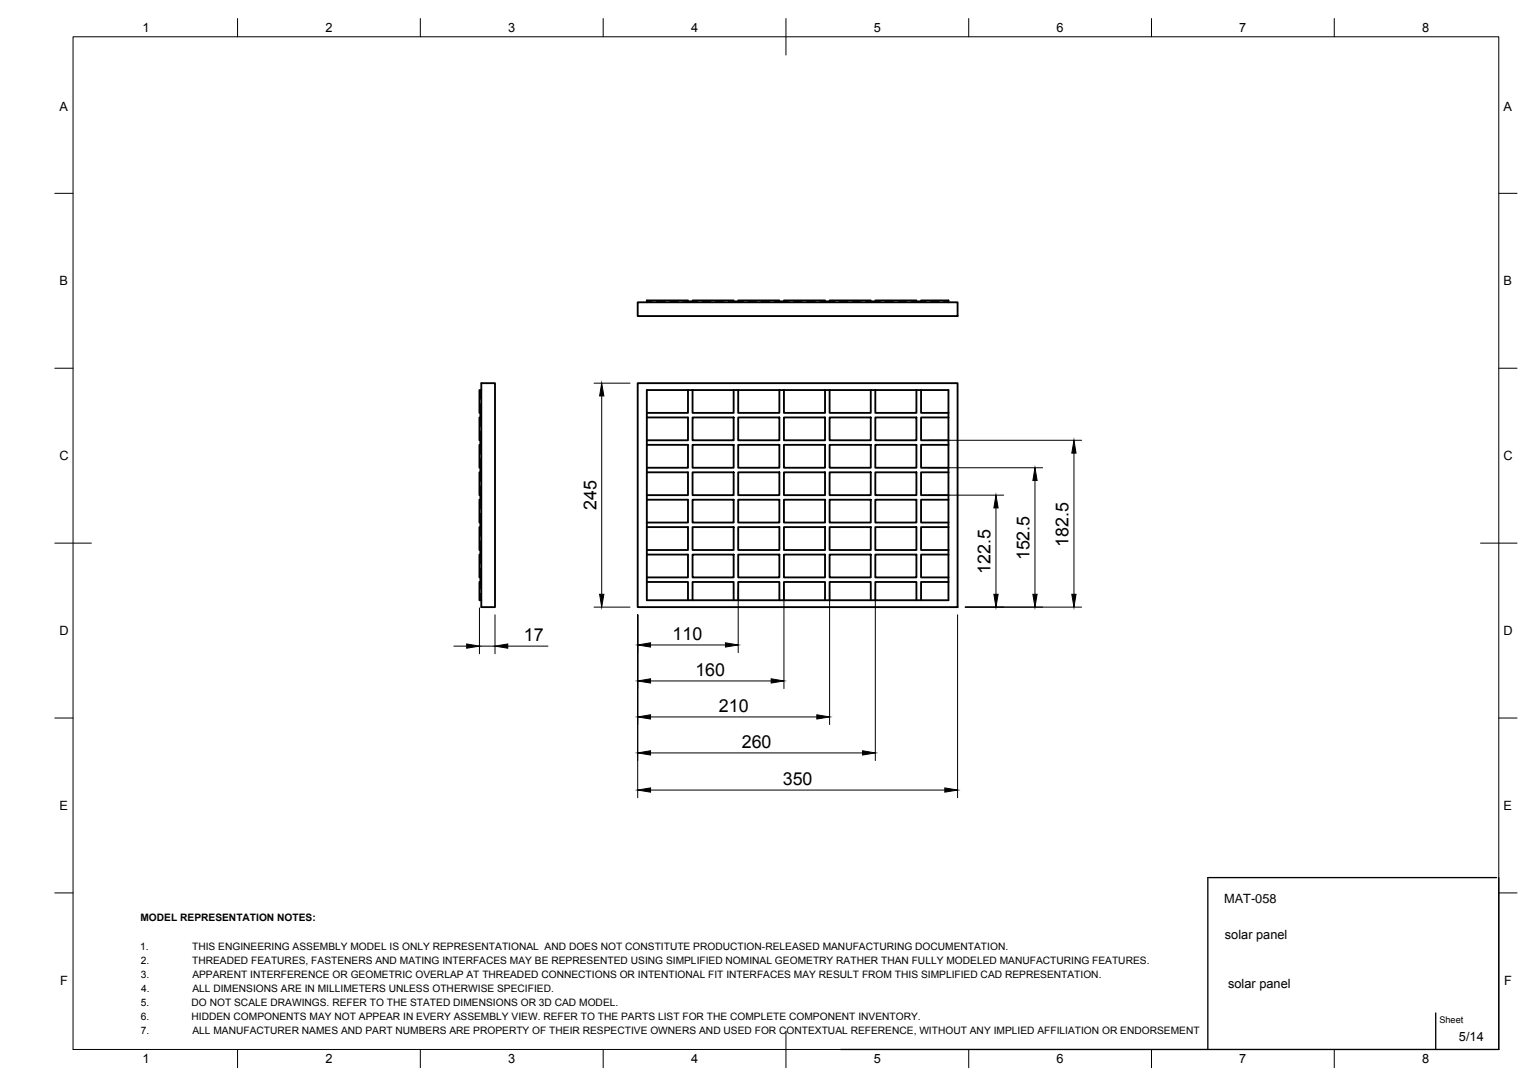
ISO-10303-21;
HEADER;
FILE_DESCRIPTION (('STEP AP214'),
    '1' );
FILE_NAME ('solar panel.step',
    '2026-10-21T17:54:40',
    ( '' ),
    ( '' ),
    'SwSTEP 2.0',
    'SolidWorks 2026',
    '' );
FILE_SCHEMA (( 'AUTOMOTIVE_DESIGN' ));
ENDSEC;

DATA;
#20=EDGE_CURVE ( 'NONE', #23493, #39659, #10554, .T. ) ;
#22=ORIENTED_EDGE ( 'NONE', *, *, #35505, .T. ) ;
#25=FACE_OUTER_BOUND ( 'NONE', #19071, .T. ) ;
#30=DIRECTION ( 'NONE',  ( 0.000000000000000000, 0.000000000000000000, 1.000000000000000000 ) ) ;
#34=AXIS2_PLACEMENT_3D ( 'NONE', #550, #47684, #4384 ) ;
#36=VERTEX_POINT ( 'NONE', #37038 ) ;
#46=ORIENTED_EDGE ( 'NONE', *, *, #39361, .F. ) ;
#51=CARTESIAN_POINT ( 'NONE',  ( -114.9999999999984652, 17.00000000000000000, 60.00000000000000000 ) ) ;
#57=LINE ( 'NONE', #42375, #32687 ) ;
#58=CARTESIAN_POINT ( 'NONE',  ( 130.0000000000021032, 17.00000000000000000, 95.00000000000000000 ) ) ;
#72=LINE ( 'NONE', #42385, #35392 ) ;
#73=EDGE_LOOP ( 'NONE', ( #24470, #20215, #48107, #6586 ) ) ;
#92=EDGE_CURVE ( 'NONE', #33627, #36736, #41611, .T. ) ;
#94=EDGE_CURVE ( 'NONE', #19596, #23363, #2597, .T. ) ;
#110=ORIENTED_EDGE ( 'NONE', *, *, #46921, .F. ) ;
#119=ORIENTED_EDGE ( 'NONE', *, *, #13290, .T. ) ;
#121=CARTESIAN_POINT ( 'NONE',  ( -114.9999999999978542, 17.00000000000000000, 95.00000000000000000 ) ) ;
#123=DIRECTION ( 'NONE',  ( -0.000000000000000000, -1.000000000000000000, -0.000000000000000000 ) ) ;
#125=CARTESIAN_POINT ( 'NONE',  ( -115.0000000000000284, 17.00000000000000000, -114.9999999999999858 ) ) ;
#133=ORIENTED_EDGE ( 'NONE', *, *, #48424, .F. ) ;
#137=FACE_OUTER_BOUND ( 'NONE', #38012, .T. ) ;
#140=VECTOR ( 'NONE', #20878, 1000.000000000000000 ) ;
#150=CARTESIAN_POINT ( 'NONE',  ( -14.99999999999876366, 17.00000000000000000, 30.00000000000000000 ) ) ;
#156=VERTEX_POINT ( 'NONE', #11065 ) ;
#162=LINE ( 'NONE', #15801, #49153 ) ;
#164=AXIS2_PLACEMENT_3D ( 'NONE', #11516, #32040, #11769 ) ;
#166=ORIENTED_EDGE ( 'NONE', *, *, #34974, .F. ) ;
#174=LINE ( 'NONE', #20666, #643 ) ;
#175=CARTESIAN_POINT ( 'NONE',  ( 30.00000000000062172, 17.00000000000000000, -54.99999999999999289 ) ) ;
#180=ADVANCED_FACE ( 'NONE', ( #12327 ), #40546, .F. ) ;
#186=ORIENTED_EDGE ( 'NONE', *, *, #38813, .T. ) ;
#193=EDGE_CURVE ( 'NONE', #28907, #37670, #20287, .T. ) ;
#196=VECTOR ( 'NONE', #29683, 1000.000000000000000 ) ;
#198=PLANE ( 'NONE',  #9790 ) ;
#221=ORIENTED_EDGE ( 'NONE', *, *, #30959, .F. ) ;
#224=ORIENTED_EDGE ( 'NONE', *, *, #7871, .F. ) ;
#230=PLANE ( 'NONE',  #20488 ) ;
#235=ADVANCED_FACE ( 'NONE', ( #32351 ), #40053, .F. ) ;
#243=DIRECTION ( 'NONE',  ( 1.000000000000000000, 0.000000000000000000, 0.000000000000000000 ) ) ;
#245=VECTOR ( 'NONE', #20305, 1000.000000000000000 ) ;
#246=EDGE_CURVE ( 'NONE', #20951, #20388, #31853, .T. ) ;
#251=DIRECTION ( 'NONE',  ( -1.000000000000000000, -0.000000000000000000, 9.251858538543084240E-16 ) ) ;
#264=EDGE_LOOP ( 'NONE', ( #43850, #6676, #18926, #28305 ) ) ;
#272=DIRECTION ( 'NONE',  ( 0.000000000000000000, 0.000000000000000000, 1.000000000000000000 ) ) ;
#277=VECTOR ( 'NONE', #22809, 1000.000000000000000 ) ;
#287=DIRECTION ( 'NONE',  ( -0.000000000000000000, -1.000000000000000000, -0.000000000000000000 ) ) ;
#302=VERTEX_POINT ( 'NONE', #41553 ) ;
#311=VECTOR ( 'NONE', #35432, 1000.000000000000000 ) ;
#313=EDGE_LOOP ( 'NONE', ( #26683, #2356, #8405, #20446 ) ) ;
#319=VECTOR ( 'NONE', #21069, 1000.000000000000000 ) ;
#321=ORIENTED_EDGE ( 'NONE', *, *, #26994, .T. ) ;
#325=VERTEX_POINT ( 'NONE', #9998 ) ;
#331=VECTOR ( 'NONE', #47511, 1000.000000000000000 ) ;
#338=EDGE_CURVE ( 'NONE', #17026, #45615, #13594, .T. ) ;
#343=VERTEX_POINT ( 'NONE', #22300 ) ;
#346=VECTOR ( 'NONE', #39780, 1000.000000000000000 ) ;
#364=FACE_OUTER_BOUND ( 'NONE', #38900, .T. ) ;
#375=VERTEX_POINT ( 'NONE', #32866 ) ;
#384=VECTOR ( 'NONE', #28524, 1000.000000000000000 ) ;
#389=DIRECTION ( 'NONE',  ( 0.000000000000000000, 0.000000000000000000, 1.000000000000000000 ) ) ;
#393=ORIENTED_EDGE ( 'NONE', *, *, #8336, .F. ) ;
#404=AXIS2_PLACEMENT_3D ( 'NONE', #20557, #28515, #1323 ) ;
#405=VERTEX_POINT ( 'NONE', #29501 ) ;
#409=DIRECTION ( 'NONE',  ( 1.000000000000000000, 0.000000000000000000, 0.000000000000000000 ) ) ;
#418=VERTEX_POINT ( 'NONE', #45117 ) ;
#437=ADVANCED_FACE ( 'NONE', ( #14088 ), #48694, .T. ) ;
#442=LINE ( 'NONE', #685, #41199 ) ;
#455=EDGE_LOOP ( 'NONE', ( #22398, #42737, #33219, #30241 ) ) ;
#465=ADVANCED_FACE ( 'NONE', ( #19658 ), #39933, .F. ) ;
#469=CARTESIAN_POINT ( 'NONE',  ( 135.0000000000015632, 17.00000000000000000, 35.00000000000000000 ) ) ;
#475=AXIS2_PLACEMENT_3D ( 'NONE', #19383, #34284, #35070 ) ;
#477=ORIENTED_EDGE ( 'NONE', *, *, #9884, .T. ) ;
#503=CARTESIAN_POINT ( 'NONE',  ( 35.00000000000186162, 17.00000000000000000, 90.00000000000000000 ) ) ;
#512=ORIENTED_EDGE ( 'NONE', *, *, #25092, .T. ) ;
#515=AXIS2_PLACEMENT_3D ( 'NONE', #26720, #30070, #30315 ) ;
#517=ORIENTED_EDGE ( 'NONE', *, *, #29930, .T. ) ;
#529=CARTESIAN_POINT ( 'NONE',  ( 130.0000000000008811, 17.00000000000000000, 0.000000000000000000 ) ) ;
#530=VECTOR ( 'NONE', #42052, 1000.000000000000000 ) ;
#540=CARTESIAN_POINT ( 'NONE',  ( 0.000000000000000000, 17.00000000000000000, 0.000000000000000000 ) ) ;
#550=CARTESIAN_POINT ( 'NONE',  ( -14.99999999999906919, 17.00000000000000000, 0.000000000000000000 ) ) ;
#553=ADVANCED_FACE ( 'NONE', ( #32726 ), #1435, .F. ) ;
#554=EDGE_LOOP ( 'NONE', ( #44360, #32925, #21521, #39510 ) ) ;
#562=FACE_OUTER_BOUND ( 'NONE', #36379, .T. ) ;
#570=FACE_OUTER_BOUND ( 'NONE', #16621, .T. ) ;
#572=VERTEX_POINT ( 'NONE', #13469 ) ;
#574=VERTEX_POINT ( 'NONE', #21414 ) ;
#593=VERTEX_POINT ( 'NONE', #47822 ) ;
#598=LINE ( 'NONE', #43663, #20030 ) ;
#608=ORIENTED_EDGE ( 'NONE', *, *, #26583, .T. ) ;
#614=VERTEX_POINT ( 'NONE', #44251 ) ;
#623=CARTESIAN_POINT ( 'NONE',  ( -19.99999999999971223, 16.00000000000000000, -84.99999999999998579 ) ) ;
#628=FACE_OUTER_BOUND ( 'NONE', #50651, .T. ) ;
#632=EDGE_LOOP ( 'NONE', ( #41784, #42230, #9108, #39526 ) ) ;
#643=VECTOR ( 'NONE', #47580, 1000.000000000000000 ) ;
#650=DIRECTION ( 'NONE',  ( -1.000000000000000000, 0.000000000000000000, -0.000000000000000000 ) ) ;
#651=ORIENTED_EDGE ( 'NONE', *, *, #30859, .F. ) ;
#654=ORIENTED_EDGE ( 'NONE', *, *, #31562, .T. ) ;
#659=ORIENTED_EDGE ( 'NONE', *, *, #38242, .F. ) ;
#674=CARTESIAN_POINT ( 'NONE',  ( -119.9999999999994174, 17.00000000000000000, -54.99999999999999289 ) ) ;
#680=CARTESIAN_POINT ( 'NONE',  ( 80.00000000000153477, 16.00000000000000000, 60.00000000000000000 ) ) ;
#681=CARTESIAN_POINT ( 'NONE',  ( 164.9999999999999716, 17.00000000000000000, -60.00000000000001421 ) ) ;
#685=CARTESIAN_POINT ( 'NONE',  ( 35.00000000000091660, 17.00000000000000000, -24.99999999999999289 ) ) ;
#690=LINE ( 'NONE', #30995, #5198 ) ;
#699=ORIENTED_EDGE ( 'NONE', *, *, #40875, .F. ) ;
#706=ORIENTED_EDGE ( 'NONE', *, *, #193, .T. ) ;
#709=CARTESIAN_POINT ( 'NONE',  ( -119.9999999999978400, 17.00000000000000000, 95.00000000000000000 ) ) ;
#717=FACE_OUTER_BOUND ( 'NONE', #38405, .T. ) ;
#726=EDGE_CURVE ( 'NONE', #3329, #34466, #14990, .T. ) ;
#732=CARTESIAN_POINT ( 'NONE',  ( -14.99999999999970868, 17.00000000000000000, -60.00000000000000000 ) ) ;
#740=EDGE_CURVE ( 'NONE', #30097, #19392, #10883, .T. ) ;
#752=VECTOR ( 'NONE', #24361, 1000.000000000000000 ) ;
#755=VECTOR ( 'NONE', #25642, 1000.000000000000000 ) ;
#766=EDGE_CURVE ( 'NONE', #31254, #1663, #37599, .T. ) ;
#768=ORIENTED_EDGE ( 'NONE', *, *, #15009, .T. ) ;
#774=ADVANCED_FACE ( 'NONE', ( #50080 ), #18072, .T. ) ;
#781=CARTESIAN_POINT ( 'NONE',  ( 135.0000000000021600, 16.00000000000000000, 95.00000000000000000 ) ) ;
#785=ORIENTED_EDGE ( 'NONE', *, *, #12346, .F. ) ;
#789=CARTESIAN_POINT ( 'NONE',  ( -19.99999999999940670, 17.00000000000000000, -30.00000000000000000 ) ) ;
#791=VECTOR ( 'NONE', #23137, 1000.000000000000000 ) ;
#794=EDGE_CURVE ( 'NONE', #35777, #38611, #10388, .T. ) ;
#798=VECTOR ( 'NONE', #15889, 1000.000000000000000 ) ;
#799=DIRECTION ( 'NONE',  ( 0.000000000000000000, -1.000000000000000000, 0.000000000000000000 ) ) ;
#802=EDGE_LOOP ( 'NONE', ( #19892, #43000, #16154, #21779 ) ) ;
#811=CARTESIAN_POINT ( 'NONE',  ( 35.00000000000186162, 16.00000000000000000, 65.00000000000000000 ) ) ;
#817=LINE ( 'NONE', #58, #1250 ) ;
#821=ORIENTED_EDGE ( 'NONE', *, *, #15184, .F. ) ;
#826=LINE ( 'NONE', #16475, #23214 ) ;
#839=CARTESIAN_POINT ( 'NONE',  ( 35.00000000000152767, 16.00000000000000000, 35.00000000000000000 ) ) ;
#844=CARTESIAN_POINT ( 'NONE',  ( -14.99999999999970868, 16.00000000000000000, -84.99999999999998579 ) ) ;
#845=VECTOR ( 'NONE', #3851, 1000.000000000000000 ) ;
#848=CARTESIAN_POINT ( 'NONE',  ( -164.9999999999990905, 17.00000000000000000, -24.99999999999999289 ) ) ;
#865=VERTEX_POINT ( 'NONE', #23456 ) ;
#867=AXIS2_PLACEMENT_3D ( 'NONE', #20688, #16848, #48346 ) ;
#871=LINE ( 'NONE', #16519, #9645 ) ;
#880=CARTESIAN_POINT ( 'NONE',  ( -19.99999999999815969, 16.00000000000000000, 65.00000000000000000 ) ) ;
#889=CARTESIAN_POINT ( 'NONE',  ( -64.99999999999940314, 17.00000000000000000, -54.99999999999999289 ) ) ;
#892=CARTESIAN_POINT ( 'NONE',  ( 85.00000000000184741, 17.00000000000000000, 65.00000000000000000 ) ) ;
#902=ORIENTED_EDGE ( 'NONE', *, *, #48896, .F. ) ;
#907=VERTEX_POINT ( 'NONE', #23706 ) ;
#908=ORIENTED_EDGE ( 'NONE', *, *, #17972, .T. ) ;
#919=LINE ( 'NONE', #40420, #42638 ) ;
#929=ORIENTED_EDGE ( 'NONE', *, *, #34476, .T. ) ;
#934=EDGE_CURVE ( 'NONE', #2472, #2811, #29066, .T. ) ;
#940=VECTOR ( 'NONE', #40898, 1000.000000000000000 ) ;
#941=ADVANCED_FACE ( 'NONE', ( #36028 ), #13159, .F. ) ;
#950=VERTEX_POINT ( 'NONE', #33187 ) ;
#970=VERTEX_POINT ( 'NONE', #24218 ) ;
#971=EDGE_CURVE ( 'NONE', #865, #3838, #17011, .T. ) ;
#978=ORIENTED_EDGE ( 'NONE', *, *, #12489, .T. ) ;
#981=LINE ( 'NONE', #28431, #46677 ) ;
#984=ORIENTED_EDGE ( 'NONE', *, *, #12101, .F. ) ;
#988=DIRECTION ( 'NONE',  ( 0.000000000000000000, 0.000000000000000000, -1.000000000000000000 ) ) ;
#997=CARTESIAN_POINT ( 'NONE',  ( -64.99999999999815259, 17.00000000000000000, 90.00000000000000000 ) ) ;
#1003=DIRECTION ( 'NONE',  ( -0.000000000000000000, -1.000000000000000000, -0.000000000000000000 ) ) ;
#1014=DIRECTION ( 'NONE',  ( 0.000000000000000000, 0.000000000000000000, -1.000000000000000000 ) ) ;
#1020=DIRECTION ( 'NONE',  ( -1.000000000000000000, -0.000000000000000000, -0.000000000000000000 ) ) ;
#1027=CARTESIAN_POINT ( 'NONE',  ( 85.00000000000056843, 17.00000000000000000, -30.00000000000000000 ) ) ;
#1034=EDGE_LOOP ( 'NONE', ( #26621, #37966, #49162, #17827 ) ) ;
#1035=CARTESIAN_POINT ( 'NONE',  ( -14.99999999999876366, 17.00000000000000000, 5.000000000000004441 ) ) ;
#1038=ORIENTED_EDGE ( 'NONE', *, *, #33245, .F. ) ;
#1046=DIRECTION ( 'NONE',  ( 0.000000000000000000, 0.000000000000000000, 1.000000000000000000 ) ) ;
#1057=DIRECTION ( 'NONE',  ( 0.000000000000000000, -0.000000000000000000, -1.000000000000000000 ) ) ;
#1067=ORIENTED_EDGE ( 'NONE', *, *, #11385, .F. ) ;
#1082=FACE_OUTER_BOUND ( 'NONE', #44486, .T. ) ;
#1090=EDGE_CURVE ( 'NONE', #32291, #24319, #41871, .T. ) ;
#1118=MECHANICAL_DESIGN_GEOMETRIC_PRESENTATION_REPRESENTATION('',(#6856),#35553);
#1147=VECTOR ( 'NONE', #17968, 1000.000000000000000 ) ;
#1148=EDGE_CURVE ( 'NONE', #30975, #45021, #10068, .T. ) ;
#1152=ORIENTED_EDGE ( 'NONE', *, *, #2044, .F. ) ;
#1162=PLANE ( 'NONE',  #7566 ) ;
#1174=VECTOR ( 'NONE', #42245, 1000.000000000000000 ) ;
#1181=ORIENTED_EDGE ( 'NONE', *, *, #33713, .F. ) ;
#1195=CARTESIAN_POINT ( 'NONE',  ( 35.00000000000122213, 17.00000000000000000, 5.000000000000004441 ) ) ;
#1202=DIRECTION ( 'NONE',  ( 0.000000000000000000, 0.000000000000000000, -1.000000000000000000 ) ) ;
#1204=AXIS2_PLACEMENT_3D ( 'NONE', #26739, #7748, #19015 ) ;
#1220=CARTESIAN_POINT ( 'NONE',  ( 35.00000000000091660, 16.00000000000000000, -24.99999999999999289 ) ) ;
#1236=EDGE_LOOP ( 'NONE', ( #22817, #30759, #48688, #4298 ) ) ;
#1245=LINE ( 'NONE', #9175, #17393 ) ;
#1247=FACE_OUTER_BOUND ( 'NONE', #4168, .T. ) ;
#1250=VECTOR ( 'NONE', #8517, 1000.000000000000000 ) ;
#1252=DIRECTION ( 'NONE',  ( -0.000000000000000000, -1.000000000000000000, -0.000000000000000000 ) ) ;
#1268=DIRECTION ( 'NONE',  ( 0.000000000000000000, 0.000000000000000000, 1.000000000000000000 ) ) ;
#1282=DIRECTION ( 'NONE',  ( -0.000000000000000000, -1.000000000000000000, -0.000000000000000000 ) ) ;
#1289=CARTESIAN_POINT ( 'NONE',  ( 80.00000000000061107, 17.00000000000000000, -54.99999999999999289 ) ) ;
#1292=EDGE_LOOP ( 'NONE', ( #10870, #27472, #30423, #39009 ) ) ;
#1293=ORIENTED_EDGE ( 'NONE', *, *, #18051, .F. ) ;
#1305=CARTESIAN_POINT ( 'NONE',  ( 30.00000000000123279, 17.00000000000000000, 5.000000000000004441 ) ) ;
#1319=DIRECTION ( 'NONE',  ( -1.000000000000000000, -0.000000000000000000, -0.000000000000000000 ) ) ;
#1323=DIRECTION ( 'NONE',  ( -1.000000000000000000, 0.000000000000000000, 2.312964634635843537E-16 ) ) ;
#1336=DIRECTION ( 'NONE',  ( -0.000000000000000000, -1.000000000000000000, -0.000000000000000000 ) ) ;
#1341=LINE ( 'NONE', #1837, #13601 ) ;
#1344=ORIENTED_EDGE ( 'NONE', *, *, #33713, .T. ) ;
#1348=CARTESIAN_POINT ( 'NONE',  ( -165.0000000000000284, 17.00000000000000000, -90.00000000000000000 ) ) ;
#1349=PLANE ( 'NONE',  #45547 ) ;
#1359=DIRECTION ( 'NONE',  ( 1.000000000000000000, 0.000000000000000000, 0.000000000000000000 ) ) ;
#1370=PLANE ( 'NONE',  #15035 ) ;
#1375=ORIENTED_EDGE ( 'NONE', *, *, #9884, .F. ) ;
#1384=DIRECTION ( 'NONE',  ( -0.000000000000000000, -0.000000000000000000, -1.000000000000000000 ) ) ;
#1386=ADVANCED_FACE ( 'NONE', ( #562 ), #28506, .F. ) ;
#1400=DIRECTION ( 'NONE',  ( 0.000000000000000000, 0.000000000000000000, 1.000000000000000000 ) ) ;
#1405=VERTEX_POINT ( 'NONE', #16688 ) ;
#1408=VECTOR ( 'NONE', #18293, 1000.000000000000000 ) ;
#1409=DIRECTION ( 'NONE',  ( 0.000000000000000000, 0.000000000000000000, 1.000000000000000000 ) ) ;
#1421=ORIENTED_EDGE ( 'NONE', *, *, #38820, .F. ) ;
#1424=AXIS2_PLACEMENT_3D ( 'NONE', #27930, #20227, #24090 ) ;
#1435=PLANE ( 'NONE',  #19680 ) ;
#1457=AXIS2_PLACEMENT_3D ( 'NONE', #19407, #34828, #31472 ) ;
#1471=DIRECTION ( 'NONE',  ( -2.312964634635864737E-16, 0.000000000000000000, -1.000000000000000000 ) ) ;
#1474=VERTEX_POINT ( 'NONE', #49462 ) ;
#1481=VERTEX_POINT ( 'NONE', #33623 ) ;
#1494=DIRECTION ( 'NONE',  ( 0.000000000000000000, 0.000000000000000000, 1.000000000000000000 ) ) ;
#1503=EDGE_CURVE ( 'NONE', #46696, #38550, #18450, .T. ) ;
#1526=LINE ( 'NONE', #32071, #45024 ) ;
#1528=VERTEX_POINT ( 'NONE', #48945 ) ;
#1535=ORIENTED_EDGE ( 'NONE', *, *, #37841, .F. ) ;
#1539=LINE ( 'NONE', #14076, #755 ) ;
#1549=CARTESIAN_POINT ( 'NONE',  ( 135.0000000000006253, 17.00000000000000000, -54.99999999999999289 ) ) ;
#1556=ORIENTED_EDGE ( 'NONE', *, *, #33956, .F. ) ;
#1578=ORIENTED_EDGE ( 'NONE', *, *, #38465, .F. ) ;
#1593=CARTESIAN_POINT ( 'NONE',  ( 135.0000000000015632, 17.00000000000000000, 35.00000000000000000 ) ) ;
#1597=CARTESIAN_POINT ( 'NONE',  ( -164.9999999999997442, 17.00000000000000000, -84.99999999999998579 ) ) ;
#1601=VECTOR ( 'NONE', #37906, 1000.000000000000000 ) ;
#1616=DIRECTION ( 'NONE',  ( 0.000000000000000000, 0.000000000000000000, 1.000000000000000000 ) ) ;
#1617=CARTESIAN_POINT ( 'NONE',  ( 129.9999999999999432, 17.00000000000000000, -114.9999999999999858 ) ) ;
#1626=DIRECTION ( 'NONE',  ( 1.000000000000000000, 0.000000000000000000, 0.000000000000000000 ) ) ;
#1628=LINE ( 'NONE', #17272, #16605 ) ;
#1653=CARTESIAN_POINT ( 'NONE',  ( 135.0000000000009663, 17.00000000000000000, -24.99999999999999289 ) ) ;
#1658=CARTESIAN_POINT ( 'NONE',  ( -64.99999999999815259, 16.00000000000000000, 90.00000000000000000 ) ) ;
#1663=VERTEX_POINT ( 'NONE', #31551 ) ;
#1669=VECTOR ( 'NONE', #37747, 1000.000000000000000 ) ;
#1683=CARTESIAN_POINT ( 'NONE',  ( -20.00000000000003197, 17.00000000000000000, -90.00000000000000000 ) ) ;
#1691=ADVANCED_FACE ( 'NONE', ( #22813 ), #15118, .F. ) ;
#1694=EDGE_CURVE ( 'NONE', #25157, #35762, #23369, .T. ) ;
#1697=ADVANCED_FACE ( 'NONE', ( #38733 ), #46388, .F. ) ;
#1701=DIRECTION ( 'NONE',  ( -0.000000000000000000, -1.000000000000000000, -0.000000000000000000 ) ) ;
#1707=AXIS2_PLACEMENT_3D ( 'NONE', #46684, #11062, #3101 ) ;
#1710=VECTOR ( 'NONE', #40010, 1000.000000000000000 ) ;
#1711=ORIENTED_EDGE ( 'NONE', *, *, #30976, .F. ) ;
#1718=ORIENTED_EDGE ( 'NONE', *, *, #38682, .T. ) ;
#1728=DIRECTION ( 'NONE',  ( 0.000000000000000000, 0.000000000000000000, 1.000000000000000000 ) ) ;
#1734=EDGE_CURVE ( 'NONE', #3452, #11387, #40498, .T. ) ;
#1743=VECTOR ( 'NONE', #7024, 1000.000000000000000 ) ;
#1751=CARTESIAN_POINT ( 'NONE',  ( 85.00000000000123634, 17.00000000000000000, 30.00000000000000000 ) ) ;
#1756=LINE ( 'NONE', #16389, #30760 ) ;
#1759=CARTESIAN_POINT ( 'NONE',  ( 135.0000000000009663, 16.00000000000000000, -24.99999999999999289 ) ) ;
#1770=EDGE_LOOP ( 'NONE', ( #6940, #12949, #39459, #6702 ) ) ;
#1775=EDGE_CURVE ( 'NONE', #28153, #21400, #32556, .T. ) ;
#1776=ORIENTED_EDGE ( 'NONE', *, *, #3846, .F. ) ;
#1778=CARTESIAN_POINT ( 'NONE',  ( 29.99999999999998579, 17.00000000000000000, -114.9999999999999858 ) ) ;
#1785=ORIENTED_EDGE ( 'NONE', *, *, #33974, .F. ) ;
#1788=ORIENTED_EDGE ( 'NONE', *, *, #23940, .F. ) ;
#1828=VECTOR ( 'NONE', #15724, 1000.000000000000000 ) ;
#1829=CARTESIAN_POINT ( 'NONE',  ( -114.9999999999991047, 16.00000000000000000, 0.000000000000000000 ) ) ;
#1834=DIRECTION ( 'NONE',  ( 0.000000000000000000, 0.000000000000000000, 1.000000000000000000 ) ) ;
#1837=CARTESIAN_POINT ( 'NONE',  ( -64.99999999999971578, 17.00000000000000000, -84.99999999999998579 ) ) ;
#1844=EDGE_CURVE ( 'NONE', #27666, #42474, #27940, .T. ) ;
#1866=DIRECTION ( 'NONE',  ( 1.000000000000000000, 0.000000000000000000, -0.000000000000000000 ) ) ;
#1867=FACE_OUTER_BOUND ( 'NONE', #40919, .T. ) ;
#1871=DIRECTION ( 'NONE',  ( 1.000000000000000000, 0.000000000000000000, 0.000000000000000000 ) ) ;
#1876=PLANE ( 'NONE',  #43014 ) ;
#1878=VERTEX_POINT ( 'NONE', #33812 ) ;
#1880=VECTOR ( 'NONE', #42551, 1000.000000000000000 ) ;
#1895=CARTESIAN_POINT ( 'NONE',  ( -114.9999999999994031, 17.00000000000000000, -30.00000000000000000 ) ) ;
#1900=ORIENTED_EDGE ( 'NONE', *, *, #7055, .T. ) ;
#1920=ORIENTED_EDGE ( 'NONE', *, *, #36078, .T. ) ;
#1929=ORIENTED_EDGE ( 'NONE', *, *, #31783, .F. ) ;
#1932=LINE ( 'NONE', #10389, #25219 ) ;
#1935=CARTESIAN_POINT ( 'NONE',  ( -64.99999999999877787, 16.00000000000000000, 5.000000000000004441 ) ) ;
#1936=EDGE_LOOP ( 'NONE', ( #15982, #1788, #659, #23682 ) ) ;
#1945=VECTOR ( 'NONE', #17455, 1000.000000000000000 ) ;
#1956=ORIENTED_EDGE ( 'NONE', *, *, #49060, .F. ) ;
#1964=DIRECTION ( 'NONE',  ( 1.000000000000000000, 0.000000000000000000, -2.312964634635864737E-16 ) ) ;
#1966=ORIENTED_EDGE ( 'NONE', *, *, #5485, .F. ) ;
#1968=CARTESIAN_POINT ( 'NONE',  ( 80.00000000000186162, 17.00000000000000000, 90.00000000000000000 ) ) ;
#1970=ORIENTED_EDGE ( 'NONE', *, *, #23753, .T. ) ;
#1972=AXIS2_PLACEMENT_3D ( 'NONE', #21850, #37515, #2333 ) ;
#1974=CARTESIAN_POINT ( 'NONE',  ( -114.9999999999997158, 17.00000000000000000, -60.00000000000000000 ) ) ;
#1976=EDGE_LOOP ( 'NONE', ( #15294, #42100, #49619, #25944 ) ) ;
#1983=EDGE_CURVE ( 'NONE', #7644, #20370, #41239, .T. ) ;
#1986=ADVANCED_FACE ( 'NONE', ( #25345 ), #40750, .F. ) ;
#2004=FACE_OUTER_BOUND ( 'NONE', #22418, .T. ) ;
#2005=EDGE_CURVE ( 'NONE', #47191, #2839, #26858, .T. ) ;
#2009=DIRECTION ( 'NONE',  ( 0.000000000000000000, 0.000000000000000000, 1.000000000000000000 ) ) ;
#2011=ORIENTED_EDGE ( 'NONE', *, *, #2047, .T. ) ;
#2014=CARTESIAN_POINT ( 'NONE',  ( -14.99999999999970868, 16.00000000000000000, -84.99999999999998579 ) ) ;
#2015=AXIS2_PLACEMENT_3D ( 'NONE', #44272, #17345, #9648 ) ;
#2023=CARTESIAN_POINT ( 'NONE',  ( -14.99999999999782041, 17.00000000000000000, 95.00000000000000000 ) ) ;
#2026=ORIENTED_EDGE ( 'NONE', *, *, #48076, .T. ) ;
#2041=ORIENTED_EDGE ( 'NONE', *, *, #38374, .F. ) ;
#2043=DIRECTION ( 'NONE',  ( -0.000000000000000000, -1.000000000000000000, -0.000000000000000000 ) ) ;
#2044=EDGE_CURVE ( 'NONE', #38025, #4851, #20418, .T. ) ;
#2047=EDGE_CURVE ( 'NONE', #35257, #35256, #8875, .T. ) ;
#2070=DIRECTION ( 'NONE',  ( 0.000000000000000000, 0.000000000000000000, -1.000000000000000000 ) ) ;
#2073=VECTOR ( 'NONE', #34325, 1000.000000000000000 ) ;
#2074=LINE ( 'NONE', #40570, #4337 ) ;
#2086=VERTEX_POINT ( 'NONE', #15819 ) ;
#2088=LINE ( 'NONE', #17475, #45768 ) ;
#2094=CARTESIAN_POINT ( 'NONE',  ( -19.99999999999878142, 16.00000000000000000, 5.000000000000004441 ) ) ;
#2096=ORIENTED_EDGE ( 'NONE', *, *, #29840, .F. ) ;
#2105=CARTESIAN_POINT ( 'NONE',  ( -19.99999999999783995, 17.00000000000000000, 95.00000000000000000 ) ) ;
#2108=CARTESIAN_POINT ( 'NONE',  ( 80.00000000000186162, 16.00000000000000000, 65.00000000000000000 ) ) ;
#2112=VECTOR ( 'NONE', #2639, 1000.000000000000000 ) ;
#2114=ORIENTED_EDGE ( 'NONE', *, *, #45262, .T. ) ;
#2118=EDGE_CURVE ( 'NONE', #35523, #46762, #44012, .T. ) ;
#2120=VECTOR ( 'NONE', #33876, 1000.000000000000000 ) ;
#2123=LINE ( 'NONE', #49009, #11921 ) ;
#2138=EDGE_CURVE ( 'NONE', #27259, #5809, #11372, .T. ) ;
#2139=VERTEX_POINT ( 'NONE', #50063 ) ;
#2156=ADVANCED_FACE ( 'NONE', ( #11635 ), #23175, .F. ) ;
#2172=FACE_OUTER_BOUND ( 'NONE', #36485, .T. ) ;
#2173=DIRECTION ( 'NONE',  ( -0.000000000000000000, -1.000000000000000000, -0.000000000000000000 ) ) ;
#2181=CARTESIAN_POINT ( 'NONE',  ( 135.0000000000021600, 16.00000000000000000, 115.0000000000000142 ) ) ;
#2183=ORIENTED_EDGE ( 'NONE', *, *, #7997, .F. ) ;
#2186=PLANE ( 'NONE',  #50543 ) ;
#2203=EDGE_CURVE ( 'NONE', #37192, #42338, #42157, .T. ) ;
#2210=DIRECTION ( 'NONE',  ( 0.000000000000000000, 0.000000000000000000, 1.000000000000000000 ) ) ;
#2212=VERTEX_POINT ( 'NONE', #27023 ) ;
#2256=EDGE_CURVE ( 'NONE', #44339, #18412, #42918, .T. ) ;
#2269=LINE ( 'NONE', #21775, #35286 ) ;
#2276=EDGE_CURVE ( 'NONE', #40766, #23064, #38342, .T. ) ;
#2277=PLANE ( 'NONE',  #41450 ) ;
#2278=ORIENTED_EDGE ( 'NONE', *, *, #5208, .F. ) ;
#2285=DIRECTION ( 'NONE',  ( -1.000000000000000000, -0.000000000000000000, -0.000000000000000000 ) ) ;
#2288=VERTEX_POINT ( 'NONE', #44899 ) ;
#2315=VECTOR ( 'NONE', #33438, 1000.000000000000000 ) ;
#2319=ORIENTED_EDGE ( 'NONE', *, *, #36924, .T. ) ;
#2324=VERTEX_POINT ( 'NONE', #13376 ) ;
#2329=DIRECTION ( 'NONE',  ( -0.000000000000000000, -0.000000000000000000, 1.000000000000000000 ) ) ;
#2330=LINE ( 'NONE', #17480, #1147 ) ;
#2333=DIRECTION ( 'NONE',  ( 0.000000000000000000, 0.000000000000000000, 1.000000000000000000 ) ) ;
#2335=ORIENTED_EDGE ( 'NONE', *, *, #44178, .F. ) ;
#2340=ADVANCED_FACE ( 'NONE', ( #45151 ), #6193, .F. ) ;
#2345=ORIENTED_EDGE ( 'NONE', *, *, #1694, .F. ) ;
#2348=PLANE ( 'NONE',  #18537 ) ;
#2356=ORIENTED_EDGE ( 'NONE', *, *, #31937, .F. ) ;
#2373=CARTESIAN_POINT ( 'NONE',  ( -114.9999999999981526, 17.00000000000000000, 65.00000000000000000 ) ) ;
#2374=ORIENTED_EDGE ( 'NONE', *, *, #30806, .F. ) ;
#2385=DIRECTION ( 'NONE',  ( 0.000000000000000000, 0.000000000000000000, 1.000000000000000000 ) ) ;
#2390=ORIENTED_EDGE ( 'NONE', *, *, #31295, .T. ) ;
#2404=LINE ( 'NONE', #6504, #16910 ) ;
#2405=CARTESIAN_POINT ( 'NONE',  ( 85.00000000000029843, 17.00000000000000000, -84.99999999999998579 ) ) ;
#2412=EDGE_CURVE ( 'NONE', #43496, #12984, #18225, .T. ) ;
#2415=ORIENTED_EDGE ( 'NONE', *, *, #42173, .F. ) ;
#2416=CARTESIAN_POINT ( 'NONE',  ( 85.00000000000029843, 16.00000000000000000, -84.99999999999998579 ) ) ;
#2417=LINE ( 'NONE', #37094, #7683 ) ;
#2422=VECTOR ( 'NONE', #2823, 1000.000000000000000 ) ;
#2425=PLANE ( 'NONE',  #10262 ) ;
#2428=EDGE_CURVE ( 'NONE', #26536, #46696, #22335, .T. ) ;
#2429=CARTESIAN_POINT ( 'NONE',  ( 35.00000000000216716, 16.00000000000000000, 115.0000000000000142 ) ) ;
#2443=VECTOR ( 'NONE', #28402, 1000.000000000000000 ) ;
#2444=LINE ( 'NONE', #29144, #11728 ) ;
#2450=LINE ( 'NONE', #29155, #45062 ) ;
#2452=CARTESIAN_POINT ( 'NONE',  ( -69.99999999999909051, 17.00000000000000000, 0.000000000000000000 ) ) ;
#2462=FACE_OUTER_BOUND ( 'NONE', #40549, .T. ) ;
#2472=VERTEX_POINT ( 'NONE', #37761 ) ;
#2483=EDGE_CURVE ( 'NONE', #43501, #26701, #32077, .T. ) ;
#2484=FACE_OUTER_BOUND ( 'NONE', #34875, .T. ) ;
#2500=ORIENTED_EDGE ( 'NONE', *, *, #41569, .F. ) ;
#2503=VECTOR ( 'NONE', #23758, 1000.000000000000000 ) ;
#2504=DIRECTION ( 'NONE',  ( -0.000000000000000000, -1.000000000000000000, -0.000000000000000000 ) ) ;
#2506=CARTESIAN_POINT ( 'NONE',  ( 164.9999999999999716, 17.00000000000000000, 59.99999999999999289 ) ) ;
#2507=VERTEX_POINT ( 'NONE', #24383 ) ;
#2513=CARTESIAN_POINT ( 'NONE',  ( -14.99999999999812594, 17.00000000000000000, 65.00000000000000000 ) ) ;
#2514=CARTESIAN_POINT ( 'NONE',  ( 34.99999999999997868, 17.00000000000000000, -90.00000000000000000 ) ) ;
#2516=LINE ( 'NONE', #17163, #37250 ) ;
#2517=ORIENTED_EDGE ( 'NONE', *, *, #44457, .F. ) ;
#2527=VERTEX_POINT ( 'NONE', #15916 ) ;
#2531=DIRECTION ( 'NONE',  ( -1.000000000000000000, -0.000000000000000000, -0.000000000000000000 ) ) ;
#2536=ORIENTED_EDGE ( 'NONE', *, *, #50341, .F. ) ;
#2544=FACE_BOUND ( 'NONE', #50410, .T. ) ;
#2547=CARTESIAN_POINT ( 'NONE',  ( -14.99999999999782041, 16.00000000000000000, 95.00000000000000000 ) ) ;
#2568=VECTOR ( 'NONE', #24294, 1000.000000000000000 ) ;
#2573=ORIENTED_EDGE ( 'NONE', *, *, #11718, .F. ) ;
#2575=CARTESIAN_POINT ( 'NONE',  ( 135.0000000000012790, 17.00000000000000000, 30.00000000000000000 ) ) ;
#2579=ORIENTED_EDGE ( 'NONE', *, *, #19259, .T. ) ;
#2580=EDGE_LOOP ( 'NONE', ( #21869, #13993, #23994, #18416 ) ) ;
#2582=ORIENTED_EDGE ( 'NONE', *, *, #14692, .T. ) ;
#2586=LINE ( 'NONE', #41347, #40139 ) ;
#2597=LINE ( 'NONE', #7737, #5617 ) ;
#2603=LINE ( 'NONE', #50203, #34893 ) ;
#2607=PLANE ( 'NONE',  #17875 ) ;
#2608=LINE ( 'NONE', #33933, #3718 ) ;
#2612=ORIENTED_EDGE ( 'NONE', *, *, #49052, .T. ) ;
#2636=CARTESIAN_POINT ( 'NONE',  ( -164.9999999999984936, 17.00000000000000000, 35.00000000000000000 ) ) ;
#2639=DIRECTION ( 'NONE',  ( 1.000000000000000000, 0.000000000000000000, 0.000000000000000000 ) ) ;
#2645=LINE ( 'NONE', #45212, #940 ) ;
#2663=FACE_OUTER_BOUND ( 'NONE', #13509, .T. ) ;
#2669=VECTOR ( 'NONE', #32314, 1000.000000000000000 ) ;
#2670=EDGE_CURVE ( 'NONE', #17128, #13622, #41268, .T. ) ;
#2675=LINE ( 'NONE', #33995, #41584 ) ;
#2677=VECTOR ( 'NONE', #42373, 1000.000000000000000 ) ;
#2689=DIRECTION ( 'NONE',  ( 0.000000000000000000, -1.000000000000000000, 0.000000000000000000 ) ) ;
#2691=ORIENTED_EDGE ( 'NONE', *, *, #7899, .F. ) ;
#2698=VECTOR ( 'NONE', #10503, 1000.000000000000000 ) ;
#2707=EDGE_LOOP ( 'NONE', ( #7508, #36482, #24854, #40175 ) ) ;
#2735=EDGE_LOOP ( 'NONE', ( #31824, #12828, #119, #35228 ) ) ;
#2747=VERTEX_POINT ( 'NONE', #25379 ) ;
#2753=CARTESIAN_POINT ( 'NONE',  ( -14.99999999999782041, 17.00000000000000000, 95.00000000000000000 ) ) ;
#2756=ADVANCED_FACE ( 'NONE', ( #39154 ), #45603, .F. ) ;
#2762=CARTESIAN_POINT ( 'NONE',  ( -19.99999999999846523, 17.00000000000000000, 60.00000000000000000 ) ) ;
#2768=VECTOR ( 'NONE', #30748, 1000.000000000000000 ) ;
#2791=CARTESIAN_POINT ( 'NONE',  ( -164.9999999999984936, 16.00000000000000000, 35.00000000000000000 ) ) ;
#2792=VECTOR ( 'NONE', #31544, 1000.000000000000000 ) ;
#2807=DIRECTION ( 'NONE',  ( 0.000000000000000000, -0.000000000000000000, -1.000000000000000000 ) ) ;
#2810=PLANE ( 'NONE',  #22180 ) ;
#2811=VERTEX_POINT ( 'NONE', #41527 ) ;
#2823=DIRECTION ( 'NONE',  ( -0.000000000000000000, -1.000000000000000000, -0.000000000000000000 ) ) ;
#2827=EDGE_CURVE ( 'NONE', #34035, #9083, #18668, .T. ) ;
#2833=LINE ( 'NONE', #11570, #18533 ) ;
#2839=VERTEX_POINT ( 'NONE', #10230 ) ;
#2848=EDGE_LOOP ( 'NONE', ( #12548, #50011, #24278, #41729 ) ) ;
#2849=EDGE_CURVE ( 'NONE', #36058, #16866, #34344, .T. ) ;
#2852=CARTESIAN_POINT ( 'NONE',  ( -114.9999999999994031, 17.00000000000000000, -54.99999999999999289 ) ) ;
#2853=DIRECTION ( 'NONE',  ( -1.000000000000000000, -0.000000000000000000, -0.000000000000000000 ) ) ;
#2868=ORIENTED_EDGE ( 'NONE', *, *, #35603, .F. ) ;
#2872=VECTOR ( 'NONE', #1252, 1000.000000000000000 ) ;
#2874=ORIENTED_EDGE ( 'NONE', *, *, #44978, .T. ) ;
#2877=LINE ( 'NONE', #14450, #7010 ) ;
#2884=ORIENTED_EDGE ( 'NONE', *, *, #5325, .T. ) ;
#2886=CARTESIAN_POINT ( 'NONE',  ( -64.99999999999877787, 17.00000000000000000, 30.00000000000000000 ) ) ;
#2908=EDGE_CURVE ( 'NONE', #22082, #37470, #14575, .T. ) ;
#2919=CARTESIAN_POINT ( 'NONE',  ( -14.99999999999845812, 17.00000000000000000, 35.00000000000000000 ) ) ;
#2934=ADVANCED_FACE ( 'NONE', ( #44477 ), #8850, .F. ) ;
#2941=DIRECTION ( 'NONE',  ( -1.000000000000000000, -0.000000000000000000, -0.000000000000000000 ) ) ;
#2951=AXIS2_PLACEMENT_3D ( 'NONE', #20075, #19309, #11624 ) ;
#2956=CARTESIAN_POINT ( 'NONE',  ( 85.00000000000090949, 17.00000000000000000, -24.99999999999999289 ) ) ;
#2959=ORIENTED_EDGE ( 'NONE', *, *, #42129, .T. ) ;
#2961=DIRECTION ( 'NONE',  ( -0.000000000000000000, -1.000000000000000000, -0.000000000000000000 ) ) ;
#2967=DIRECTION ( 'NONE',  ( -6.938893903907222461E-16, -0.000000000000000000, -1.000000000000000000 ) ) ;
#2976=ORIENTED_EDGE ( 'NONE', *, *, #28015, .T. ) ;
#2977=CARTESIAN_POINT ( 'NONE',  ( 0.000000000000000000, 17.00000000000000000, 0.000000000000000000 ) ) ;
#2978=CARTESIAN_POINT ( 'NONE',  ( -19.99999999999815969, 16.00000000000000000, 90.00000000000000000 ) ) ;
#2986=EDGE_LOOP ( 'NONE', ( #17759, #28658, #20389, #1956 ) ) ;
#2993=AXIS2_PLACEMENT_3D ( 'NONE', #43795, #24563, #24067 ) ;
#3004=EDGE_CURVE ( 'NONE', #20642, #23633, #49307, .T. ) ;
#3007=LINE ( 'NONE', #14304, #29645 ) ;
#3008=DIRECTION ( 'NONE',  ( 1.000000000000000000, 0.000000000000000000, -9.251858538543084240E-16 ) ) ;
#3009=LINE ( 'NONE', #18655, #2073 ) ;
#3010=ORIENTED_EDGE ( 'NONE', *, *, #11718, .T. ) ;
#3014=LINE ( 'NONE', #2762, #17264 ) ;
#3017=DIRECTION ( 'NONE',  ( -0.000000000000000000, -1.000000000000000000, -0.000000000000000000 ) ) ;
#3021=CARTESIAN_POINT ( 'NONE',  ( 135.0000000000003411, 17.00000000000000000, -84.99999999999998579 ) ) ;
#3040=CARTESIAN_POINT ( 'NONE',  ( -14.99999999999812594, 17.00000000000000000, 90.00000000000000000 ) ) ;
#3041=DIRECTION ( 'NONE',  ( 0.000000000000000000, -0.000000000000000000, -1.000000000000000000 ) ) ;
#3043=CARTESIAN_POINT ( 'NONE',  ( 35.00000000000122213, 17.00000000000000000, 30.00000000000000000 ) ) ;
#3044=CARTESIAN_POINT ( 'NONE',  ( -14.99999999999937472, 17.00000000000000000, -30.00000000000000000 ) ) ;
#3049=EDGE_CURVE ( 'NONE', #32394, #22969, #49558, .T. ) ;
#3052=EDGE_CURVE ( 'NONE', #43342, #34175, #49058, .T. ) ;
#3056=LINE ( 'NONE', #18700, #32288 ) ;
#3065=LINE ( 'NONE', #37994, #26446 ) ;
#3078=LINE ( 'NONE', #33899, #2422 ) ;
#3079=CARTESIAN_POINT ( 'NONE',  ( 80.00000000000028422, 17.00000000000000000, -60.00000000000000000 ) ) ;
#3086=VERTEX_POINT ( 'NONE', #29606 ) ;
#3093=EDGE_LOOP ( 'NONE', ( #8101, #18855, #13246, #36911 ) ) ;
#3096=DIRECTION ( 'NONE',  ( -1.000000000000000000, -0.000000000000000000, 4.625929269271635797E-16 ) ) ;
#3099=FACE_OUTER_BOUND ( 'NONE', #17848, .T. ) ;
#3101=DIRECTION ( 'NONE',  ( 0.000000000000000000, 0.000000000000000000, 1.000000000000000000 ) ) ;
#3102=CARTESIAN_POINT ( 'NONE',  ( -114.9999999999991047, 17.00000000000000000, -24.99999999999999289 ) ) ;
#3106=CARTESIAN_POINT ( 'NONE',  ( 30.00000000000187228, 17.00000000000000000, 65.00000000000000000 ) ) ;
#3115=AXIS2_PLACEMENT_3D ( 'NONE', #37666, #37173, #45809 ) ;
#3116=CARTESIAN_POINT ( 'NONE',  ( 35.00000000000028422, 17.00000000000000000, -84.99999999999998579 ) ) ;
#3118=CARTESIAN_POINT ( 'NONE',  ( -19.99999999999878142, 17.00000000000000000, 5.000000000000004441 ) ) ;
#3129=LINE ( 'NONE', #31107, #42142 ) ;
#3130=LINE ( 'NONE', #43162, #23045 ) ;
#3131=ORIENTED_EDGE ( 'NONE', *, *, #37323, .T. ) ;
#3138=ORIENTED_EDGE ( 'NONE', *, *, #22162, .F. ) ;
#3141=ADVANCED_FACE ( 'NONE', ( #21916 ), #37583, .F. ) ;
#3142=VECTOR ( 'NONE', #25991, 1000.000000000000000 ) ;
#3149=ORIENTED_EDGE ( 'NONE', *, *, #42550, .T. ) ;
#3154=LINE ( 'NONE', #18300, #28798 ) ;
#3159=CARTESIAN_POINT ( 'NONE',  ( 85.00000000000123634, 17.00000000000000000, 5.000000000000004441 ) ) ;
#3166=ORIENTED_EDGE ( 'NONE', *, *, #19090, .F. ) ;
#3175=DIRECTION ( 'NONE',  ( 1.000000000000000000, 0.000000000000000000, 0.000000000000000000 ) ) ;
#3176=CARTESIAN_POINT ( 'NONE',  ( -20.00000000000003197, 16.00000000000000000, -114.9999999999999858 ) ) ;
#3181=CARTESIAN_POINT ( 'NONE',  ( 135.0000000000006253, 16.00000000000000000, -54.99999999999999289 ) ) ;
#3182=VECTOR ( 'NONE', #6227, 1000.000000000000000 ) ;
#3183=PLANE ( 'NONE',  #12279 ) ;
#3194=EDGE_CURVE ( 'NONE', #17776, #34175, #42153, .T. ) ;
#3198=ORIENTED_EDGE ( 'NONE', *, *, #37933, .T. ) ;
#3202=CARTESIAN_POINT ( 'NONE',  ( -69.99999999999816680, 17.00000000000000000, 65.00000000000000000 ) ) ;
#3216=VERTEX_POINT ( 'NONE', #38337 ) ;
#3221=CARTESIAN_POINT ( 'NONE',  ( 35.00000000000061107, 16.00000000000000000, -30.00000000000000000 ) ) ;
#3229=CARTESIAN_POINT ( 'NONE',  ( -14.99999999999812594, 17.00000000000000000, 90.00000000000000000 ) ) ;
#3233=DIRECTION ( 'NONE',  ( 0.000000000000000000, -0.000000000000000000, -1.000000000000000000 ) ) ;
#3236=CARTESIAN_POINT ( 'NONE',  ( -64.99999999999971578, 16.00000000000000000, -60.00000000000000000 ) ) ;
#3250=VECTOR ( 'NONE', #31432, 1000.000000000000000 ) ;
#3256=VECTOR ( 'NONE', #17185, 1000.000000000000000 ) ;
#3258=VERTEX_POINT ( 'NONE', #26772 ) ;
#3275=ORIENTED_EDGE ( 'NONE', *, *, #12788, .F. ) ;
#3279=EDGE_LOOP ( 'NONE', ( #36139, #43467, #26596, #6835 ) ) ;
#3284=VERTEX_POINT ( 'NONE', #26515 ) ;
#3287=ORIENTED_EDGE ( 'NONE', *, *, #49621, .T. ) ;
#3297=EDGE_CURVE ( 'NONE', #20901, #15399, #36008, .T. ) ;
#3306=DIRECTION ( 'NONE',  ( -0.000000000000000000, -1.000000000000000000, -0.000000000000000000 ) ) ;
#3317=LINE ( 'NONE', #31048, #25609 ) ;
#3323=LINE ( 'NONE', #30801, #43763 ) ;
#3327=VECTOR ( 'NONE', #48289, 1000.000000000000000 ) ;
#3329=VERTEX_POINT ( 'NONE', #4930 ) ;
#3331=CARTESIAN_POINT ( 'NONE',  ( 30.00000000000092726, 17.00000000000000000, -24.99999999999999289 ) ) ;
#3339=AXIS2_PLACEMENT_3D ( 'NONE', #47286, #19860, #30933 ) ;
#3348=ORIENTED_EDGE ( 'NONE', *, *, #27379, .T. ) ;
#3349=DIRECTION ( 'NONE',  ( 0.000000000000000000, 0.000000000000000000, -1.000000000000000000 ) ) ;
#3355=LINE ( 'NONE', #41858, #30385 ) ;
#3361=ORIENTED_EDGE ( 'NONE', *, *, #20811, .T. ) ;
#3381=DIRECTION ( 'NONE',  ( -0.000000000000000000, -0.000000000000000000, -1.000000000000000000 ) ) ;
#3388=EDGE_CURVE ( 'NONE', #36127, #23493, #27543, .T. ) ;
#3389=DIRECTION ( 'NONE',  ( -1.000000000000000000, -0.000000000000000000, -0.000000000000000000 ) ) ;
#3395=VERTEX_POINT ( 'NONE', #23681 ) ;
#3404=VECTOR ( 'NONE', #1319, 1000.000000000000000 ) ;
#3409=DIRECTION ( 'NONE',  ( 0.000000000000000000, 0.000000000000000000, 1.000000000000000000 ) ) ;
#3412=DIRECTION ( 'NONE',  ( -0.000000000000000000, -0.000000000000000000, -1.000000000000000000 ) ) ;
#3413=AXIS2_PLACEMENT_3D ( 'NONE', #19158, #15338, #35105 ) ;
#3426=ORIENTED_EDGE ( 'NONE', *, *, #40442, .T. ) ;
#3438=VECTOR ( 'NONE', #42191, 1000.000000000000000 ) ;
#3442=LINE ( 'NONE', #3181, #34377 ) ;
#3452=VERTEX_POINT ( 'NONE', #25702 ) ;
#3453=CARTESIAN_POINT ( 'NONE',  ( -175.0000000000000000, 15.00000000000000000, 122.5000000000000142 ) ) ;
#3463=EDGE_CURVE ( 'NONE', #11684, #2139, #29297, .T. ) ;
#3465=ORIENTED_EDGE ( 'NONE', *, *, #7771, .T. ) ;
#3468=CARTESIAN_POINT ( 'NONE',  ( 85.00000000000152056, 17.00000000000000000, 35.00000000000000000 ) ) ;
#3474=ORIENTED_EDGE ( 'NONE', *, *, #22858, .F. ) ;
#3478=PLANE ( 'NONE',  #25794 ) ;
#3481=CARTESIAN_POINT ( 'NONE',  ( 129.9999999999999432, 16.00000000000000000, -90.00000000000000000 ) ) ;
#3487=VECTOR ( 'NONE', #47496, 1000.000000000000000 ) ;
#3499=ORIENTED_EDGE ( 'NONE', *, *, #25092, .F. ) ;
#3502=DIRECTION ( 'NONE',  ( 0.000000000000000000, 0.000000000000000000, 1.000000000000000000 ) ) ;
#3505=DIRECTION ( 'NONE',  ( -1.000000000000000000, 0.000000000000000000, -0.000000000000000000 ) ) ;
#3506=DIRECTION ( 'NONE',  ( -0.000000000000000000, -1.000000000000000000, -0.000000000000000000 ) ) ;
#3517=CARTESIAN_POINT ( 'NONE',  ( -65.00000000000002842, 17.00000000000000000, -114.9999999999999858 ) ) ;
#3529=CARTESIAN_POINT ( 'NONE',  ( 0.000000000000000000, 17.00000000000000000, 0.000000000000000000 ) ) ;
#3534=CARTESIAN_POINT ( 'NONE',  ( 85.00000000000213163, 17.00000000000000000, 115.0000000000000142 ) ) ;
#3550=CARTESIAN_POINT ( 'NONE',  ( -15.00000000000001421, 17.00000000000000000, -114.9999999999999858 ) ) ;
#3563=ORIENTED_EDGE ( 'NONE', *, *, #11111, .F. ) ;
#3569=DIRECTION ( 'NONE',  ( -0.000000000000000000, -1.000000000000000000, -0.000000000000000000 ) ) ;
#3576=DIRECTION ( 'NONE',  ( 0.000000000000000000, 0.000000000000000000, 1.000000000000000000 ) ) ;
#3599=CARTESIAN_POINT ( 'NONE',  ( 30.00000000000092726, 17.00000000000000000, 0.000000000000000000 ) ) ;
#3606=CARTESIAN_POINT ( 'NONE',  ( 85.00000000000090949, 17.00000000000000000, -24.99999999999999289 ) ) ;
#3607=EDGE_LOOP ( 'NONE', ( #34537, #18552, #35865, #36207 ) ) ;
#3610=CARTESIAN_POINT ( 'NONE',  ( 0.000000000000000000, 17.00000000000000000, 0.000000000000000000 ) ) ;
#3611=DIRECTION ( 'NONE',  ( 0.000000000000000000, 0.000000000000000000, 1.000000000000000000 ) ) ;
#3613=VECTOR ( 'NONE', #42083, 1000.000000000000000 ) ;
#3614=ORIENTED_EDGE ( 'NONE', *, *, #6119, .F. ) ;
#3616=EDGE_CURVE ( 'NONE', #39284, #48491, #15415, .T. ) ;
#3619=VECTOR ( 'NONE', #26495, 1000.000000000000000 ) ;
#3630=DIRECTION ( 'NONE',  ( -0.000000000000000000, -1.000000000000000000, -0.000000000000000000 ) ) ;
#3634=DIRECTION ( 'NONE',  ( 0.000000000000000000, 0.000000000000000000, 1.000000000000000000 ) ) ;
#3673=CARTESIAN_POINT ( 'NONE',  ( 130.0000000000021032, 16.00000000000000000, 95.00000000000000000 ) ) ;
#3674=ORIENTED_EDGE ( 'NONE', *, *, #36613, .T. ) ;
#3680=CARTESIAN_POINT ( 'NONE',  ( -65.00000000000002842, 16.00000000000000000, -90.00000000000000000 ) ) ;
#3683=CARTESIAN_POINT ( 'NONE',  ( -65.00000000000002842, 16.00000000000000000, -90.00000000000000000 ) ) ;
#3693=VECTOR ( 'NONE', #4074, 1000.000000000000000 ) ;
#3703=AXIS2_PLACEMENT_3D ( 'NONE', #32046, #36923, #37171 ) ;
#3705=ADVANCED_FACE ( 'NONE', ( #44107 ), #35442, .F. ) ;
#3709=LINE ( 'NONE', #27584, #4912 ) ;
#3711=CARTESIAN_POINT ( 'NONE',  ( 164.9999999999999716, 16.00000000000000000, 65.00000000000000000 ) ) ;
#3713=VECTOR ( 'NONE', #5926, 1000.000000000000000 ) ;
#3718=VECTOR ( 'NONE', #10070, 1000.000000000000000 ) ;
#3719=VERTEX_POINT ( 'NONE', #16670 ) ;
#3720=ORIENTED_EDGE ( 'NONE', *, *, #43078, .T. ) ;
#3730=AXIS2_PLACEMENT_3D ( 'NONE', #26082, #13766, #6585 ) ;
#3739=LINE ( 'NONE', #38651, #3861 ) ;
#3742=ORIENTED_EDGE ( 'NONE', *, *, #12633, .T. ) ;
#3746=CARTESIAN_POINT ( 'NONE',  ( -69.99999999999940314, 17.00000000000000000, -54.99999999999999289 ) ) ;
#3766=AXIS2_PLACEMENT_3D ( 'NONE', #45100, #37960, #14581 ) ;
#3772=DIRECTION ( 'NONE',  ( -0.000000000000000000, -1.000000000000000000, -0.000000000000000000 ) ) ;
#3780=CARTESIAN_POINT ( 'NONE',  ( 164.9999999999999716, 15.00000000000000000, 115.0000000000000142 ) ) ;
#3789=VERTEX_POINT ( 'NONE', #47934 ) ;
#3791=LINE ( 'NONE', #4307, #46173 ) ;
#3796=DIRECTION ( 'NONE',  ( 1.000000000000000000, 0.000000000000000000, 0.000000000000000000 ) ) ;
#3798=CARTESIAN_POINT ( 'NONE',  ( -69.99999999999940314, 16.00000000000000000, -30.00000000000000000 ) ) ;
#3803=VERTEX_POINT ( 'NONE', #35187 ) ;
#3806=ORIENTED_EDGE ( 'NONE', *, *, #8825, .F. ) ;
#3807=DIRECTION ( 'NONE',  ( -0.000000000000000000, -1.000000000000000000, -0.000000000000000000 ) ) ;
#3813=PLANE ( 'NONE',  #25568 ) ;
#3819=DIRECTION ( 'NONE',  ( 0.000000000000000000, 0.000000000000000000, -1.000000000000000000 ) ) ;
#3820=CARTESIAN_POINT ( 'NONE',  ( 35.00000000000216716, 17.00000000000000000, 115.0000000000000142 ) ) ;
#3838=VERTEX_POINT ( 'NONE', #20277 ) ;
#3841=EDGE_CURVE ( 'NONE', #7468, #41411, #35946, .T. ) ;
#3846=EDGE_CURVE ( 'NONE', #9471, #7228, #32084, .T. ) ;
#3847=AXIS2_PLACEMENT_3D ( 'NONE', #42030, #21520, #29478 ) ;
#3851=DIRECTION ( 'NONE',  ( -0.000000000000000000, -0.000000000000000000, -1.000000000000000000 ) ) ;
#3852=DIRECTION ( 'NONE',  ( -0.000000000000000000, -1.000000000000000000, -0.000000000000000000 ) ) ;
#3861=VECTOR ( 'NONE', #34813, 1000.000000000000000 ) ;
#3863=CARTESIAN_POINT ( 'NONE',  ( -165.0000000000000284, 16.00000000000000000, -114.9999999999999858 ) ) ;
#3867=EDGE_LOOP ( 'NONE', ( #9418, #36728, #42468, #12485 ) ) ;
#3884=FACE_OUTER_BOUND ( 'NONE', #39698, .T. ) ;
#3888=EDGE_CURVE ( 'NONE', #34035, #31951, #9225, .T. ) ;
#3914=EDGE_LOOP ( 'NONE', ( #27318, #30038, #31505, #40737 ) ) ;
#3916=EDGE_CURVE ( 'NONE', #9256, #30177, #1539, .T. ) ;
#3921=DIRECTION ( 'NONE',  ( 1.000000000000000000, 0.000000000000000000, 0.000000000000000000 ) ) ;
#3926=EDGE_CURVE ( 'NONE', #34772, #8207, #5879, .T. ) ;
#3927=ORIENTED_EDGE ( 'NONE', *, *, #35284, .T. ) ;
#3934=ORIENTED_EDGE ( 'NONE', *, *, #21121, .F. ) ;
#3936=CARTESIAN_POINT ( 'NONE',  ( -114.9999999999987779, 17.00000000000000000, 30.00000000000000000 ) ) ;
#3940=ORIENTED_EDGE ( 'NONE', *, *, #44807, .T. ) ;
#3943=ORIENTED_EDGE ( 'NONE', *, *, #12300, .F. ) ;
#3955=FACE_OUTER_BOUND ( 'NONE', #41248, .T. ) ;
#3964=AXIS2_PLACEMENT_3D ( 'NONE', #5219, #16771, #9076 ) ;
#3965=LINE ( 'NONE', #30155, #23785 ) ;
#3969=ORIENTED_EDGE ( 'NONE', *, *, #971, .F. ) ;
#3982=CARTESIAN_POINT ( 'NONE',  ( 35.00000000000091660, 16.00000000000000000, -24.99999999999999289 ) ) ;
#3984=ORIENTED_EDGE ( 'NONE', *, *, #46187, .T. ) ;
#3988=CARTESIAN_POINT ( 'NONE',  ( -69.99999999999972999, 17.00000000000000000, -60.00000000000000000 ) ) ;
#3998=LINE ( 'NONE', #42476, #48834 ) ;
#4019=VECTOR ( 'NONE', #18189, 1000.000000000000000 ) ;
#4023=ORIENTED_EDGE ( 'NONE', *, *, #7311, .T. ) ;
#4024=PLANE ( 'NONE',  #33528 ) ;
#4037=ORIENTED_EDGE ( 'NONE', *, *, #26822, .T. ) ;
#4044=EDGE_CURVE ( 'NONE', #49920, #14126, #34109, .T. ) ;
#4047=LINE ( 'NONE', #8159, #24117 ) ;
#4053=ADVANCED_FACE ( 'NONE', ( #25900 ), #26390, .F. ) ;
#4063=ORIENTED_EDGE ( 'NONE', *, *, #33730, .T. ) ;
#4064=DIRECTION ( 'NONE',  ( 1.000000000000000000, 0.000000000000000000, 0.000000000000000000 ) ) ;
#4069=DIRECTION ( 'NONE',  ( -1.000000000000000000, -0.000000000000000000, -0.000000000000000000 ) ) ;
#4074=DIRECTION ( 'NONE',  ( 1.000000000000000000, 0.000000000000000000, 0.000000000000000000 ) ) ;
#4077=FACE_OUTER_BOUND ( 'NONE', #33283, .T. ) ;
#4080=VECTOR ( 'NONE', #6104, 1000.000000000000000 ) ;
#4088=VECTOR ( 'NONE', #48245, 1000.000000000000000 ) ;
#4091=LINE ( 'NONE', #39506, #752 ) ;
#4092=CARTESIAN_POINT ( 'NONE',  ( -114.9999999999984652, 17.00000000000000000, 35.00000000000000000 ) ) ;
#4093=CARTESIAN_POINT ( 'NONE',  ( -164.9999999999997442, 17.00000000000000000, -60.00000000000000000 ) ) ;
#4095=VECTOR ( 'NONE', #23354, 1000.000000000000000 ) ;
#4098=ORIENTED_EDGE ( 'NONE', *, *, #11415, .F. ) ;
#4101=FACE_OUTER_BOUND ( 'NONE', #10309, .T. ) ;
#4105=ORIENTED_EDGE ( 'NONE', *, *, #28088, .T. ) ;
#4107=CARTESIAN_POINT ( 'NONE',  ( 29.99999999999998579, 17.00000000000000000, -90.00000000000000000 ) ) ;
#4114=CARTESIAN_POINT ( 'NONE',  ( -165.0000000000000284, 16.00000000000000000, 115.0000000000000142 ) ) ;
#4130=CARTESIAN_POINT ( 'NONE',  ( 135.0000000000003411, 16.00000000000000000, -60.00000000000000000 ) ) ;
#4140=PLANE ( 'NONE',  #24805 ) ;
#4142=EDGE_LOOP ( 'NONE', ( #9671, #14688, #699, #4511 ) ) ;
#4146=PLANE ( 'NONE',  #39828 ) ;
#4164=AXIS2_PLACEMENT_3D ( 'NONE', #38541, #22611, #3611 ) ;
#4165=VECTOR ( 'NONE', #10960, 1000.000000000000000 ) ;
#4167=CARTESIAN_POINT ( 'NONE',  ( 135.0000000000012790, 17.00000000000000000, 5.000000000000004441 ) ) ;
#4168=EDGE_LOOP ( 'NONE', ( #34605, #11609, #27626, #32368 ) ) ;
#4173=DIRECTION ( 'NONE',  ( 0.000000000000000000, -1.000000000000000000, 0.000000000000000000 ) ) ;
#4183=DIRECTION ( 'NONE',  ( 0.000000000000000000, 0.000000000000000000, 1.000000000000000000 ) ) ;
#4187=ORIENTED_EDGE ( 'NONE', *, *, #21739, .T. ) ;
#4191=VECTOR ( 'NONE', #46469, 1000.000000000000000 ) ;
#4197=CARTESIAN_POINT ( 'NONE',  ( -114.9999999999994031, 17.00000000000000000, -30.00000000000000000 ) ) ;
#4198=PLANE ( 'NONE',  #5409 ) ;
#4199=VECTOR ( 'NONE', #7271, 1000.000000000000000 ) ;
#4202=PRODUCT_DEFINITION_CONTEXT ( 'detailed design', #39776, 'design' ) ;
#4205=VECTOR ( 'NONE', #1202, 1000.000000000000000 ) ;
#4207=CARTESIAN_POINT ( 'NONE',  ( 35.00000000000152767, 16.00000000000000000, 35.00000000000000000 ) ) ;
#4208=EDGE_LOOP ( 'NONE', ( #18998, #37444, #48111, #24651 ) ) ;
#4218=DIRECTION ( 'NONE',  ( 0.000000000000000000, -0.000000000000000000, -1.000000000000000000 ) ) ;
#4222=EDGE_CURVE ( 'NONE', #593, #23700, #23817, .T. ) ;
#4224=DIRECTION ( 'NONE',  ( -0.000000000000000000, -1.000000000000000000, -0.000000000000000000 ) ) ;
#4235=CARTESIAN_POINT ( 'NONE',  ( 35.00000000000216716, 16.00000000000000000, 95.00000000000000000 ) ) ;
#4255=DIRECTION ( 'NONE',  ( -0.000000000000000000, -1.000000000000000000, -0.000000000000000000 ) ) ;
#4262=ORIENTED_EDGE ( 'NONE', *, *, #19250, .F. ) ;
#4263=VERTEX_POINT ( 'NONE', #1974 ) ;
#4265=CARTESIAN_POINT ( 'NONE',  ( -69.99999999999940314, 17.00000000000000000, -30.00000000000000000 ) ) ;
#4270=CARTESIAN_POINT ( 'NONE',  ( -164.9999999999997442, 17.00000000000000000, -60.00000000000000000 ) ) ;
#4298=ORIENTED_EDGE ( 'NONE', *, *, #23675, .T. ) ;
#4305=VECTOR ( 'NONE', #10915, 1000.000000000000000 ) ;
#4307=CARTESIAN_POINT ( 'NONE',  ( -64.99999999999877787, 17.00000000000000000, 5.000000000000004441 ) ) ;
#4309=DIRECTION ( 'NONE',  ( 0.000000000000000000, 0.000000000000000000, 1.000000000000000000 ) ) ;
#4317=CARTESIAN_POINT ( 'NONE',  ( -64.99999999999846523, 16.00000000000000000, 35.00000000000000000 ) ) ;
#4326=PLANE ( 'NONE',  #4920 ) ;
#4335=LINE ( 'NONE', #3820, #11721 ) ;
#4337=VECTOR ( 'NONE', #17722, 1000.000000000000000 ) ;
#4340=EDGE_CURVE ( 'NONE', #39670, #46399, #48119, .T. ) ;
#4345=DIRECTION ( 'NONE',  ( 1.000000000000000000, 0.000000000000000000, 0.000000000000000000 ) ) ;
#4352=VERTEX_POINT ( 'NONE', #18364 ) ;
#4356=EDGE_LOOP ( 'NONE', ( #33297, #34547, #24964, #35461 ) ) ;
#4377=CARTESIAN_POINT ( 'NONE',  ( -15.00000000000001421, 17.00000000000000000, -90.00000000000000000 ) ) ;
#4378=CARTESIAN_POINT ( 'NONE',  ( -64.99999999999846523, 16.00000000000000000, 35.00000000000000000 ) ) ;
#4381=EDGE_CURVE ( 'NONE', #37527, #20642, #38155, .T. ) ;
#4383=CARTESIAN_POINT ( 'NONE',  ( -165.0000000000000284, 16.00000000000000000, 115.0000000000000142 ) ) ;
#4384=DIRECTION ( 'NONE',  ( -1.000000000000000000, 0.000000000000000000, -0.000000000000000000 ) ) ;
#4389=DIRECTION ( 'NONE',  ( 4.625929269271635797E-16, -0.000000000000000000, 1.000000000000000000 ) ) ;
#4391=ORIENTED_EDGE ( 'NONE', *, *, #6692, .F. ) ;
#4392=VERTEX_POINT ( 'NONE', #34546 ) ;
#4400=DIRECTION ( 'NONE',  ( -0.000000000000000000, -0.000000000000000000, -1.000000000000000000 ) ) ;
#4402=PLANE ( 'NONE',  #40097 ) ;
#4407=ORIENTED_EDGE ( 'NONE', *, *, #29641, .T. ) ;
#4409=ORIENTED_EDGE ( 'NONE', *, *, #3297, .F. ) ;
#4410=CARTESIAN_POINT ( 'NONE',  ( -19.99999999999908695, 17.00000000000000000, 0.000000000000000000 ) ) ;
#4437=ORIENTED_EDGE ( 'NONE', *, *, #27623, .T. ) ;
#4439=EDGE_CURVE ( 'NONE', #17801, #46696, #11200, .T. ) ;
#4447=LINE ( 'NONE', #35513, #5019 ) ;
#4451=ORIENTED_EDGE ( 'NONE', *, *, #45572, .F. ) ;
#4454=ORIENTED_EDGE ( 'NONE', *, *, #16913, .F. ) ;
#4472=VECTOR ( 'NONE', #46300, 1000.000000000000000 ) ;
#4484=EDGE_CURVE ( 'NONE', #17776, #17128, #20147, .T. ) ;
#4493=ORIENTED_EDGE ( 'NONE', *, *, #41816, .F. ) ;
#4494=VECTOR ( 'NONE', #21822, 1000.000000000000000 ) ;
#4509=EDGE_CURVE ( 'NONE', #28907, #572, #16058, .T. ) ;
#4511=ORIENTED_EDGE ( 'NONE', *, *, #21469, .T. ) ;
#4520=ORIENTED_EDGE ( 'NONE', *, *, #46000, .T. ) ;
#4523=DIRECTION ( 'NONE',  ( -3.469446951953611724E-16, 0.000000000000000000, 1.000000000000000000 ) ) ;
#4527=EDGE_CURVE ( 'NONE', #32976, #22529, #35573, .T. ) ;
#4536=AXIS2_PLACEMENT_3D ( 'NONE', #32172, #24726, #32670 ) ;
#4538=VECTOR ( 'NONE', #36400, 1000.000000000000000 ) ;
#4539=ORIENTED_EDGE ( 'NONE', *, *, #3004, .F. ) ;
#4543=ORIENTED_EDGE ( 'NONE', *, *, #47512, .T. ) ;
#4555=PLANE ( 'NONE',  #2993 ) ;
#4567=VECTOR ( 'NONE', #44736, 1000.000000000000000 ) ;
#4568=ORIENTED_EDGE ( 'NONE', *, *, #49970, .T. ) ;
#4578=CARTESIAN_POINT ( 'NONE',  ( -164.9999999999997442, 17.00000000000000000, -84.99999999999998579 ) ) ;
#4579=VECTOR ( 'NONE', #19946, 1000.000000000000000 ) ;
#4580=LINE ( 'NONE', #44545, #21892 ) ;
#4585=DIRECTION ( 'NONE',  ( -1.000000000000000000, 0.000000000000000000, 0.000000000000000000 ) ) ;
#4590=AXIS2_PLACEMENT_3D ( 'NONE', #1653, #32698, #25004 ) ;
#4591=CARTESIAN_POINT ( 'NONE',  ( -65.00000000000002842, 16.00000000000000000, -114.9999999999999858 ) ) ;
#4593=EDGE_CURVE ( 'NONE', #45598, #5571, #919, .T. ) ;
#4594=PLANE ( 'NONE',  #28179 ) ;
#4599=CARTESIAN_POINT ( 'NONE',  ( -19.99999999999878142, 17.00000000000000000, 5.000000000000004441 ) ) ;
#4604=CARTESIAN_POINT ( 'NONE',  ( -64.99999999999815259, 17.00000000000000000, 65.00000000000000000 ) ) ;
#4612=CARTESIAN_POINT ( 'NONE',  ( 135.0000000000006253, 17.00000000000000000, -30.00000000000000000 ) ) ;
#4634=LINE ( 'NONE', #16672, #3256 ) ;
#4644=VECTOR ( 'NONE', #42594, 1000.000000000000000 ) ;
#4649=ADVANCED_FACE ( 'NONE', ( #20653 ), #38293, .F. ) ;
#4657=CARTESIAN_POINT ( 'NONE',  ( -19.99999999999846523, 16.00000000000000000, 35.00000000000000000 ) ) ;
#4660=DIRECTION ( 'NONE',  ( 1.000000000000000000, 0.000000000000000000, -2.312964634635864737E-16 ) ) ;
#4664=VECTOR ( 'NONE', #27657, 1000.000000000000000 ) ;
#4668=CARTESIAN_POINT ( 'NONE',  ( -164.9999999999994031, 17.00000000000000000, -54.99999999999999289 ) ) ;
#4672=LINE ( 'NONE', #44397, #46955 ) ;
#4680=FACE_OUTER_BOUND ( 'NONE', #45680, .T. ) ;
#4684=EDGE_LOOP ( 'NONE', ( #47062, #20099, #110, #37219 ) ) ;
#4685=ORIENTED_EDGE ( 'NONE', *, *, #23613, .F. ) ;
#4689=ADVANCED_FACE ( 'NONE', ( #50517 ), #35196, .F. ) ;
#4691=DIRECTION ( 'NONE',  ( 0.000000000000000000, 0.000000000000000000, 1.000000000000000000 ) ) ;
#4700=ORIENTED_EDGE ( 'NONE', *, *, #14862, .T. ) ;
#4702=ORIENTED_EDGE ( 'NONE', *, *, #12383, .F. ) ;
#4710=LINE ( 'NONE', #47262, #25030 ) ;
#4712=( LENGTH_UNIT ( ) NAMED_UNIT ( * ) SI_UNIT ( .MILLI., .METRE. ) );
#4717=CARTESIAN_POINT ( 'NONE',  ( -114.9999999999991047, 16.00000000000000000, -24.99999999999999289 ) ) ;
#4720=ORIENTED_EDGE ( 'NONE', *, *, #6786, .T. ) ;
#4722=DIRECTION ( 'NONE',  ( 1.000000000000000000, 0.000000000000000000, 0.000000000000000000 ) ) ;
#4725=ORIENTED_EDGE ( 'NONE', *, *, #23850, .F. ) ;
#4728=EDGE_CURVE ( 'NONE', #38804, #36506, #3355, .T. ) ;
#4731=LINE ( 'NONE', #3780, #32041 ) ;
#4736=CARTESIAN_POINT ( 'NONE',  ( 80.00000000000028422, 17.00000000000000000, -84.99999999999998579 ) ) ;
#4760=PLANE ( 'NONE',  #16783 ) ;
#4762=VERTEX_POINT ( 'NONE', #34431 ) ;
#4763=DIRECTION ( 'NONE',  ( -1.000000000000000000, 0.000000000000000000, 0.000000000000000000 ) ) ;
#4785=ORIENTED_EDGE ( 'NONE', *, *, #43874, .T. ) ;
#4791=FACE_OUTER_BOUND ( 'NONE', #13855, .T. ) ;
#4793=DIRECTION ( 'NONE',  ( -0.000000000000000000, -1.000000000000000000, -0.000000000000000000 ) ) ;
#4794=LINE ( 'NONE', #469, #21733 ) ;
#4798=ADVANCED_FACE ( 'NONE', ( #26460 ), #26966, .F. ) ;
#4820=LINE ( 'NONE', #35667, #18329 ) ;
#4821=ORIENTED_EDGE ( 'NONE', *, *, #32289, .T. ) ;
#4843=ORIENTED_EDGE ( 'NONE', *, *, #7323, .T. ) ;
#4851=VERTEX_POINT ( 'NONE', #39288 ) ;
#4852=CARTESIAN_POINT ( 'NONE',  ( -114.9999999999997158, 17.00000000000000000, -84.99999999999998579 ) ) ;
#4856=EDGE_CURVE ( 'NONE', #39319, #34689, #36203, .T. ) ;
#4858=FACE_OUTER_BOUND ( 'NONE', #14635, .T. ) ;
#4859=ADVANCED_FACE ( 'NONE', ( #24149 ), #16437, .F. ) ;
#4861=ADVANCED_FACE ( 'NONE', ( #16949 ), #28492, .F. ) ;
#4876=CARTESIAN_POINT ( 'NONE',  ( 79.99999999999997158, 17.00000000000000000, -114.9999999999999858 ) ) ;
#4882=ORIENTED_EDGE ( 'NONE', *, *, #33394, .F. ) ;
#4903=PLANE ( 'NONE',  #10984 ) ;
#4912=VECTOR ( 'NONE', #47284, 1000.000000000000000 ) ;
#4913=FACE_OUTER_BOUND ( 'NONE', #21349, .T. ) ;
#4917=CARTESIAN_POINT ( 'NONE',  ( -119.9999999999987921, 17.00000000000000000, 30.00000000000000000 ) ) ;
#4920=AXIS2_PLACEMENT_3D ( 'NONE', #47373, #47125, #24346 ) ;
#4921=EDGE_CURVE ( 'NONE', #23363, #45598, #36726, .T. ) ;
#4923=ORIENTED_EDGE ( 'NONE', *, *, #11591, .F. ) ;
#4927=EDGE_CURVE ( 'NONE', #27084, #43076, #48440, .T. ) ;
#4928=LINE ( 'NONE', #12880, #43793 ) ;
#4930=CARTESIAN_POINT ( 'NONE',  ( 85.00000000000056843, 16.00000000000000000, -30.00000000000000000 ) ) ;
#4931=ORIENTED_EDGE ( 'NONE', *, *, #37246, .F. ) ;
#4936=LINE ( 'NONE', #31401, #27188 ) ;
#4942=FACE_OUTER_BOUND ( 'NONE', #33154, .T. ) ;
#4953=VECTOR ( 'NONE', #50294, 1000.000000000000000 ) ;
#4962=FACE_OUTER_BOUND ( 'NONE', #22538, .T. ) ;
#4970=ORIENTED_EDGE ( 'NONE', *, *, #13329, .T. ) ;
#4974=EDGE_CURVE ( 'NONE', #45538, #29858, #6146, .T. ) ;
#4987=VECTOR ( 'NONE', #33155, 1000.000000000000000 ) ;
#5006=ORIENTED_EDGE ( 'NONE', *, *, #39938, .T. ) ;
#5011=ORIENTED_EDGE ( 'NONE', *, *, #7749, .T. ) ;
#5019=VECTOR ( 'NONE', #19580, 1000.000000000000000 ) ;
#5025=CARTESIAN_POINT ( 'NONE',  ( -114.9999999999981526, 17.00000000000000000, 65.00000000000000000 ) ) ;
#5042=FACE_OUTER_BOUND ( 'NONE', #24888, .T. ) ;
#5044=ORIENTED_EDGE ( 'NONE', *, *, #40567, .T. ) ;
#5046=AXIS2_PLACEMENT_3D ( 'NONE', #10177, #29932, #10676 ) ;
#5048=EDGE_LOOP ( 'NONE', ( #40796, #18660, #49133, #47207 ) ) ;
#5050=DIRECTION ( 'NONE',  ( 0.000000000000000000, 0.000000000000000000, 1.000000000000000000 ) ) ;
#5056=ORIENTED_EDGE ( 'NONE', *, *, #34066, .F. ) ;
#5070=CARTESIAN_POINT ( 'NONE',  ( -165.0000000000000284, 16.00000000000000000, -60.00000000000000000 ) ) ;
#5071=CARTESIAN_POINT ( 'NONE',  ( -64.99999999999846523, 17.00000000000000000, 35.00000000000000000 ) ) ;
#5078=DIRECTION ( 'NONE',  ( -0.000000000000000000, -1.000000000000000000, -0.000000000000000000 ) ) ;
#5086=CARTESIAN_POINT ( 'NONE',  ( 84.99999999999997158, 17.00000000000000000, -114.9999999999999858 ) ) ;
#5087=ORIENTED_EDGE ( 'NONE', *, *, #5791, .T. ) ;
#5089=ADVANCED_FACE ( 'NONE', ( #14594 ), #42542, .F. ) ;
#5091=LINE ( 'NONE', #40260, #39952 ) ;
#5096=ORIENTED_EDGE ( 'NONE', *, *, #20669, .F. ) ;
#5100=DIRECTION ( 'NONE',  ( 1.000000000000000000, 0.000000000000000000, 0.000000000000000000 ) ) ;
#5104=LINE ( 'NONE', #48920, #48325 ) ;
#5112=DIRECTION ( 'NONE',  ( 0.000000000000000000, -1.000000000000000000, 0.000000000000000000 ) ) ;
#5113=EDGE_CURVE ( 'NONE', #11032, #7258, #6905, .T. ) ;
#5118=ORIENTED_EDGE ( 'NONE', *, *, #32213, .T. ) ;
#5121=VECTOR ( 'NONE', #11586, 1000.000000000000000 ) ;
#5125=ADVANCED_FACE ( 'NONE', ( #11768 ), #230, .F. ) ;
#5130=EDGE_CURVE ( 'NONE', #8610, #593, #27928, .T. ) ;
#5132=VECTOR ( 'NONE', #42621, 1000.000000000000000 ) ;
#5149=ADVANCED_FACE ( 'NONE', ( #31536 ), #4326, .F. ) ;
#5162=DIRECTION ( 'NONE',  ( -0.000000000000000000, -0.000000000000000000, -1.000000000000000000 ) ) ;
#5169=EDGE_LOOP ( 'NONE', ( #16225, #46487, #29076, #34908 ) ) ;
#5181=CARTESIAN_POINT ( 'NONE',  ( 85.00000000000184741, 17.00000000000000000, 90.00000000000000000 ) ) ;
#5190=LINE ( 'NONE', #35572, #21043 ) ;
#5198=VECTOR ( 'NONE', #3506, 1000.000000000000000 ) ;
#5203=CARTESIAN_POINT ( 'NONE',  ( -175.0000000000000000, 15.00000000000000000, 122.5000000000000142 ) ) ;
#5208=EDGE_CURVE ( 'NONE', #21162, #17655, #21727, .T. ) ;
#5217=EDGE_LOOP ( 'NONE', ( #26376, #30953, #46345, #22316 ) ) ;
#5219=CARTESIAN_POINT ( 'NONE',  ( -69.99999999999847944, 17.00000000000000000, 35.00000000000000000 ) ) ;
#5227=CARTESIAN_POINT ( 'NONE',  ( 135.0000000000012790, 16.00000000000000000, 30.00000000000000000 ) ) ;
#5236=VECTOR ( 'NONE', #17309, 1000.000000000000000 ) ;
#5237=EDGE_CURVE ( 'NONE', #31581, #24012, #33305, .T. ) ;
#5256=ORIENTED_EDGE ( 'NONE', *, *, #25549, .T. ) ;
#5261=EDGE_CURVE ( 'NONE', #38804, #41095, #10189, .T. ) ;
#5263=ORIENTED_EDGE ( 'NONE', *, *, #16747, .T. ) ;
#5268=EDGE_CURVE ( 'NONE', #39269, #42413, #13769, .T. ) ;
#5270=LINE ( 'NONE', #35587, #30947 ) ;
#5277=CARTESIAN_POINT ( 'NONE',  ( -119.9999999999981668, 17.00000000000000000, 90.00000000000000000 ) ) ;
#5280=PLANE ( 'NONE',  #23440 ) ;
#5286=EDGE_LOOP ( 'NONE', ( #33348, #36382, #21791, #17622 ) ) ;
#5294=ORIENTED_EDGE ( 'NONE', *, *, #5261, .F. ) ;
#5303=VECTOR ( 'NONE', #18047, 1000.000000000000000 ) ;
#5310=DIRECTION ( 'NONE',  ( 0.000000000000000000, 0.000000000000000000, -1.000000000000000000 ) ) ;
#5325=EDGE_CURVE ( 'NONE', #42661, #3719, #1245, .T. ) ;
#5334=CARTESIAN_POINT ( 'NONE',  ( 79.99999999999997158, 17.00000000000000000, -114.9999999999999858 ) ) ;
#5346=VECTOR ( 'NONE', #20854, 1000.000000000000000 ) ;
#5347=LINE ( 'NONE', #44824, #40202 ) ;
#5351=DIRECTION ( 'NONE',  ( -0.000000000000000000, -1.000000000000000000, -0.000000000000000000 ) ) ;
#5353=EDGE_LOOP ( 'NONE', ( #24773, #47702, #43505, #11575 ) ) ;
#5370=VECTOR ( 'NONE', #38706, 1000.000000000000000 ) ;
#5372=DIRECTION ( 'NONE',  ( -1.000000000000000000, 0.000000000000000000, -0.000000000000000000 ) ) ;
#5377=ORIENTED_EDGE ( 'NONE', *, *, #34426, .T. ) ;
#5381=VECTOR ( 'NONE', #13271, 1000.000000000000000 ) ;
#5382=AXIS2_PLACEMENT_3D ( 'NONE', #3453, #10158, #33774 ) ;
#5395=VECTOR ( 'NONE', #37270, 1000.000000000000000 ) ;
#5403=FACE_OUTER_BOUND ( 'NONE', #4208, .T. ) ;
#5405=ORIENTED_EDGE ( 'NONE', *, *, #48093, .F. ) ;
#5406=CARTESIAN_POINT ( 'NONE',  ( -14.99999999999845812, 16.00000000000000000, 60.00000000000000000 ) ) ;
#5408=DIRECTION ( 'NONE',  ( -0.000000000000000000, -1.000000000000000000, -0.000000000000000000 ) ) ;
#5409=AXIS2_PLACEMENT_3D ( 'NONE', #28302, #43193, #36275 ) ;
#5410=VERTEX_POINT ( 'NONE', #2978 ) ;
#5418=CARTESIAN_POINT ( 'NONE',  ( -119.9999999999990905, 17.00000000000000000, -24.99999999999999289 ) ) ;
#5431=VECTOR ( 'NONE', #42152, 1000.000000000000000 ) ;
#5432=DIRECTION ( 'NONE',  ( -0.000000000000000000, -1.000000000000000000, -0.000000000000000000 ) ) ;
#5442=ORIENTED_EDGE ( 'NONE', *, *, #29353, .T. ) ;
#5445=VECTOR ( 'NONE', #24901, 1000.000000000000000 ) ;
#5450=DIRECTION ( 'NONE',  ( -1.000000000000000000, 0.000000000000000000, -0.000000000000000000 ) ) ;
#5453=ORIENTED_EDGE ( 'NONE', *, *, #4509, .F. ) ;
#5455=AXIS2_PLACEMENT_3D ( 'NONE', #16608, #12250, #4309 ) ;
#5456=DIRECTION ( 'NONE',  ( 0.000000000000000000, 0.000000000000000000, 1.000000000000000000 ) ) ;
#5461=CARTESIAN_POINT ( 'NONE',  ( -164.9999999999981526, 16.00000000000000000, 90.00000000000000000 ) ) ;
#5464=LINE ( 'NONE', #2373, #5978 ) ;
#5469=DIRECTION ( 'NONE',  ( 1.000000000000000000, 0.000000000000000000, 0.000000000000000000 ) ) ;
#5485=EDGE_CURVE ( 'NONE', #25915, #19067, #8623, .T. ) ;
#5486=DIRECTION ( 'NONE',  ( -0.000000000000000000, -1.000000000000000000, -0.000000000000000000 ) ) ;
#5494=ORIENTED_EDGE ( 'NONE', *, *, #9251, .F. ) ;
#5496=CARTESIAN_POINT ( 'NONE',  ( 0.000000000000000000, 17.00000000000000000, 0.000000000000000000 ) ) ;
#5522=DIRECTION ( 'NONE',  ( 1.000000000000000000, 0.000000000000000000, 0.000000000000000000 ) ) ;
#5530=DIRECTION ( 'NONE',  ( 6.938893903907223447E-16, 0.000000000000000000, 1.000000000000000000 ) ) ;
#5541=LINE ( 'NONE', #13488, #6562 ) ;
#5546=ORIENTED_EDGE ( 'NONE', *, *, #32398, .T. ) ;
#5547=CARTESIAN_POINT ( 'NONE',  ( 130.0000000000005684, 17.00000000000000000, -30.00000000000000000 ) ) ;
#5558=VECTOR ( 'NONE', #42177, 1000.000000000000000 ) ;
#5567=ORIENTED_EDGE ( 'NONE', *, *, #23054, .T. ) ;
#5571=VERTEX_POINT ( 'NONE', #9121 ) ;
#5574=PLANE ( 'NONE',  #1424 ) ;
#5575=CARTESIAN_POINT ( 'NONE',  ( 34.99999999999997868, 17.00000000000000000, -114.9999999999999858 ) ) ;
#5583=CARTESIAN_POINT ( 'NONE',  ( -114.9999999999981526, 17.00000000000000000, 65.00000000000000000 ) ) ;
#5585=VERTEX_POINT ( 'NONE', #9368 ) ;
#5609=CARTESIAN_POINT ( 'NONE',  ( 135.0000000000019043, 17.00000000000000000, 90.00000000000000000 ) ) ;
#5617=VECTOR ( 'NONE', #11838, 1000.000000000000000 ) ;
#5635=DIRECTION ( 'NONE',  ( -0.000000000000000000, -1.000000000000000000, -0.000000000000000000 ) ) ;
#5643=VECTOR ( 'NONE', #7613, 1000.000000000000000 ) ;
#5650=AXIS2_PLACEMENT_3D ( 'NONE', #24908, #17209, #39812 ) ;
#5667=CARTESIAN_POINT ( 'NONE',  ( -119.9999999999987921, 17.00000000000000000, 5.000000000000004441 ) ) ;
#5669=LINE ( 'NONE', #16479, #25336 ) ;
#5670=ORIENTED_EDGE ( 'NONE', *, *, #27288, .T. ) ;
#5671=CARTESIAN_POINT ( 'NONE',  ( 30.00000000000092726, 17.00000000000000000, 0.000000000000000000 ) ) ;
#5678=ORIENTED_EDGE ( 'NONE', *, *, #34132, .T. ) ;
#5682=ORIENTED_EDGE ( 'NONE', *, *, #8710, .F. ) ;
#5690=ORIENTED_EDGE ( 'NONE', *, *, #45622, .F. ) ;
#5695=DIRECTION ( 'NONE',  ( 0.000000000000000000, 0.000000000000000000, 1.000000000000000000 ) ) ;
#5705=CARTESIAN_POINT ( 'NONE',  ( 34.99999999999997868, 17.00000000000000000, -114.9999999999999858 ) ) ;
#5708=CARTESIAN_POINT ( 'NONE',  ( -164.9999999999981526, 16.00000000000000000, 65.00000000000000000 ) ) ;
#5725=VECTOR ( 'NONE', #36971, 1000.000000000000000 ) ;
#5753=VECTOR ( 'NONE', #29588, 1000.000000000000000 ) ;
#5760=CARTESIAN_POINT ( 'NONE',  ( 35.00000000000061107, 17.00000000000000000, -30.00000000000000000 ) ) ;
#5791=EDGE_CURVE ( 'NONE', #3803, #33627, #9506, .T. ) ;
#5792=CARTESIAN_POINT ( 'NONE',  ( 164.9999999999999716, 16.00000000000000000, 115.0000000000000142 ) ) ;
#5794=ORIENTED_EDGE ( 'NONE', *, *, #34974, .T. ) ;
#5797=EDGE_CURVE ( 'NONE', #10318, #22771, #25418, .T. ) ;
#5809=VERTEX_POINT ( 'NONE', #29015 ) ;
#5812=ORIENTED_EDGE ( 'NONE', *, *, #21954, .T. ) ;
#5815=LINE ( 'NONE', #14261, #14347 ) ;
#5820=CARTESIAN_POINT ( 'NONE',  ( -64.99999999999783995, 17.00000000000000000, 95.00000000000000000 ) ) ;
#5822=ORIENTED_EDGE ( 'NONE', *, *, #29641, .F. ) ;
#5832=ADVANCED_FACE ( 'NONE', ( #5403 ), #9757, .F. ) ;
#5836=CARTESIAN_POINT ( 'NONE',  ( 164.9999999999999716, 17.00000000000000000, 34.99999999999999289 ) ) ;
#5837=DIRECTION ( 'NONE',  ( -1.000000000000000000, -0.000000000000000000, -0.000000000000000000 ) ) ;
#5857=PLANE ( 'NONE',  #23829 ) ;
#5879=LINE ( 'NONE', #45353, #50698 ) ;
#5888=CARTESIAN_POINT ( 'NONE',  ( -165.0000000000000284, 15.00000000000000000, 115.0000000000000142 ) ) ;
#5894=CARTESIAN_POINT ( 'NONE',  ( -65.00000000000002842, 17.00000000000000000, -90.00000000000000000 ) ) ;
#5896=DIRECTION ( 'NONE',  ( 0.000000000000000000, -0.000000000000000000, -1.000000000000000000 ) ) ;
#5915=DIRECTION ( 'NONE',  ( -1.000000000000000000, -0.000000000000000000, 4.625929269271584521E-16 ) ) ;
#5926=DIRECTION ( 'NONE',  ( -0.000000000000000000, -1.000000000000000000, -0.000000000000000000 ) ) ;
#5938=EDGE_LOOP ( 'NONE', ( #47149, #38697, #19708, #8780 ) ) ;
#5953=CARTESIAN_POINT ( 'NONE',  ( 35.00000000000028422, 17.00000000000000000, -84.99999999999998579 ) ) ;
#5958=DIRECTION ( 'NONE',  ( 0.000000000000000000, 0.000000000000000000, -1.000000000000000000 ) ) ;
#5959=VERTEX_POINT ( 'NONE', #18462 ) ;
#5963=DIRECTION ( 'NONE',  ( -0.000000000000000000, -1.000000000000000000, -0.000000000000000000 ) ) ;
#5969=ADVANCED_FACE ( 'NONE', ( #6662 ), #2810, .F. ) ;
#5977=EDGE_LOOP ( 'NONE', ( #29681, #17204, #46672, #34831 ) ) ;
#5978=VECTOR ( 'NONE', #21618, 1000.000000000000000 ) ;
#5984=VERTEX_POINT ( 'NONE', #14105 ) ;
#5985=LINE ( 'NONE', #13924, #5753 ) ;
#5993=EDGE_CURVE ( 'NONE', #16365, #3789, #26927, .T. ) ;
#6000=EDGE_LOOP ( 'NONE', ( #35629, #27430, #11990, #50346 ) ) ;
#6008=ORIENTED_EDGE ( 'NONE', *, *, #47342, .T. ) ;
#6011=VERTEX_POINT ( 'NONE', #7182 ) ;
#6018=DIRECTION ( 'NONE',  ( -0.000000000000000000, -1.000000000000000000, -0.000000000000000000 ) ) ;
#6023=ORIENTED_EDGE ( 'NONE', *, *, #39006, .T. ) ;
#6031=VECTOR ( 'NONE', #46909, 1000.000000000000000 ) ;
#6039=ADVANCED_FACE ( 'NONE', ( #45641 ), #15893, .F. ) ;
#6048=ORIENTED_EDGE ( 'NONE', *, *, #22870, .F. ) ;
#6054=CARTESIAN_POINT ( 'NONE',  ( 164.9999999999999716, 17.00000000000000000, 65.00000000000000000 ) ) ;
#6059=VECTOR ( 'NONE', #20162, 1000.000000000000000 ) ;
#6062=ORIENTED_EDGE ( 'NONE', *, *, #12416, .T. ) ;
#6089=EDGE_CURVE ( 'NONE', #33102, #14175, #39251, .T. ) ;
#6104=DIRECTION ( 'NONE',  ( 0.000000000000000000, 0.000000000000000000, 1.000000000000000000 ) ) ;
#6119=EDGE_CURVE ( 'NONE', #43660, #17110, #32311, .T. ) ;
#6122=DIRECTION ( 'NONE',  ( 1.000000000000000000, 0.000000000000000000, 0.000000000000000000 ) ) ;
#6126=EDGE_CURVE ( 'NONE', #43660, #32627, #16908, .T. ) ;
#6130=ORIENTED_EDGE ( 'NONE', *, *, #20040, .F. ) ;
#6132=CARTESIAN_POINT ( 'NONE',  ( 35.00000000000216716, 17.00000000000000000, 95.00000000000000000 ) ) ;
#6133=CARTESIAN_POINT ( 'NONE',  ( -114.9999999999984652, 16.00000000000000000, 35.00000000000000000 ) ) ;
#6146=LINE ( 'NONE', #1549, #36115 ) ;
#6149=EDGE_CURVE ( 'NONE', #35238, #7083, #48151, .T. ) ;
#6151=VECTOR ( 'NONE', #41388, 1000.000000000000000 ) ;
#6157=ORIENTED_EDGE ( 'NONE', *, *, #39006, .F. ) ;
#6161=LINE ( 'NONE', #21815, #21605 ) ;
#6172=CARTESIAN_POINT ( 'NONE',  ( -64.99999999999783995, 16.00000000000000000, 95.00000000000000000 ) ) ;
#6173=VERTEX_POINT ( 'NONE', #45072 ) ;
#6174=CARTESIAN_POINT ( 'NONE',  ( 164.9999999999999716, 17.00000000000000000, 95.00000000000000000 ) ) ;
#6175=EDGE_CURVE ( 'NONE', #4762, #43380, #5347, .T. ) ;
#6178=LINE ( 'NONE', #21835, #1669 ) ;
#6179=DIRECTION ( 'NONE',  ( 1.000000000000000000, 0.000000000000000000, 0.000000000000000000 ) ) ;
#6184=ADVANCED_FACE ( 'NONE', ( #2004 ), #17651, .F. ) ;
#6185=CARTESIAN_POINT ( 'NONE',  ( 85.00000000000213163, 17.00000000000000000, 95.00000000000000000 ) ) ;
#6193=PLANE ( 'NONE',  #1972 ) ;
#6194=ORIENTED_EDGE ( 'NONE', *, *, #31295, .F. ) ;
#6195=EDGE_CURVE ( 'NONE', #42902, #25915, #24363, .T. ) ;
#6206=CARTESIAN_POINT ( 'NONE',  ( -69.99999999999783995, 16.00000000000000000, 115.0000000000000142 ) ) ;
#6210=DIRECTION ( 'NONE',  ( 1.000000000000000000, 0.000000000000000000, -4.625929269271584521E-16 ) ) ;
#6217=VERTEX_POINT ( 'NONE', #24605 ) ;
#6218=DIRECTION ( 'NONE',  ( -0.000000000000000000, -0.000000000000000000, -1.000000000000000000 ) ) ;
#6219=AXIS2_PLACEMENT_3D ( 'NONE', #17809, #45225, #33731 ) ;
#6223=LINE ( 'NONE', #32931, #45232 ) ;
#6227=DIRECTION ( 'NONE',  ( 0.000000000000000000, 0.000000000000000000, -1.000000000000000000 ) ) ;
#6232=DIRECTION ( 'NONE',  ( 0.000000000000000000, 0.000000000000000000, -1.000000000000000000 ) ) ;
#6233=VECTOR ( 'NONE', #13657, 1000.000000000000000 ) ;
#6237=FACE_OUTER_BOUND ( 'NONE', #15261, .T. ) ;
#6243=ORIENTED_EDGE ( 'NONE', *, *, #45572, .T. ) ;
#6246=CARTESIAN_POINT ( 'NONE',  ( -164.9999999999978400, 16.00000000000000000, 95.00000000000000000 ) ) ;
#6249=CARTESIAN_POINT ( 'NONE',  ( -19.99999999999940670, 17.00000000000000000, -54.99999999999999289 ) ) ;
#6251=EDGE_CURVE ( 'NONE', #13654, #27632, #9950, .T. ) ;
#6255=ORIENTED_EDGE ( 'NONE', *, *, #30709, .T. ) ;
#6257=DIRECTION ( 'NONE',  ( 1.000000000000000000, 0.000000000000000000, -0.000000000000000000 ) ) ;
#6262=CARTESIAN_POINT ( 'NONE',  ( 85.00000000000152056, 16.00000000000000000, 35.00000000000000000 ) ) ;
#6280=CARTESIAN_POINT ( 'NONE',  ( -164.9999999999994031, 17.00000000000000000, -30.00000000000000000 ) ) ;
#6284=ORIENTED_EDGE ( 'NONE', *, *, #47110, .T. ) ;
#6292=CARTESIAN_POINT ( 'NONE',  ( 0.000000000000000000, 17.00000000000000000, 0.000000000000000000 ) ) ;
#6314=CARTESIAN_POINT ( 'NONE',  ( -19.99999999999878142, 17.00000000000000000, 5.000000000000004441 ) ) ;
#6336=FACE_OUTER_BOUND ( 'NONE', #25061, .T. ) ;
#6347=FACE_OUTER_BOUND ( 'NONE', #20153, .T. ) ;
#6349=VECTOR ( 'NONE', #9627, 1000.000000000000000 ) ;
#6363=PLANE ( 'NONE',  #13444 ) ;
#6368=ORIENTED_EDGE ( 'NONE', *, *, #17586, .T. ) ;
#6380=LINE ( 'NONE', #29734, #33269 ) ;
#6388=ORIENTED_EDGE ( 'NONE', *, *, #49052, .F. ) ;
#6389=DIRECTION ( 'NONE',  ( 1.000000000000000000, 0.000000000000000000, 0.000000000000000000 ) ) ;
#6395=FACE_BOUND ( 'NONE', #44191, .T. ) ;
#6400=EDGE_CURVE ( 'NONE', #37393, #3284, #45322, .T. ) ;
#6404=LINE ( 'NONE', #37731, #2120 ) ;
#6415=CARTESIAN_POINT ( 'NONE',  ( 35.00000000000216716, 17.00000000000000000, 95.00000000000000000 ) ) ;
#6418=CARTESIAN_POINT ( 'NONE',  ( 80.00000000000186162, 17.00000000000000000, 65.00000000000000000 ) ) ;
#6420=ORIENTED_EDGE ( 'NONE', *, *, #1090, .T. ) ;
#6438=ORIENTED_EDGE ( 'NONE', *, *, #26362, .F. ) ;
#6445=EDGE_CURVE ( 'NONE', #30975, #907, #23536, .T. ) ;
#6454=EDGE_CURVE ( 'NONE', #34191, #20388, #50423, .T. ) ;
#6461=ORIENTED_EDGE ( 'NONE', *, *, #34919, .T. ) ;
#6462=VECTOR ( 'NONE', #11614, 1000.000000000000000 ) ;
#6466=EDGE_CURVE ( 'NONE', #15741, #13767, #11470, .T. ) ;
#6468=DIRECTION ( 'NONE',  ( 0.000000000000000000, 0.000000000000000000, -1.000000000000000000 ) ) ;
#6471=ORIENTED_EDGE ( 'NONE', *, *, #33956, .T. ) ;
#6479=EDGE_LOOP ( 'NONE', ( #33213, #35563, #27771, #2612 ) ) ;
#6481=ORIENTED_EDGE ( 'NONE', *, *, #30533, .T. ) ;
#6496=ORIENTED_EDGE ( 'NONE', *, *, #47690, .F. ) ;
#6497=ORIENTED_EDGE ( 'NONE', *, *, #34401, .F. ) ;
#6504=CARTESIAN_POINT ( 'NONE',  ( 80.00000000000122213, 17.00000000000000000, 5.000000000000004441 ) ) ;
#6506=ORIENTED_EDGE ( 'NONE', *, *, #44322, .T. ) ;
#6510=PLANE ( 'NONE',  #6219 ) ;
#6511=LINE ( 'NONE', #6280, #5236 ) ;
#6519=VECTOR ( 'NONE', #7968, 1000.000000000000000 ) ;
#6520=ORIENTED_EDGE ( 'NONE', *, *, #7095, .T. ) ;
#6523=AXIS2_PLACEMENT_3D ( 'NONE', #27643, #10964, #3502 ) ;
#6524=ORIENTED_EDGE ( 'NONE', *, *, #40567, .F. ) ;
#6525=DIRECTION ( 'NONE',  ( -1.000000000000000000, 0.000000000000000000, 0.000000000000000000 ) ) ;
#6527=LINE ( 'NONE', #32995, #48928 ) ;
#6534=CARTESIAN_POINT ( 'NONE',  ( -19.99999999999908695, 16.00000000000000000, 0.000000000000000000 ) ) ;
#6538=EDGE_CURVE ( 'NONE', #17655, #34173, #20941, .T. ) ;
#6541=EDGE_CURVE ( 'NONE', #10961, #405, #13484, .T. ) ;
#6546=LINE ( 'NONE', #22201, #17979 ) ;
#6554=DIRECTION ( 'NONE',  ( -1.000000000000000000, -0.000000000000000000, -0.000000000000000000 ) ) ;
#6556=CARTESIAN_POINT ( 'NONE',  ( -119.9999999999984652, 17.00000000000000000, 35.00000000000000000 ) ) ;
#6562=VECTOR ( 'NONE', #37876, 1000.000000000000000 ) ;
#6564=ORIENTED_EDGE ( 'NONE', *, *, #47449, .T. ) ;
#6569=VECTOR ( 'NONE', #23296, 1000.000000000000000 ) ;
#6571=EDGE_LOOP ( 'NONE', ( #6023, #6420, #8362, #30515 ) ) ;
#6575=DIRECTION ( 'NONE',  ( -0.000000000000000000, -0.000000000000000000, -1.000000000000000000 ) ) ;
#6583=LINE ( 'NONE', #22234, #39382 ) ;
#6585=DIRECTION ( 'NONE',  ( 0.000000000000000000, 0.000000000000000000, -1.000000000000000000 ) ) ;
#6586=ORIENTED_EDGE ( 'NONE', *, *, #2849, .F. ) ;
#6593=FACE_OUTER_BOUND ( 'NONE', #19243, .T. ) ;
#6594=DIRECTION ( 'NONE',  ( -1.000000000000000000, 0.000000000000000000, 0.000000000000000000 ) ) ;
#6604=VECTOR ( 'NONE', #4255, 1000.000000000000000 ) ;
#6607=ORIENTED_EDGE ( 'NONE', *, *, #44982, .F. ) ;
#6613=LINE ( 'NONE', #2014, #45101 ) ;
#6625=DIRECTION ( 'NONE',  ( 1.000000000000000000, 0.000000000000000000, 0.000000000000000000 ) ) ;
#6629=VERTEX_POINT ( 'NONE', #36625 ) ;
#6631=EDGE_CURVE ( 'NONE', #38172, #7457, #12972, .T. ) ;
#6651=ORIENTED_EDGE ( 'NONE', *, *, #50432, .F. ) ;
#6661=CARTESIAN_POINT ( 'NONE',  ( -65.00000000000002842, 17.00000000000000000, -114.9999999999999858 ) ) ;
#6662=FACE_OUTER_BOUND ( 'NONE', #28009, .T. ) ;
#6664=ORIENTED_EDGE ( 'NONE', *, *, #32113, .T. ) ;
#6668=EDGE_LOOP ( 'NONE', ( #43590, #42292, #30083, #16544 ) ) ;
#6673=VECTOR ( 'NONE', #42889, 1000.000000000000000 ) ;
#6676=ORIENTED_EDGE ( 'NONE', *, *, #7323, .F. ) ;
#6689=ORIENTED_EDGE ( 'NONE', *, *, #15366, .T. ) ;
#6691=EDGE_CURVE ( 'NONE', #32541, #50118, #37120, .T. ) ;
#6692=EDGE_CURVE ( 'NONE', #46399, #31585, #44769, .T. ) ;
#6702=ORIENTED_EDGE ( 'NONE', *, *, #23940, .T. ) ;
#6708=EDGE_LOOP ( 'NONE', ( #41960, #34655, #7524, #47985 ) ) ;
#6710=CARTESIAN_POINT ( 'NONE',  ( 135.0000000000003411, 17.00000000000000000, -60.00000000000000000 ) ) ;
#6719=EDGE_CURVE ( 'NONE', #6011, #45351, #41184, .T. ) ;
#6737=DIRECTION ( 'NONE',  ( -1.000000000000000000, 0.000000000000000000, 0.000000000000000000 ) ) ;
#6742=CARTESIAN_POINT ( 'NONE',  ( -114.9999999999991047, 16.00000000000000000, 0.000000000000000000 ) ) ;
#6743=EDGE_LOOP ( 'NONE', ( #6243, #36241, #2536, #33323 ) ) ;
#6747=CARTESIAN_POINT ( 'NONE',  ( -114.9999999999981526, 16.00000000000000000, 90.00000000000000000 ) ) ;
#6749=VERTEX_POINT ( 'NONE', #7063 ) ;
#6755=ORIENTED_EDGE ( 'NONE', *, *, #28674, .F. ) ;
#6756=CARTESIAN_POINT ( 'NONE',  ( -165.0000000000000284, 16.00000000000000000, 115.0000000000000142 ) ) ;
#6758=DIRECTION ( 'NONE',  ( 1.000000000000000000, 0.000000000000000000, -0.000000000000000000 ) ) ;
#6760=LINE ( 'NONE', #19059, #1408 ) ;
#6763=VECTOR ( 'NONE', #15781, 1000.000000000000000 ) ;
#6767=CARTESIAN_POINT ( 'NONE',  ( -69.99999999999940314, 17.00000000000000000, -54.99999999999999289 ) ) ;
#6786=EDGE_CURVE ( 'NONE', #9357, #22918, #45520, .T. ) ;
#6790=CARTESIAN_POINT ( 'NONE',  ( 35.00000000000061107, 17.00000000000000000, -54.99999999999999289 ) ) ;
#6801=ORIENTED_EDGE ( 'NONE', *, *, #2827, .T. ) ;
#6802=CARTESIAN_POINT ( 'NONE',  ( -15.00000000000001421, 17.00000000000000000, -90.00000000000000000 ) ) ;
#6804=VECTOR ( 'NONE', #27452, 1000.000000000000000 ) ;
#6822=ORIENTED_EDGE ( 'NONE', *, *, #34964, .F. ) ;
#6835=ORIENTED_EDGE ( 'NONE', *, *, #48462, .T. ) ;
#6852=PLANE ( 'NONE',  #34967 ) ;
#6853=DIRECTION ( 'NONE',  ( 0.000000000000000000, 0.000000000000000000, 1.000000000000000000 ) ) ;
#6856=STYLED_ITEM('',(#50754),#39479);
#6879=ORIENTED_EDGE ( 'NONE', *, *, #2276, .F. ) ;
#6881=CARTESIAN_POINT ( 'NONE',  ( -175.0000000000000000, 0.000000000000000000, 122.5000000000000142 ) ) ;
#6900=ADVANCED_FACE ( 'NONE', ( #35541 ), #26815, .F. ) ;
#6901=CARTESIAN_POINT ( 'NONE',  ( -119.9999999999994174, 17.00000000000000000, -30.00000000000000000 ) ) ;
#6903=ORIENTED_EDGE ( 'NONE', *, *, #44836, .F. ) ;
#6905=LINE ( 'NONE', #3040, #13917 ) ;
#6907=VECTOR ( 'NONE', #19140, 1000.000000000000000 ) ;
#6924=CARTESIAN_POINT ( 'NONE',  ( -14.99999999999906919, 16.00000000000000000, -24.99999999999999289 ) ) ;
#6925=DIRECTION ( 'NONE',  ( 0.000000000000000000, 0.000000000000000000, 1.000000000000000000 ) ) ;
#6936=VERTEX_POINT ( 'NONE', #3711 ) ;
#6940=ORIENTED_EDGE ( 'NONE', *, *, #6175, .T. ) ;
#6941=CARTESIAN_POINT ( 'NONE',  ( -164.9999999999987779, 16.00000000000000000, 30.00000000000000000 ) ) ;
#6942=LINE ( 'NONE', #3079, #36393 ) ;
#6975=CARTESIAN_POINT ( 'NONE',  ( -114.9999999999987779, 16.00000000000000000, 5.000000000000004441 ) ) ;
#6978=CARTESIAN_POINT ( 'NONE',  ( -114.9999999999991047, 17.00000000000000000, -24.99999999999999289 ) ) ;
#6988=ORIENTED_EDGE ( 'NONE', *, *, #4509, .T. ) ;
#7007=DIRECTION ( 'NONE',  ( 0.000000000000000000, 0.000000000000000000, 1.000000000000000000 ) ) ;
#7010=VECTOR ( 'NONE', #50048, 1000.000000000000000 ) ;
#7020=DIRECTION ( 'NONE',  ( 1.000000000000000000, 0.000000000000000000, -4.625929269271635797E-16 ) ) ;
#7024=DIRECTION ( 'NONE',  ( -0.000000000000000000, -0.000000000000000000, -1.000000000000000000 ) ) ;
#7026=CARTESIAN_POINT ( 'NONE',  ( 30.00000000000123279, 16.00000000000000000, 5.000000000000004441 ) ) ;
#7030=ORIENTED_EDGE ( 'NONE', *, *, #23116, .T. ) ;
#7031=ORIENTED_EDGE ( 'NONE', *, *, #37246, .T. ) ;
#7034=LINE ( 'NONE', #3159, #47970 ) ;
#7055=EDGE_CURVE ( 'NONE', #48040, #20500, #12670, .T. ) ;
#7063=CARTESIAN_POINT ( 'NONE',  ( 80.00000000000153477, 16.00000000000000000, 35.00000000000000000 ) ) ;
#7069=LINE ( 'NONE', #34524, #16835 ) ;
#7083=VERTEX_POINT ( 'NONE', #20369 ) ;
#7085=LINE ( 'NONE', #26072, #42180 ) ;
#7091=CARTESIAN_POINT ( 'NONE',  ( 35.00000000000152767, 16.00000000000000000, 60.00000000000000000 ) ) ;
#7093=ORIENTED_EDGE ( 'NONE', *, *, #37841, .T. ) ;
#7095=EDGE_CURVE ( 'NONE', #22294, #39423, #47781, .T. ) ;
#7099=EDGE_LOOP ( 'NONE', ( #38413, #49678, #30253, #13879 ) ) ;
#7104=LINE ( 'NONE', #26851, #48313 ) ;
#7108=CARTESIAN_POINT ( 'NONE',  ( 135.0000000000000000, 16.00000000000000000, -114.9999999999999858 ) ) ;
#7109=DIRECTION ( 'NONE',  ( 0.000000000000000000, 0.000000000000000000, -1.000000000000000000 ) ) ;
#7117=EDGE_CURVE ( 'NONE', #36660, #2139, #21899, .T. ) ;
#7119=CARTESIAN_POINT ( 'NONE',  ( -64.99999999999877787, 17.00000000000000000, 5.000000000000004441 ) ) ;
#7124=VECTOR ( 'NONE', #24884, 1000.000000000000000 ) ;
#7126=VERTEX_POINT ( 'NONE', #6249 ) ;
#7129=CARTESIAN_POINT ( 'NONE',  ( -164.9999999999984936, 17.00000000000000000, 60.00000000000000000 ) ) ;
#7134=ORIENTED_EDGE ( 'NONE', *, *, #30959, .T. ) ;
#7139=DIRECTION ( 'NONE',  ( 0.000000000000000000, 0.000000000000000000, -1.000000000000000000 ) ) ;
#7161=DIRECTION ( 'NONE',  ( 0.000000000000000000, -1.000000000000000000, 0.000000000000000000 ) ) ;
#7182=CARTESIAN_POINT ( 'NONE',  ( 30.00000000000187228, 16.00000000000000000, 90.00000000000000000 ) ) ;
#7187=ORIENTED_EDGE ( 'NONE', *, *, #16757, .T. ) ;
#7190=EDGE_CURVE ( 'NONE', #36, #10961, #38821, .T. ) ;
#7196=VECTOR ( 'NONE', #29436, 1000.000000000000000 ) ;
#7198=LINE ( 'NONE', #49492, #48275 ) ;
#7205=ORIENTED_EDGE ( 'NONE', *, *, #50324, .T. ) ;
#7221=DIRECTION ( 'NONE',  ( 1.000000000000000000, 0.000000000000000000, 0.000000000000000000 ) ) ;
#7222=CARTESIAN_POINT ( 'NONE',  ( -14.99999999999937472, 17.00000000000000000, -54.99999999999999289 ) ) ;
#7228=VERTEX_POINT ( 'NONE', #31108 ) ;
#7239=DIRECTION ( 'NONE',  ( -1.000000000000000000, -0.000000000000000000, -0.000000000000000000 ) ) ;
#7250=ORIENTED_EDGE ( 'NONE', *, *, #38192, .F. ) ;
#7258=VERTEX_POINT ( 'NONE', #46714 ) ;
#7259=VERTEX_POINT ( 'NONE', #7511 ) ;
#7268=ORIENTED_EDGE ( 'NONE', *, *, #22763, .T. ) ;
#7269=CARTESIAN_POINT ( 'NONE',  ( -164.9999999999984936, 16.00000000000000000, 60.00000000000000000 ) ) ;
#7271=DIRECTION ( 'NONE',  ( 1.000000000000000000, 0.000000000000000000, 0.000000000000000000 ) ) ;
#7276=ORIENTED_EDGE ( 'NONE', *, *, #5130, .F. ) ;
#7282=ORIENTED_EDGE ( 'NONE', *, *, #32740, .F. ) ;
#7285=DIRECTION ( 'NONE',  ( 0.000000000000000000, 0.000000000000000000, -1.000000000000000000 ) ) ;
#7294=CARTESIAN_POINT ( 'NONE',  ( -64.99999999999909051, 17.00000000000000000, 0.000000000000000000 ) ) ;
#7302=VECTOR ( 'NONE', #17266, 1000.000000000000000 ) ;
#7309=EDGE_CURVE ( 'NONE', #35301, #17811, #42130, .T. ) ;
#7311=EDGE_CURVE ( 'NONE', #11806, #6011, #72, .T. ) ;
#7323=EDGE_CURVE ( 'NONE', #41885, #35737, #3130, .T. ) ;
#7334=VECTOR ( 'NONE', #44332, 1000.000000000000000 ) ;
#7335=CARTESIAN_POINT ( 'NONE',  ( -119.9999999999994174, 16.00000000000000000, -30.00000000000000000 ) ) ;
#7340=EDGE_CURVE ( 'NONE', #1481, #23962, #43399, .T. ) ;
#7344=CARTESIAN_POINT ( 'NONE',  ( 80.00000000000216005, 17.00000000000000000, 95.00000000000000000 ) ) ;
#7348=VECTOR ( 'NONE', #22231, 1000.000000000000000 ) ;
#7349=EDGE_CURVE ( 'NONE', #23722, #41220, #28274, .T. ) ;
#7350=AXIS2_PLACEMENT_3D ( 'NONE', #7477, #23106, #16184 ) ;
#7359=DIRECTION ( 'NONE',  ( -1.000000000000000000, 0.000000000000000000, -0.000000000000000000 ) ) ;
#7360=EDGE_LOOP ( 'NONE', ( #30920, #23282, #13409, #16400 ) ) ;
#7366=CARTESIAN_POINT ( 'NONE',  ( 35.00000000000028422, 17.00000000000000000, -60.00000000000000000 ) ) ;
#7387=VECTOR ( 'NONE', #36516, 1000.000000000000000 ) ;
#7389=VECTOR ( 'NONE', #20025, 1000.000000000000000 ) ;
#7402=DIRECTION ( 'NONE',  ( -0.000000000000000000, -1.000000000000000000, -0.000000000000000000 ) ) ;
#7410=FACE_OUTER_BOUND ( 'NONE', #44592, .T. ) ;
#7423=FACE_BOUND ( 'NONE', #2986, .T. ) ;
#7431=VECTOR ( 'NONE', #41548, 1000.000000000000000 ) ;
#7432=LINE ( 'NONE', #8699, #31408 ) ;
#7437=EDGE_CURVE ( 'NONE', #9086, #6173, #31882, .T. ) ;
#7438=DIRECTION ( 'NONE',  ( 0.000000000000000000, 0.000000000000000000, 1.000000000000000000 ) ) ;
#7443=DIRECTION ( 'NONE',  ( -1.000000000000000000, -0.000000000000000000, -0.000000000000000000 ) ) ;
#7452=CARTESIAN_POINT ( 'NONE',  ( -64.99999999999940314, 17.00000000000000000, -30.00000000000000000 ) ) ;
#7457=VERTEX_POINT ( 'NONE', #41758 ) ;
#7464=LINE ( 'NONE', #38766, #35760 ) ;
#7466=ORIENTED_EDGE ( 'NONE', *, *, #16868, .T. ) ;
#7468=VERTEX_POINT ( 'NONE', #26370 ) ;
#7477=CARTESIAN_POINT ( 'NONE',  ( 35.00000000000216716, 17.00000000000000000, 95.00000000000000000 ) ) ;
#7485=EDGE_CURVE ( 'NONE', #27386, #38025, #49163, .T. ) ;
#7492=VECTOR ( 'NONE', #34474, 1000.000000000000000 ) ;
#7493=ORIENTED_EDGE ( 'NONE', *, *, #3463, .F. ) ;
#7502=VECTOR ( 'NONE', #18151, 1000.000000000000000 ) ;
#7505=VERTEX_POINT ( 'NONE', #34322 ) ;
#7507=CARTESIAN_POINT ( 'NONE',  ( 130.0000000000005684, 17.00000000000000000, -54.99999999999999289 ) ) ;
#7508=ORIENTED_EDGE ( 'NONE', *, *, #35288, .T. ) ;
#7511=CARTESIAN_POINT ( 'NONE',  ( -14.99999999999845812, 17.00000000000000000, 60.00000000000000000 ) ) ;
#7514=DIRECTION ( 'NONE',  ( 0.000000000000000000, -0.000000000000000000, -1.000000000000000000 ) ) ;
#7519=UNCERTAINTY_MEASURE_WITH_UNIT (LENGTH_MEASURE( 1.000000000000000082E-05 ), #4712, 'distance_accuracy_value', 'NONE');
#7523=ORIENTED_EDGE ( 'NONE', *, *, #794, .T. ) ;
#7524=ORIENTED_EDGE ( 'NONE', *, *, #21872, .F. ) ;
#7528=ORIENTED_EDGE ( 'NONE', *, *, #971, .T. ) ;
#7529=VECTOR ( 'NONE', #16963, 1000.000000000000000 ) ;
#7538=EDGE_CURVE ( 'NONE', #45021, #39034, #38196, .T. ) ;
#7539=DIRECTION ( 'NONE',  ( -1.000000000000000000, -0.000000000000000000, -0.000000000000000000 ) ) ;
#7544=EDGE_CURVE ( 'NONE', #36600, #15720, #3007, .T. ) ;
#7550=PLANE ( 'NONE',  #36510 ) ;
#7557=VERTEX_POINT ( 'NONE', #33829 ) ;
#7561=PLANE ( 'NONE',  #42488 ) ;
#7564=VECTOR ( 'NONE', #4224, 1000.000000000000000 ) ;
#7566=AXIS2_PLACEMENT_3D ( 'NONE', #5496, #24256, #12933 ) ;
#7567=CARTESIAN_POINT ( 'NONE',  ( -115.0000000000000284, 17.00000000000000000, -90.00000000000000000 ) ) ;
#7581=EDGE_LOOP ( 'NONE', ( #21016, #22608, #26068, #5678 ) ) ;
#7592=PLANE ( 'NONE',  #39058 ) ;
#7593=ORIENTED_EDGE ( 'NONE', *, *, #6541, .F. ) ;
#7594=DIRECTION ( 'NONE',  ( -0.000000000000000000, -1.000000000000000000, -0.000000000000000000 ) ) ;
#7596=DIRECTION ( 'NONE',  ( 0.000000000000000000, -0.000000000000000000, -1.000000000000000000 ) ) ;
#7613=DIRECTION ( 'NONE',  ( 1.000000000000000000, 0.000000000000000000, 0.000000000000000000 ) ) ;
#7626=CARTESIAN_POINT ( 'NONE',  ( 130.0000000000015064, 17.00000000000000000, 35.00000000000000000 ) ) ;
#7636=ORIENTED_EDGE ( 'NONE', *, *, #14680, .T. ) ;
#7644=VERTEX_POINT ( 'NONE', #19682 ) ;
#7650=EDGE_CURVE ( 'NONE', #23917, #42991, #23791, .T. ) ;
#7652=LINE ( 'NONE', #38963, #10256 ) ;
#7655=ADVANCED_FACE ( 'NONE', ( #39955 ), #12233, .F. ) ;
#7657=ADVANCED_FACE ( 'NONE', ( #20186 ), #198, .F. ) ;
#7659=AXIS2_PLACEMENT_3D ( 'NONE', #9704, #9959, #8957 ) ;
#7662=ORIENTED_EDGE ( 'NONE', *, *, #35284, .F. ) ;
#7663=CARTESIAN_POINT ( 'NONE',  ( 85.00000000000056843, 17.00000000000000000, -54.99999999999999289 ) ) ;
#7668=ADVANCED_FACE ( 'NONE', ( #47341 ), #27898, .F. ) ;
#7671=CARTESIAN_POINT ( 'NONE',  ( -114.9999999999978542, 17.00000000000000000, 115.0000000000000142 ) ) ;
#7679=FACE_OUTER_BOUND ( 'NONE', #23290, .T. ) ;
#7683=VECTOR ( 'NONE', #30128, 1000.000000000000000 ) ;
#7685=LINE ( 'NONE', #49716, #17509 ) ;
#7687=EDGE_LOOP ( 'NONE', ( #26628, #14716, #26841, #21055 ) ) ;
#7689=CARTESIAN_POINT ( 'NONE',  ( -119.9999999999990905, 16.00000000000000000, 0.000000000000000000 ) ) ;
#7690=LINE ( 'NONE', #26926, #16837 ) ;
#7692=ADVANCED_FACE ( 'NONE', ( #11478 ), #39199, .F. ) ;
#7694=EDGE_CURVE ( 'NONE', #10222, #18457, #46837, .T. ) ;
#7695=ORIENTED_EDGE ( 'NONE', *, *, #27088, .F. ) ;
#7698=ORIENTED_EDGE ( 'NONE', *, *, #34656, .T. ) ;
#7702=DIRECTION ( 'NONE',  ( 1.000000000000000000, 0.000000000000000000, 0.000000000000000000 ) ) ;
#7706=ORIENTED_EDGE ( 'NONE', *, *, #16792, .F. ) ;
#7711=ORIENTED_EDGE ( 'NONE', *, *, #46471, .T. ) ;
#7715=LINE ( 'NONE', #49992, #4095 ) ;
#7737=CARTESIAN_POINT ( 'NONE',  ( 85.00000000000152056, 17.00000000000000000, 35.00000000000000000 ) ) ;
#7742=ORIENTED_EDGE ( 'NONE', *, *, #30355, .F. ) ;
#7748=DIRECTION ( 'NONE',  ( 1.000000000000000000, 0.000000000000000000, 0.000000000000000000 ) ) ;
#7749=EDGE_CURVE ( 'NONE', #12984, #23377, #44024, .T. ) ;
#7771=EDGE_CURVE ( 'NONE', #49813, #39284, #40455, .T. ) ;
#7773=EDGE_LOOP ( 'NONE', ( #14732, #41715, #1785, #27743 ) ) ;
#7787=CARTESIAN_POINT ( 'NONE',  ( -114.9999999999994031, 16.00000000000000000, -54.99999999999999289 ) ) ;
#7790=CARTESIAN_POINT ( 'NONE',  ( 34.99999999999997868, 16.00000000000000000, -90.00000000000000000 ) ) ;
#7811=DIRECTION ( 'NONE',  ( 0.000000000000000000, -0.000000000000000000, -1.000000000000000000 ) ) ;
#7813=DIRECTION ( 'NONE',  ( 0.000000000000000000, 0.000000000000000000, 1.000000000000000000 ) ) ;
#7822=LINE ( 'NONE', #31426, #36778 ) ;
#7830=FACE_OUTER_BOUND ( 'NONE', #44358, .T. ) ;
#7859=FACE_OUTER_BOUND ( 'NONE', #8897, .T. ) ;
#7860=CARTESIAN_POINT ( 'NONE',  ( -164.9999999999987779, 17.00000000000000000, 30.00000000000000000 ) ) ;
#7865=ORIENTED_EDGE ( 'NONE', *, *, #11591, .T. ) ;
#7870=VERTEX_POINT ( 'NONE', #33511 ) ;
#7871=EDGE_CURVE ( 'NONE', #418, #5585, #26314, .T. ) ;
#7877=LINE ( 'NONE', #23521, #18742 ) ;
#7884=DIRECTION ( 'NONE',  ( 1.000000000000000000, 0.000000000000000000, 0.000000000000000000 ) ) ;
#7892=AXIS2_PLACEMENT_3D ( 'NONE', #23735, #35819, #39404 ) ;
#7899=EDGE_CURVE ( 'NONE', #27098, #45593, #21953, .T. ) ;
#7920=CARTESIAN_POINT ( 'NONE',  ( 135.0000000000015632, 16.00000000000000000, 60.00000000000000000 ) ) ;
#7921=VECTOR ( 'NONE', #14402, 1000.000000000000000 ) ;
#7932=VECTOR ( 'NONE', #16235, 1000.000000000000000 ) ;
#7936=CARTESIAN_POINT ( 'NONE',  ( -64.99999999999909051, 17.00000000000000000, -24.99999999999999289 ) ) ;
#7941=DIRECTION ( 'NONE',  ( 0.000000000000000000, 0.000000000000000000, 1.000000000000000000 ) ) ;
#7959=EDGE_CURVE ( 'NONE', #34874, #30968, #21694, .T. ) ;
#7965=VECTOR ( 'NONE', #11123, 1000.000000000000000 ) ;
#7968=DIRECTION ( 'NONE',  ( -0.000000000000000000, -1.000000000000000000, -0.000000000000000000 ) ) ;
#7971=LINE ( 'NONE', #22591, #32778 ) ;
#7976=CARTESIAN_POINT ( 'NONE',  ( -165.0000000000000284, 16.00000000000000000, -114.9999999999999858 ) ) ;
#7983=FACE_OUTER_BOUND ( 'NONE', #16547, .T. ) ;
#7997=EDGE_CURVE ( 'NONE', #41585, #27664, #50364, .T. ) ;
#8001=VERTEX_POINT ( 'NONE', #35545 ) ;
#8009=ORIENTED_EDGE ( 'NONE', *, *, #20165, .F. ) ;
#8024=CARTESIAN_POINT ( 'NONE',  ( -14.99999999999906919, 16.00000000000000000, 0.000000000000000000 ) ) ;
#8026=DIRECTION ( 'NONE',  ( -0.000000000000000000, -1.000000000000000000, -0.000000000000000000 ) ) ;
#8039=ORIENTED_EDGE ( 'NONE', *, *, #19692, .T. ) ;
#8040=LINE ( 'NONE', #7790, #35624 ) ;
#8055=EDGE_LOOP ( 'NONE', ( #11064, #23799, #36833, #24824 ) ) ;
#8063=ORIENTED_EDGE ( 'NONE', *, *, #4044, .T. ) ;
#8065=PLANE ( 'NONE',  #34857 ) ;
#8069=DIRECTION ( 'NONE',  ( -0.000000000000000000, -1.000000000000000000, -0.000000000000000000 ) ) ;
#8073=ORIENTED_EDGE ( 'NONE', *, *, #20226, .T. ) ;
#8088=CARTESIAN_POINT ( 'NONE',  ( 35.00000000000028422, 16.00000000000000000, -84.99999999999998579 ) ) ;
#8092=PLANE ( 'NONE',  #7892 ) ;
#8100=EDGE_LOOP ( 'NONE', ( #32067, #29360, #29865, #4785 ) ) ;
#8101=ORIENTED_EDGE ( 'NONE', *, *, #38820, .T. ) ;
#8102=EDGE_LOOP ( 'NONE', ( #42979, #18110, #18413, #46439 ) ) ;
#8116=ORIENTED_EDGE ( 'NONE', *, *, #20542, .F. ) ;
#8137=DIRECTION ( 'NONE',  ( -0.000000000000000000, -0.000000000000000000, -1.000000000000000000 ) ) ;
#8138=AXIS2_PLACEMENT_3D ( 'NONE', #11867, #27527, #7514 ) ;
#8148=ORIENTED_EDGE ( 'NONE', *, *, #5237, .F. ) ;
#8159=CARTESIAN_POINT ( 'NONE',  ( -114.9999999999981526, 17.00000000000000000, 65.00000000000000000 ) ) ;
#8160=VECTOR ( 'NONE', #2967, 1000.000000000000000 ) ;
#8174=LINE ( 'NONE', #38974, #41801 ) ;
#8189=VECTOR ( 'NONE', #41024, 1000.000000000000000 ) ;
#8190=VECTOR ( 'NONE', #21831, 1000.000000000000000 ) ;
#8196=LINE ( 'NONE', #39246, #33058 ) ;
#8199=LINE ( 'NONE', #39504, #40105 ) ;
#8207=VERTEX_POINT ( 'NONE', #21382 ) ;
#8210=PLANE ( 'NONE',  #32847 ) ;
#8213=EDGE_LOOP ( 'NONE', ( #40311, #17819, #47034, #17786 ) ) ;
#8221=CARTESIAN_POINT ( 'NONE',  ( -114.9999999999978542, 16.00000000000000000, 95.00000000000000000 ) ) ;
#8226=VECTOR ( 'NONE', #28010, 1000.000000000000000 ) ;
#8235=DIRECTION ( 'NONE',  ( -0.000000000000000000, -1.000000000000000000, -0.000000000000000000 ) ) ;
#8238=DIRECTION ( 'NONE',  ( -0.000000000000000000, -0.000000000000000000, 1.000000000000000000 ) ) ;
#8243=PLANE ( 'NONE',  #16892 ) ;
#8261=ORIENTED_EDGE ( 'NONE', *, *, #14011, .F. ) ;
#8271=LINE ( 'NONE', #32632, #15020 ) ;
#8275=EDGE_CURVE ( 'NONE', #17128, #5984, #10846, .T. ) ;
#8282=LINE ( 'NONE', #46721, #43416 ) ;
#8302=ORIENTED_EDGE ( 'NONE', *, *, #27093, .T. ) ;
#8315=ADVANCED_FACE ( 'NONE', ( #33459 ), #13927, .F. ) ;
#8321=CARTESIAN_POINT ( 'NONE',  ( -70.00000000000002842, 17.00000000000000000, -90.00000000000000000 ) ) ;
#8326=FACE_OUTER_BOUND ( 'NONE', #1770, .T. ) ;
#8331=LINE ( 'NONE', #23978, #3250 ) ;
#8336=EDGE_CURVE ( 'NONE', #4263, #37483, #8282, .T. ) ;
#8339=ADVANCED_FACE ( 'NONE', ( #50303 ), #19811, .F. ) ;
#8340=CARTESIAN_POINT ( 'NONE',  ( -69.99999999999909051, 17.00000000000000000, -24.99999999999999289 ) ) ;
#8343=VECTOR ( 'NONE', #37064, 1000.000000000000000 ) ;
#8344=ORIENTED_EDGE ( 'NONE', *, *, #7544, .T. ) ;
#8351=ORIENTED_EDGE ( 'NONE', *, *, #4439, .F. ) ;
#8361=CARTESIAN_POINT ( 'NONE',  ( 85.00000000000090949, 17.00000000000000000, -24.99999999999999289 ) ) ;
#8362=ORIENTED_EDGE ( 'NONE', *, *, #29139, .T. ) ;
#8373=EDGE_LOOP ( 'NONE', ( #41061, #28074, #33523, #19635 ) ) ;
#8388=VECTOR ( 'NONE', #33968, 1000.000000000000000 ) ;
#8397=CARTESIAN_POINT ( 'NONE',  ( -175.0000000000000000, 15.00000000000000000, 122.5000000000000142 ) ) ;
#8399=CARTESIAN_POINT ( 'NONE',  ( -64.99999999999940314, 17.00000000000000000, -30.00000000000000000 ) ) ;
#8405=ORIENTED_EDGE ( 'NONE', *, *, #2412, .F. ) ;
#8406=DIRECTION ( 'NONE',  ( -1.000000000000000000, -0.000000000000000000, -0.000000000000000000 ) ) ;
#8412=VECTOR ( 'NONE', #44971, 1000.000000000000000 ) ;
#8421=LINE ( 'NONE', #7920, #4579 ) ;
#8422=ORIENTED_EDGE ( 'NONE', *, *, #1983, .T. ) ;
#8444=DIRECTION ( 'NONE',  ( -0.000000000000000000, -1.000000000000000000, -0.000000000000000000 ) ) ;
#8457=EDGE_CURVE ( 'NONE', #7083, #49071, #9526, .T. ) ;
#8460=EDGE_LOOP ( 'NONE', ( #47594, #1711, #45817, #14173 ) ) ;
#8462=LINE ( 'NONE', #23857, #8472 ) ;
#8463=DIRECTION ( 'NONE',  ( 0.000000000000000000, 0.000000000000000000, 1.000000000000000000 ) ) ;
#8472=VECTOR ( 'NONE', #39516, 1000.000000000000000 ) ;
#8474=DIRECTION ( 'NONE',  ( -0.000000000000000000, -1.000000000000000000, -0.000000000000000000 ) ) ;
#8475=LINE ( 'NONE', #8733, #11970 ) ;
#8476=EDGE_CURVE ( 'NONE', #43115, #13598, #44159, .T. ) ;
#8481=VECTOR ( 'NONE', #46139, 1000.000000000000000 ) ;
#8488=CARTESIAN_POINT ( 'NONE',  ( 135.0000000000012790, 17.00000000000000000, 5.000000000000004441 ) ) ;
#8492=CARTESIAN_POINT ( 'NONE',  ( -14.99999999999845812, 17.00000000000000000, 35.00000000000000000 ) ) ;
#8517=DIRECTION ( 'NONE',  ( -0.000000000000000000, -1.000000000000000000, -0.000000000000000000 ) ) ;
#8524=LINE ( 'NONE', #27516, #4953 ) ;
#8525=FACE_OUTER_BOUND ( 'NONE', #48560, .T. ) ;
#8533=CARTESIAN_POINT ( 'NONE',  ( -69.99999999999847944, 17.00000000000000000, 60.00000000000000000 ) ) ;
#8542=DIRECTION ( 'NONE',  ( -0.000000000000000000, -1.000000000000000000, -0.000000000000000000 ) ) ;
#8545=VECTOR ( 'NONE', #39467, 1000.000000000000000 ) ;
#8546=CARTESIAN_POINT ( 'NONE',  ( -14.99999999999937472, 16.00000000000000000, -54.99999999999999289 ) ) ;
#8549=VECTOR ( 'NONE', #43646, 1000.000000000000000 ) ;
#8553=DIRECTION ( 'NONE',  ( 1.000000000000000000, 0.000000000000000000, -0.000000000000000000 ) ) ;
#8569=VECTOR ( 'NONE', #10192, 1000.000000000000000 ) ;
#8590=DIRECTION ( 'NONE',  ( 1.000000000000000000, 0.000000000000000000, 0.000000000000000000 ) ) ;
#8598=VECTOR ( 'NONE', #38869, 1000.000000000000000 ) ;
#8610=VERTEX_POINT ( 'NONE', #8789 ) ;
#8623=LINE ( 'NONE', #39931, #42801 ) ;
#8633=FACE_OUTER_BOUND ( 'NONE', #9362, .T. ) ;
#8634=EDGE_CURVE ( 'NONE', #25941, #9086, #34167, .T. ) ;
#8653=VECTOR ( 'NONE', #40226, 1000.000000000000000 ) ;
#8665=ORIENTED_EDGE ( 'NONE', *, *, #11415, .T. ) ;
#8671=ORIENTED_EDGE ( 'NONE', *, *, #28628, .F. ) ;
#8673=FACE_OUTER_BOUND ( 'NONE', #36897, .T. ) ;
#8674=LINE ( 'NONE', #20449, #14421 ) ;
#8675=VECTOR ( 'NONE', #12424, 1000.000000000000000 ) ;
#8684=DIRECTION ( 'NONE',  ( 0.000000000000000000, 0.000000000000000000, 1.000000000000000000 ) ) ;
#8699=CARTESIAN_POINT ( 'NONE',  ( -64.99999999999971578, 17.00000000000000000, -84.99999999999998579 ) ) ;
#8700=AXIS2_PLACEMENT_3D ( 'NONE', #23877, #11828, #43613 ) ;
#8702=VECTOR ( 'NONE', #13933, 1000.000000000000000 ) ;
#8707=LINE ( 'NONE', #20737, #46988 ) ;
#8710=EDGE_CURVE ( 'NONE', #45864, #17776, #38765, .T. ) ;
#8716=LINE ( 'NONE', #4604, #2669 ) ;
#8717=AXIS2_PLACEMENT_3D ( 'NONE', #16423, #15924, #28233 ) ;
#8732=CARTESIAN_POINT ( 'NONE',  ( 80.00000000000153477, 17.00000000000000000, 35.00000000000000000 ) ) ;
#8733=CARTESIAN_POINT ( 'NONE',  ( 35.00000000000091660, 17.00000000000000000, 0.000000000000000000 ) ) ;
#8736=EDGE_LOOP ( 'NONE', ( #24943, #33909, #5087, #14298 ) ) ;
#8742=SHAPE_REPRESENTATION ( 'solar panel', ( #45486 ), #32386 ) ;
#8743=EDGE_LOOP ( 'NONE', ( #16432, #14192, #6879, #5546 ) ) ;
#8746=ORIENTED_EDGE ( 'NONE', *, *, #20317, .T. ) ;
#8757=FACE_OUTER_BOUND ( 'NONE', #28923, .T. ) ;
#8768=ORIENTED_EDGE ( 'NONE', *, *, #35761, .F. ) ;
#8770=PLANE ( 'NONE',  #49258 ) ;
#8771=EDGE_CURVE ( 'NONE', #23064, #35976, #7715, .T. ) ;
#8780=ORIENTED_EDGE ( 'NONE', *, *, #3194, .T. ) ;
#8786=CARTESIAN_POINT ( 'NONE',  ( -114.9999999999994031, 16.00000000000000000, -30.00000000000000000 ) ) ;
#8788=LINE ( 'NONE', #40583, #44306 ) ;
#8789=CARTESIAN_POINT ( 'NONE',  ( -19.99999999999846523, 17.00000000000000000, 35.00000000000000000 ) ) ;
#8791=EDGE_CURVE ( 'NONE', #13767, #42432, #7971, .T. ) ;
#8794=DIRECTION ( 'NONE',  ( -0.000000000000000000, -1.000000000000000000, -0.000000000000000000 ) ) ;
#8797=ORIENTED_EDGE ( 'NONE', *, *, #46791, .F. ) ;
#8811=LINE ( 'NONE', #28554, #19979 ) ;
#8813=VERTEX_POINT ( 'NONE', #8732 ) ;
#8821=CARTESIAN_POINT ( 'NONE',  ( -119.9999999999984652, 17.00000000000000000, 35.00000000000000000 ) ) ;
#8824=ORIENTED_EDGE ( 'NONE', *, *, #21778, .T. ) ;
#8825=EDGE_CURVE ( 'NONE', #32291, #10429, #24381, .T. ) ;
#8827=CARTESIAN_POINT ( 'NONE',  ( 30.00000000000062172, 17.00000000000000000, -54.99999999999999289 ) ) ;
#8835=ORIENTED_EDGE ( 'NONE', *, *, #33042, .T. ) ;
#8839=CARTESIAN_POINT ( 'NONE',  ( -114.9999999999981526, 16.00000000000000000, 65.00000000000000000 ) ) ;
#8841=VERTEX_POINT ( 'NONE', #16410 ) ;
#8846=EDGE_LOOP ( 'NONE', ( #29349, #46, #33778, #18756 ) ) ;
#8849=CARTESIAN_POINT ( 'NONE',  ( -114.9999999999978542, 17.00000000000000000, 115.0000000000000142 ) ) ;
#8850=PLANE ( 'NONE',  #14113 ) ;
#8861=ORIENTED_EDGE ( 'NONE', *, *, #45295, .F. ) ;
#8870=ADVANCED_FACE ( 'NONE', ( #32839 ), #36181, .F. ) ;
#8875=LINE ( 'NONE', #24033, #2568 ) ;
#8879=ADVANCED_FACE ( 'NONE', ( #27714 ), #31832, .F. ) ;
#8881=CARTESIAN_POINT ( 'NONE',  ( 129.9999999999999432, 17.00000000000000000, -90.00000000000000000 ) ) ;
#8885=CARTESIAN_POINT ( 'NONE',  ( 135.0000000000006253, 16.00000000000000000, -30.00000000000000000 ) ) ;
#8897=EDGE_LOOP ( 'NONE', ( #27285, #31828, #17440, #29243 ) ) ;
#8929=EDGE_CURVE ( 'NONE', #17047, #50635, #5104, .T. ) ;
#8934=CARTESIAN_POINT ( 'NONE',  ( -64.99999999999815259, 16.00000000000000000, 90.00000000000000000 ) ) ;
#8935=EDGE_CURVE ( 'NONE', #34164, #7228, #2269, .T. ) ;
#8936=DIRECTION ( 'NONE',  ( 0.000000000000000000, 0.000000000000000000, 1.000000000000000000 ) ) ;
#8939=ADVANCED_FACE ( 'NONE', ( #49177 ), #25631, .F. ) ;
#8954=ORIENTED_EDGE ( 'NONE', *, *, #30646, .F. ) ;
#8957=DIRECTION ( 'NONE',  ( 0.000000000000000000, -0.000000000000000000, -1.000000000000000000 ) ) ;
#8963=VECTOR ( 'NONE', #33505, 1000.000000000000000 ) ;
#8978=DIRECTION ( 'NONE',  ( 0.000000000000000000, -0.000000000000000000, -1.000000000000000000 ) ) ;
#8981=PLANE ( 'NONE',  #23473 ) ;
#8985=CARTESIAN_POINT ( 'NONE',  ( 85.00000000000029843, 17.00000000000000000, -60.00000000000000000 ) ) ;
#8997=LINE ( 'NONE', #24653, #41452 ) ;
#9000=ORIENTED_EDGE ( 'NONE', *, *, #32402, .T. ) ;
#9010=EDGE_CURVE ( 'NONE', #13545, #6749, #15351, .T. ) ;
#9013=CARTESIAN_POINT ( 'NONE',  ( 35.00000000000122213, 16.00000000000000000, 5.000000000000004441 ) ) ;
#9026=VECTOR ( 'NONE', #32442, 1000.000000000000000 ) ;
#9030=DIRECTION ( 'NONE',  ( -0.000000000000000000, -1.000000000000000000, -0.000000000000000000 ) ) ;
#9048=ORIENTED_EDGE ( 'NONE', *, *, #38680, .T. ) ;
#9049=CARTESIAN_POINT ( 'NONE',  ( 130.0000000000015064, 17.00000000000000000, 35.00000000000000000 ) ) ;
#9054=DIRECTION ( 'NONE',  ( -0.000000000000000000, -1.000000000000000000, -0.000000000000000000 ) ) ;
#9057=ORIENTED_EDGE ( 'NONE', *, *, #4527, .T. ) ;
#9061=CARTESIAN_POINT ( 'NONE',  ( 135.0000000000000000, 16.00000000000000000, -114.9999999999999858 ) ) ;
#9066=DIRECTION ( 'NONE',  ( -0.000000000000000000, -1.000000000000000000, -0.000000000000000000 ) ) ;
#9070=FACE_OUTER_BOUND ( 'NONE', #42932, .T. ) ;
#9076=DIRECTION ( 'NONE',  ( 0.000000000000000000, 0.000000000000000000, 1.000000000000000000 ) ) ;
#9082=FACE_OUTER_BOUND ( 'NONE', #42973, .T. ) ;
#9083=VERTEX_POINT ( 'NONE', #22780 ) ;
#9086=VERTEX_POINT ( 'NONE', #34340 ) ;
#9091=DIRECTION ( 'NONE',  ( 1.000000000000000000, 0.000000000000000000, -0.000000000000000000 ) ) ;
#9101=AXIS2_PLACEMENT_3D ( 'NONE', #48542, #21637, #16788 ) ;
#9105=DIRECTION ( 'NONE',  ( -0.000000000000000000, -1.000000000000000000, -0.000000000000000000 ) ) ;
#9108=ORIENTED_EDGE ( 'NONE', *, *, #3916, .F. ) ;
#9116=ORIENTED_EDGE ( 'NONE', *, *, #17628, .F. ) ;
#9121=CARTESIAN_POINT ( 'NONE',  ( 130.0000000000015064, 17.00000000000000000, 60.00000000000000000 ) ) ;
#9128=CARTESIAN_POINT ( 'NONE',  ( 130.0000000000005684, 17.00000000000000000, -54.99999999999999289 ) ) ;
#9168=ORIENTED_EDGE ( 'NONE', *, *, #35375, .T. ) ;
#9169=DIRECTION ( 'NONE',  ( 1.000000000000000000, 0.000000000000000000, -0.000000000000000000 ) ) ;
#9171=LINE ( 'NONE', #48125, #31594 ) ;
#9175=CARTESIAN_POINT ( 'NONE',  ( 35.00000000000186162, 17.00000000000000000, 65.00000000000000000 ) ) ;
#9178=CARTESIAN_POINT ( 'NONE',  ( -175.0000000000000000, 0.000000000000000000, -122.5000000000000000 ) ) ;
#9183=CARTESIAN_POINT ( 'NONE',  ( 130.0000000000005684, 17.00000000000000000, -54.99999999999999289 ) ) ;
#9215=DIRECTION ( 'NONE',  ( -0.000000000000000000, -1.000000000000000000, -0.000000000000000000 ) ) ;
#9217=DIRECTION ( 'NONE',  ( 0.000000000000000000, 0.000000000000000000, 1.000000000000000000 ) ) ;
#9218=AXIS2_PLACEMENT_3D ( 'NONE', #3021, #26382, #46786 ) ;
#9225=LINE ( 'NONE', #17432, #32692 ) ;
#9228=EDGE_LOOP ( 'NONE', ( #40039, #10659, #18039, #29670 ) ) ;
#9232=CARTESIAN_POINT ( 'NONE',  ( -114.9999999999991047, 17.00000000000000000, -24.99999999999999289 ) ) ;
#9243=LINE ( 'NONE', #41555, #38767 ) ;
#9244=EDGE_CURVE ( 'NONE', #28645, #41417, #21683, .T. ) ;
#9251=EDGE_CURVE ( 'NONE', #43110, #12379, #46716, .T. ) ;
#9256=VERTEX_POINT ( 'NONE', #39331 ) ;
#9258=CARTESIAN_POINT ( 'NONE',  ( -69.99999999999909051, 16.00000000000000000, -24.99999999999999289 ) ) ;
#9263=VERTEX_POINT ( 'NONE', #23418 ) ;
#9272=DIRECTION ( 'NONE',  ( 0.000000000000000000, 0.000000000000000000, -1.000000000000000000 ) ) ;
#9274=ORIENTED_EDGE ( 'NONE', *, *, #24265, .F. ) ;
#9275=AXIS2_PLACEMENT_3D ( 'NONE', #14499, #49100, #23414 ) ;
#9280=LINE ( 'NONE', #29032, #16381 ) ;
#9285=ORIENTED_EDGE ( 'NONE', *, *, #16717, .F. ) ;
#9296=DIRECTION ( 'NONE',  ( -1.000000000000000000, 0.000000000000000000, -0.000000000000000000 ) ) ;
#9301=VECTOR ( 'NONE', #272, 1000.000000000000000 ) ;
#9317=EDGE_CURVE ( 'NONE', #31951, #34191, #15708, .T. ) ;
#9323=ADVANCED_FACE ( 'NONE', ( #22896 ), #34986, .F. ) ;
#9325=DIRECTION ( 'NONE',  ( 0.000000000000000000, 0.000000000000000000, -1.000000000000000000 ) ) ;
#9328=ADVANCED_FACE ( 'NONE', ( #15452 ), #15970, .F. ) ;
#9329=AXIS2_PLACEMENT_3D ( 'NONE', #47753, #23947, #5450 ) ;
#9330=LINE ( 'NONE', #24986, #29666 ) ;
#9333=CARTESIAN_POINT ( 'NONE',  ( -69.99999999999783995, 16.00000000000000000, 95.00000000000000000 ) ) ;
#9336=CARTESIAN_POINT ( 'NONE',  ( 130.0000000000005684, 16.00000000000000000, -54.99999999999999289 ) ) ;
#9339=EDGE_LOOP ( 'NONE', ( #36894, #6607, #27198, #40819 ) ) ;
#9342=DIRECTION ( 'NONE',  ( -0.000000000000000000, -1.000000000000000000, -0.000000000000000000 ) ) ;
#9357=VERTEX_POINT ( 'NONE', #8786 ) ;
#9359=EDGE_CURVE ( 'NONE', #22541, #156, #5669, .T. ) ;
#9360=LINE ( 'NONE', #25017, #25885 ) ;
#9362=EDGE_LOOP ( 'NONE', ( #32478, #49995, #34131, #9285 ) ) ;
#9368=CARTESIAN_POINT ( 'NONE',  ( -165.0000000000000284, 16.00000000000000000, 35.00000000000000000 ) ) ;
#9375=EDGE_CURVE ( 'NONE', #48546, #45606, #36243, .T. ) ;
#9377=ORIENTED_EDGE ( 'NONE', *, *, #50589, .T. ) ;
#9379=FACE_OUTER_BOUND ( 'NONE', #34440, .T. ) ;
#9383=VECTOR ( 'NONE', #27732, 1000.000000000000000 ) ;
#9384=ADVANCED_FACE ( 'NONE', ( #4913 ), #24685, .F. ) ;
#9387=FACE_OUTER_BOUND ( 'NONE', #15657, .T. ) ;
#9403=EDGE_LOOP ( 'NONE', ( #33604, #10684, #10255, #2026 ) ) ;
#9417=CARTESIAN_POINT ( 'NONE',  ( -165.0000000000000284, 16.00000000000000000, -114.9999999999999858 ) ) ;
#9418=ORIENTED_EDGE ( 'NONE', *, *, #35720, .T. ) ;
#9435=CARTESIAN_POINT ( 'NONE',  ( 135.0000000000006253, 17.00000000000000000, -54.99999999999999289 ) ) ;
#9440=ORIENTED_EDGE ( 'NONE', *, *, #9317, .F. ) ;
#9451=ORIENTED_EDGE ( 'NONE', *, *, #15000, .T. ) ;
#9457=ORIENTED_EDGE ( 'NONE', *, *, #6445, .T. ) ;
#9463=DIRECTION ( 'NONE',  ( -1.000000000000000000, -0.000000000000000000, -0.000000000000000000 ) ) ;
#9470=DIRECTION ( 'NONE',  ( -0.000000000000000000, -1.000000000000000000, -0.000000000000000000 ) ) ;
#9471=VERTEX_POINT ( 'NONE', #16720 ) ;
#9478=ORIENTED_EDGE ( 'NONE', *, *, #38074, .T. ) ;
#9484=VECTOR ( 'NONE', #15844, 1000.000000000000000 ) ;
#9498=LINE ( 'NONE', #24911, #24873 ) ;
#9506=LINE ( 'NONE', #29516, #20530 ) ;
#9509=ORIENTED_EDGE ( 'NONE', *, *, #32344, .T. ) ;
#9526=LINE ( 'NONE', #44651, #36089 ) ;
#9535=ADVANCED_FACE ( 'NONE', ( #22328 ), #45144, .F. ) ;
#9537=ORIENTED_EDGE ( 'NONE', *, *, #22357, .F. ) ;
#9554=VERTEX_POINT ( 'NONE', #17734 ) ;
#9556=EDGE_LOOP ( 'NONE', ( #8835, #40877, #36846, #48279 ) ) ;
#9562=ORIENTED_EDGE ( 'NONE', *, *, #17824, .T. ) ;
#9565=FACE_OUTER_BOUND ( 'NONE', #33287, .T. ) ;
#9575=EDGE_LOOP ( 'NONE', ( #14324, #31273, #38521, #14127 ) ) ;
#9581=ORIENTED_EDGE ( 'NONE', *, *, #47461, .T. ) ;
#9586=EDGE_CURVE ( 'NONE', #20951, #46680, #2088, .T. ) ;
#9606=DIRECTION ( 'NONE',  ( -0.000000000000000000, -1.000000000000000000, -0.000000000000000000 ) ) ;
#9616=ORIENTED_EDGE ( 'NONE', *, *, #19386, .F. ) ;
#9627=DIRECTION ( 'NONE',  ( -0.000000000000000000, -1.000000000000000000, -0.000000000000000000 ) ) ;
#9629=EDGE_CURVE ( 'NONE', #38277, #14475, #11742, .T. ) ;
#9645=VECTOR ( 'NONE', #8069, 1000.000000000000000 ) ;
#9648=DIRECTION ( 'NONE',  ( 0.000000000000000000, -0.000000000000000000, -1.000000000000000000 ) ) ;
#9663=EDGE_CURVE ( 'NONE', #13070, #42474, #47605, .T. ) ;
#9668=CARTESIAN_POINT ( 'NONE',  ( -165.0000000000000284, 16.00000000000000000, 60.00000000000000000 ) ) ;
#9671=ORIENTED_EDGE ( 'NONE', *, *, #5797, .T. ) ;
#9676=EDGE_CURVE ( 'NONE', #3789, #42829, #43534, .T. ) ;
#9700=DIRECTION ( 'NONE',  ( 0.000000000000000000, -0.000000000000000000, -1.000000000000000000 ) ) ;
#9704=CARTESIAN_POINT ( 'NONE',  ( 0.000000000000000000, 17.00000000000000000, 0.000000000000000000 ) ) ;
#9706=ORIENTED_EDGE ( 'NONE', *, *, #20839, .F. ) ;
#9707=FACE_OUTER_BOUND ( 'NONE', #42896, .T. ) ;
#9710=LINE ( 'NONE', #2023, #22167 ) ;
#9716=DIRECTION ( 'NONE',  ( -0.000000000000000000, -0.000000000000000000, -1.000000000000000000 ) ) ;
#9736=DIRECTION ( 'NONE',  ( 0.000000000000000000, 0.000000000000000000, 1.000000000000000000 ) ) ;
#9749=ORIENTED_EDGE ( 'NONE', *, *, #4856, .T. ) ;
#9757=PLANE ( 'NONE',  #17278 ) ;
#9759=AXIS2_PLACEMENT_3D ( 'NONE', #5418, #39843, #44645 ) ;
#9764=ORIENTED_EDGE ( 'NONE', *, *, #36140, .T. ) ;
#9776=CARTESIAN_POINT ( 'NONE',  ( 35.00000000000122213, 17.00000000000000000, 5.000000000000004441 ) ) ;
#9777=VECTOR ( 'NONE', #14437, 1000.000000000000000 ) ;
#9790=AXIS2_PLACEMENT_3D ( 'NONE', #50429, #23542, #15835 ) ;
#9797=EDGE_CURVE ( 'NONE', #30725, #6936, #36889, .T. ) ;
#9798=LINE ( 'NONE', #49004, #24935 ) ;
#9818=VECTOR ( 'NONE', #23089, 1000.000000000000000 ) ;
#9820=EDGE_CURVE ( 'NONE', #25937, #12379, #36640, .T. ) ;
#9827=AXIS2_PLACEMENT_3D ( 'NONE', #41542, #10492, #25646 ) ;
#9835=FACE_OUTER_BOUND ( 'NONE', #42939, .T. ) ;
#9843=CARTESIAN_POINT ( 'NONE',  ( -114.9999999999997158, 17.00000000000000000, -84.99999999999998579 ) ) ;
#9845=ORIENTED_EDGE ( 'NONE', *, *, #43751, .T. ) ;
#9853=ORIENTED_EDGE ( 'NONE', *, *, #11385, .T. ) ;
#9867=ORIENTED_EDGE ( 'NONE', *, *, #25812, .T. ) ;
#9883=EDGE_CURVE ( 'NONE', #11818, #3838, #38134, .T. ) ;
#9884=EDGE_CURVE ( 'NONE', #29962, #375, #14507, .T. ) ;
#9894=CARTESIAN_POINT ( 'NONE',  ( 164.9999999999999716, 17.00000000000000000, 90.00000000000000000 ) ) ;
#9895=VECTOR ( 'NONE', #44217, 1000.000000000000000 ) ;
#9900=VERTEX_POINT ( 'NONE', #10657 ) ;
#9902=VECTOR ( 'NONE', #38432, 1000.000000000000000 ) ;
#9909=ORIENTED_EDGE ( 'NONE', *, *, #7485, .T. ) ;
#9934=ADVANCED_FACE ( 'NONE', ( #18101 ), #37883, .F. ) ;
#9940=VECTOR ( 'NONE', #45585, 1000.000000000000000 ) ;
#9949=CARTESIAN_POINT ( 'NONE',  ( -175.0000000000000000, 15.00000000000000000, -122.5000000000000000 ) ) ;
#9950=LINE ( 'NONE', #2506, #4165 ) ;
#9953=ORIENTED_EDGE ( 'NONE', *, *, #46124, .F. ) ;
#9959=DIRECTION ( 'NONE',  ( 0.000000000000000000, -1.000000000000000000, 0.000000000000000000 ) ) ;
#9963=ORIENTED_EDGE ( 'NONE', *, *, #9586, .F. ) ;
#9977=DIRECTION ( 'NONE',  ( -1.000000000000000000, -0.000000000000000000, -0.000000000000000000 ) ) ;
#9983=LINE ( 'NONE', #49188, #7124 ) ;
#9988=FACE_OUTER_BOUND ( 'NONE', #8102, .T. ) ;
#9998=CARTESIAN_POINT ( 'NONE',  ( 30.00000000000153833, 16.00000000000000000, 60.00000000000000000 ) ) ;
#10007=ADVANCED_FACE ( 'NONE', ( #31443 ), #8092, .F. ) ;
#10020=ORIENTED_EDGE ( 'NONE', *, *, #35555, .T. ) ;
#10027=CARTESIAN_POINT ( 'NONE',  ( 35.00000000000028422, 17.00000000000000000, -60.00000000000000000 ) ) ;
#10029=LINE ( 'NONE', #5667, #319 ) ;
#10030=ORIENTED_EDGE ( 'NONE', *, *, #19397, .T. ) ;
#10037=CARTESIAN_POINT ( 'NONE',  ( -119.9999999999984652, 16.00000000000000000, 35.00000000000000000 ) ) ;
#10048=DIRECTION ( 'NONE',  ( 0.000000000000000000, 0.000000000000000000, 1.000000000000000000 ) ) ;
#10052=LINE ( 'NONE', #41352, #22714 ) ;
#10058=VERTEX_POINT ( 'NONE', #4736 ) ;
#10067=EDGE_LOOP ( 'NONE', ( #48538, #11928, #40802, #4409 ) ) ;
#10068=LINE ( 'NONE', #29318, #3182 ) ;
#10070=DIRECTION ( 'NONE',  ( 0.000000000000000000, 0.000000000000000000, 1.000000000000000000 ) ) ;
#10087=CARTESIAN_POINT ( 'NONE',  ( 0.000000000000000000, 17.00000000000000000, 0.000000000000000000 ) ) ;
#10100=ORIENTED_EDGE ( 'NONE', *, *, #3388, .F. ) ;
#10111=CARTESIAN_POINT ( 'NONE',  ( 0.000000000000000000, 17.00000000000000000, 0.000000000000000000 ) ) ;
#10124=DIRECTION ( 'NONE',  ( -0.000000000000000000, -1.000000000000000000, -0.000000000000000000 ) ) ;
#10129=ORIENTED_EDGE ( 'NONE', *, *, #48830, .T. ) ;
#10130=DIRECTION ( 'NONE',  ( 0.000000000000000000, -1.000000000000000000, 0.000000000000000000 ) ) ;
#10141=VECTOR ( 'NONE', #2173, 1000.000000000000000 ) ;
#10148=ORIENTED_EDGE ( 'NONE', *, *, #46335, .F. ) ;
#10158=DIRECTION ( 'NONE',  ( 0.000000000000000000, 0.000000000000000000, -1.000000000000000000 ) ) ;
#10173=ADVANCED_FACE ( 'NONE', ( #44966 ), #20889, .F. ) ;
#10177=CARTESIAN_POINT ( 'NONE',  ( -14.99999999999937472, 17.00000000000000000, -54.99999999999999289 ) ) ;
#10183=AXIS2_PLACEMENT_3D ( 'NONE', #40077, #39576, #43161 ) ;
#10189=LINE ( 'NONE', #49140, #18221 ) ;
#10192=DIRECTION ( 'NONE',  ( 1.000000000000000000, 0.000000000000000000, 0.000000000000000000 ) ) ;
#10194=DIRECTION ( 'NONE',  ( 0.000000000000000000, 0.000000000000000000, 1.000000000000000000 ) ) ;
#10202=EDGE_CURVE ( 'NONE', #38172, #17930, #11114, .T. ) ;
#10205=ORIENTED_EDGE ( 'NONE', *, *, #44178, .T. ) ;
#10222=VERTEX_POINT ( 'NONE', #37825 ) ;
#10228=ADVANCED_FACE ( 'NONE', ( #42146 ), #33464, .F. ) ;
#10229=DIRECTION ( 'NONE',  ( -1.000000000000000000, 0.000000000000000000, -0.000000000000000000 ) ) ;
#10230=CARTESIAN_POINT ( 'NONE',  ( 80.00000000000028422, 17.00000000000000000, -60.00000000000000000 ) ) ;
#10231=CARTESIAN_POINT ( 'NONE',  ( 135.0000000000012790, 17.00000000000000000, 5.000000000000004441 ) ) ;
#10242=ORIENTED_EDGE ( 'NONE', *, *, #20, .F. ) ;
#10253=FACE_BOUND ( 'NONE', #46200, .T. ) ;
#10255=ORIENTED_EDGE ( 'NONE', *, *, #45625, .F. ) ;
#10256=VECTOR ( 'NONE', #3796, 1000.000000000000000 ) ;
#10262=AXIS2_PLACEMENT_3D ( 'NONE', #18069, #19589, #7811 ) ;
#10276=ORIENTED_EDGE ( 'NONE', *, *, #43094, .T. ) ;
#10282=AXIS2_PLACEMENT_3D ( 'NONE', #14672, #47454, #31355 ) ;
#10296=EDGE_LOOP ( 'NONE', ( #20382, #26510, #27115, #33635 ) ) ;
#10300=EDGE_CURVE ( 'NONE', #21591, #49766, #29855, .T. ) ;
#10301=ORIENTED_EDGE ( 'NONE', *, *, #2670, .T. ) ;
#10309=EDGE_LOOP ( 'NONE', ( #41983, #38654, #5294, #13936 ) ) ;
#10318=VERTEX_POINT ( 'NONE', #41653 ) ;
#10322=EDGE_CURVE ( 'NONE', #30968, #15451, #14703, .T. ) ;
#10333=DIRECTION ( 'NONE',  ( 0.000000000000000000, 0.000000000000000000, 1.000000000000000000 ) ) ;
#10356=DIRECTION ( 'NONE',  ( -1.000000000000000000, -0.000000000000000000, -0.000000000000000000 ) ) ;
#10363=CARTESIAN_POINT ( 'NONE',  ( -119.9999999999984652, 17.00000000000000000, 35.00000000000000000 ) ) ;
#10373=VECTOR ( 'NONE', #41904, 1000.000000000000000 ) ;
#10375=FACE_OUTER_BOUND ( 'NONE', #48052, .T. ) ;
#10378=EDGE_CURVE ( 'NONE', #23064, #10490, #47490, .T. ) ;
#10379=DIRECTION ( 'NONE',  ( 0.000000000000000000, -0.000000000000000000, -1.000000000000000000 ) ) ;
#10387=DIRECTION ( 'NONE',  ( 0.000000000000000000, 0.000000000000000000, 1.000000000000000000 ) ) ;
#10388=LINE ( 'NONE', #29626, #40800 ) ;
#10389=CARTESIAN_POINT ( 'NONE',  ( -64.99999999999971578, 17.00000000000000000, -84.99999999999998579 ) ) ;
#10390=LINE ( 'NONE', #49582, #39376 ) ;
#10393=ORIENTED_EDGE ( 'NONE', *, *, #27794, .T. ) ;
#10402=CARTESIAN_POINT ( 'NONE',  ( -114.9999999999994031, 16.00000000000000000, -30.00000000000000000 ) ) ;
#10403=ADVANCED_FACE ( 'NONE', ( #15461 ), #39342, .F. ) ;
#10410=ORIENTED_EDGE ( 'NONE', *, *, #47146, .F. ) ;
#10412=DIRECTION ( 'NONE',  ( 1.000000000000000000, 0.000000000000000000, 0.000000000000000000 ) ) ;
#10417=LINE ( 'NONE', #21705, #48623 ) ;
#10425=ORIENTED_EDGE ( 'NONE', *, *, #2005, .T. ) ;
#10429=VERTEX_POINT ( 'NONE', #7787 ) ;
#10430=ORIENTED_EDGE ( 'NONE', *, *, #35603, .T. ) ;
#10443=PLANE ( 'NONE',  #44700 ) ;
#10451=CARTESIAN_POINT ( 'NONE',  ( -14.99999999999845812, 16.00000000000000000, 35.00000000000000000 ) ) ;
#10458=EDGE_CURVE ( 'NONE', #4352, #23493, #15979, .T. ) ;
#10469=ORIENTED_EDGE ( 'NONE', *, *, #23811, .F. ) ;
#10473=CARTESIAN_POINT ( 'NONE',  ( 85.00000000000152056, 16.00000000000000000, 60.00000000000000000 ) ) ;
#10486=EDGE_CURVE ( 'NONE', #30177, #6629, #24696, .T. ) ;
#10490=VERTEX_POINT ( 'NONE', #16988 ) ;
#10492=DIRECTION ( 'NONE',  ( 1.000000000000000000, 0.000000000000000000, 0.000000000000000000 ) ) ;
#10497=CARTESIAN_POINT ( 'NONE',  ( -119.9999999999978400, 17.00000000000000000, 115.0000000000000142 ) ) ;
#10499=FACE_BOUND ( 'NONE', #41012, .T. ) ;
#10503=DIRECTION ( 'NONE',  ( -0.000000000000000000, -1.000000000000000000, -0.000000000000000000 ) ) ;
#10522=CARTESIAN_POINT ( 'NONE',  ( 130.0000000000005684, 16.00000000000000000, -30.00000000000000000 ) ) ;
#10526=DIRECTION ( 'NONE',  ( -1.000000000000000000, -0.000000000000000000, -0.000000000000000000 ) ) ;
#10531=ORIENTED_EDGE ( 'NONE', *, *, #2428, .T. ) ;
#10548=AXIS2_PLACEMENT_3D ( 'NONE', #22190, #14218, #42428 ) ;
#10553=VERTEX_POINT ( 'NONE', #844 ) ;
#10554=LINE ( 'NONE', #49260, #26942 ) ;
#10560=VECTOR ( 'NONE', #24153, 1000.000000000000000 ) ;
#10564=VECTOR ( 'NONE', #46971, 1000.000000000000000 ) ;
#10569=FACE_OUTER_BOUND ( 'NONE', #33163, .T. ) ;
#10570=ORIENTED_EDGE ( 'NONE', *, *, #4439, .T. ) ;
#10576=ADVANCED_FACE ( 'NONE', ( #36002 ), #16488, .F. ) ;
#10580=CARTESIAN_POINT ( 'NONE',  ( -14.99999999999876366, 17.00000000000000000, 30.00000000000000000 ) ) ;
#10592=EDGE_LOOP ( 'NONE', ( #48221, #34760, #46414, #27155 ) ) ;
#10598=EDGE_CURVE ( 'NONE', #31678, #29962, #21853, .T. ) ;
#10605=DIRECTION ( 'NONE',  ( 0.000000000000000000, 0.000000000000000000, 1.000000000000000000 ) ) ;
#10611=CARTESIAN_POINT ( 'NONE',  ( -14.99999999999845812, 17.00000000000000000, 60.00000000000000000 ) ) ;
#10613=ORIENTED_EDGE ( 'NONE', *, *, #50050, .T. ) ;
#10620=VECTOR ( 'NONE', #34338, 1000.000000000000000 ) ;
#10628=DIRECTION ( 'NONE',  ( 1.000000000000000000, 0.000000000000000000, 0.000000000000000000 ) ) ;
#10629=CARTESIAN_POINT ( 'NONE',  ( -64.99999999999940314, 16.00000000000000000, -30.00000000000000000 ) ) ;
#10657=CARTESIAN_POINT ( 'NONE',  ( -119.9999999999984652, 16.00000000000000000, 60.00000000000000000 ) ) ;
#10658=AXIS2_PLACEMENT_3D ( 'NONE', #49484, #22577, #37258 ) ;
#10659=ORIENTED_EDGE ( 'NONE', *, *, #32652, .F. ) ;
#10661=AXIS2_PLACEMENT_3D ( 'NONE', #48829, #5522, #32996 ) ;
#10676=DIRECTION ( 'NONE',  ( 0.000000000000000000, 0.000000000000000000, -1.000000000000000000 ) ) ;
#10684=ORIENTED_EDGE ( 'NONE', *, *, #4927, .F. ) ;
#10686=PLANE ( 'NONE',  #24194 ) ;
#10700=VECTOR ( 'NONE', #31725, 1000.000000000000000 ) ;
#10710=DIRECTION ( 'NONE',  ( -0.000000000000000000, -1.000000000000000000, -0.000000000000000000 ) ) ;
#10711=FACE_OUTER_BOUND ( 'NONE', #47867, .T. ) ;
#10731=DIRECTION ( 'NONE',  ( 0.000000000000000000, 0.000000000000000000, 1.000000000000000000 ) ) ;
#10745=ADVANCED_FACE ( 'NONE', ( #33410 ), #50246, .F. ) ;
#10765=VECTOR ( 'NONE', #27173, 1000.000000000000000 ) ;
#10771=CARTESIAN_POINT ( 'NONE',  ( -15.00000000000001421, 16.00000000000000000, -90.00000000000000000 ) ) ;
#10779=EDGE_LOOP ( 'NONE', ( #11239, #17743, #38510, #35016 ) ) ;
#10783=EDGE_LOOP ( 'NONE', ( #27144, #17980, #25449, #21626 ) ) ;
#10793=EDGE_LOOP ( 'NONE', ( #7268, #42612, #25063, #15459 ) ) ;
#10827=CARTESIAN_POINT ( 'NONE',  ( -165.0000000000000284, 17.00000000000000000, -90.00000000000000000 ) ) ;
#10829=EDGE_CURVE ( 'NONE', #27666, #7870, #18988, .T. ) ;
#10843=FACE_OUTER_BOUND ( 'NONE', #23138, .T. ) ;
#10846=LINE ( 'NONE', #41137, #22909 ) ;
#10848=EDGE_CURVE ( 'NONE', #24997, #15604, #46916, .T. ) ;
#10851=CARTESIAN_POINT ( 'NONE',  ( 35.00000000000152767, 17.00000000000000000, 35.00000000000000000 ) ) ;
#10852=LINE ( 'NONE', #14704, #4191 ) ;
#10870=ORIENTED_EDGE ( 'NONE', *, *, #7959, .F. ) ;
#10878=VECTOR ( 'NONE', #13354, 1000.000000000000000 ) ;
#10879=EDGE_CURVE ( 'NONE', #23358, #3329, #40280, .T. ) ;
#10880=ORIENTED_EDGE ( 'NONE', *, *, #34146, .F. ) ;
#10883=LINE ( 'NONE', #30394, #5558 ) ;
#10884=FACE_OUTER_BOUND ( 'NONE', #27356, .T. ) ;
#10885=FACE_OUTER_BOUND ( 'NONE', #41197, .T. ) ;
#10898=DIRECTION ( 'NONE',  ( -0.000000000000000000, -0.000000000000000000, -1.000000000000000000 ) ) ;
#10909=VECTOR ( 'NONE', #45581, 1000.000000000000000 ) ;
#10915=DIRECTION ( 'NONE',  ( -0.000000000000000000, -1.000000000000000000, -0.000000000000000000 ) ) ;
#10917=PLANE ( 'NONE',  #16874 ) ;
#10922=CARTESIAN_POINT ( 'NONE',  ( -119.9999999999984652, 16.00000000000000000, 35.00000000000000000 ) ) ;
#10935=ADVANCED_FACE ( 'NONE', ( #13312 ), #16174, .F. ) ;
#10951=CARTESIAN_POINT ( 'NONE',  ( -14.99999999999782041, 16.00000000000000000, 115.0000000000000142 ) ) ;
#10960=DIRECTION ( 'NONE',  ( -0.000000000000000000, -1.000000000000000000, -0.000000000000000000 ) ) ;
#10961=VERTEX_POINT ( 'NONE', #10231 ) ;
#10964=DIRECTION ( 'NONE',  ( -1.000000000000000000, 0.000000000000000000, 0.000000000000000000 ) ) ;
#10971=ADVANCED_FACE ( 'NONE', ( #25380 ), #37211, .F. ) ;
#10978=EDGE_LOOP ( 'NONE', ( #43092, #33177, #43985, #35389 ) ) ;
#10982=AXIS2_PLACEMENT_3D ( 'NONE', #19940, #12493, #20704 ) ;
#10984=AXIS2_PLACEMENT_3D ( 'NONE', #39080, #19539, #16473 ) ;
#10991=DIRECTION ( 'NONE',  ( 0.000000000000000000, -0.000000000000000000, -1.000000000000000000 ) ) ;
#10996=EDGE_LOOP ( 'NONE', ( #26411, #42940, #12290, #33205 ) ) ;
#11010=ADVANCED_FACE ( 'NONE', ( #13807 ), #49179, .F. ) ;
#11011=CARTESIAN_POINT ( 'NONE',  ( 35.00000000000061107, 16.00000000000000000, -54.99999999999999289 ) ) ;
#11014=DIRECTION ( 'NONE',  ( -0.000000000000000000, -1.000000000000000000, -0.000000000000000000 ) ) ;
#11015=AXIS2_PLACEMENT_3D ( 'NONE', #49056, #10605, #26269 ) ;
#11016=DIRECTION ( 'NONE',  ( -0.000000000000000000, -1.000000000000000000, -0.000000000000000000 ) ) ;
#11021=LINE ( 'NONE', #15387, #798 ) ;
#11026=DIRECTION ( 'NONE',  ( 0.000000000000000000, 0.000000000000000000, 1.000000000000000000 ) ) ;
#11032=VERTEX_POINT ( 'NONE', #26383 ) ;
#11033=CARTESIAN_POINT ( 'NONE',  ( 135.0000000000006253, 16.00000000000000000, -54.99999999999999289 ) ) ;
#11044=VERTEX_POINT ( 'NONE', #48922 ) ;
#11046=LINE ( 'NONE', #11303, #20158 ) ;
#11060=PLANE ( 'NONE',  #515 ) ;
#11062=DIRECTION ( 'NONE',  ( -1.000000000000000000, 0.000000000000000000, 0.000000000000000000 ) ) ;
#11064=ORIENTED_EDGE ( 'NONE', *, *, #45295, .T. ) ;
#11065=CARTESIAN_POINT ( 'NONE',  ( 85.00000000000056843, 16.00000000000000000, -54.99999999999999289 ) ) ;
#11068=LINE ( 'NONE', #42362, #33818 ) ;
#11078=CARTESIAN_POINT ( 'NONE',  ( 130.0000000000005684, 16.00000000000000000, -54.99999999999999289 ) ) ;
#11080=VECTOR ( 'NONE', #25108, 1000.000000000000000 ) ;
#11081=DIRECTION ( 'NONE',  ( 1.000000000000000000, 0.000000000000000000, 0.000000000000000000 ) ) ;
#11082=EDGE_LOOP ( 'NONE', ( #6284, #44033, #17687, #3361 ) ) ;
#11090=ORIENTED_EDGE ( 'NONE', *, *, #9820, .T. ) ;
#11106=VERTEX_POINT ( 'NONE', #12007 ) ;
#11111=EDGE_CURVE ( 'NONE', #48546, #1481, #43289, .T. ) ;
#11112=ORIENTED_EDGE ( 'NONE', *, *, #35984, .F. ) ;
#11114=LINE ( 'NONE', #49551, #8702 ) ;
#11116=ORIENTED_EDGE ( 'NONE', *, *, #12043, .T. ) ;
#11123=DIRECTION ( 'NONE',  ( -0.000000000000000000, -1.000000000000000000, -0.000000000000000000 ) ) ;
#11127=ADVANCED_FACE ( 'NONE', ( #30485 ), #18670, .F. ) ;
#11128=DIRECTION ( 'NONE',  ( -0.000000000000000000, -1.000000000000000000, -0.000000000000000000 ) ) ;
#11129=LINE ( 'NONE', #6767, #36210 ) ;
#11143=AXIS2_PLACEMENT_3D ( 'NONE', #31989, #47831, #47584 ) ;
#11149=DIRECTION ( 'NONE',  ( 0.000000000000000000, -0.000000000000000000, 1.000000000000000000 ) ) ;
#11151=DIRECTION ( 'NONE',  ( -0.000000000000000000, -0.000000000000000000, -1.000000000000000000 ) ) ;
#11159=VECTOR ( 'NONE', #9215, 1000.000000000000000 ) ;
#11160=CARTESIAN_POINT ( 'NONE',  ( 35.00000000000091660, 17.00000000000000000, 0.000000000000000000 ) ) ;
#11176=CARTESIAN_POINT ( 'NONE',  ( 130.0000000000008811, 16.00000000000000000, -24.99999999999999289 ) ) ;
#11177=EDGE_CURVE ( 'NONE', #21648, #45351, #50445, .T. ) ;
#11182=EDGE_CURVE ( 'NONE', #25320, #16028, #31262, .T. ) ;
#11186=ORIENTED_EDGE ( 'NONE', *, *, #4728, .F. ) ;
#11200=LINE ( 'NONE', #34289, #7348 ) ;
#11239=ORIENTED_EDGE ( 'NONE', *, *, #9359, .T. ) ;
#11252=EDGE_LOOP ( 'NONE', ( #4720, #30211, #30486, #9451 ) ) ;
#11253=CARTESIAN_POINT ( 'NONE',  ( 135.0000000000021600, 17.00000000000000000, 115.0000000000000142 ) ) ;
#11260=ORIENTED_EDGE ( 'NONE', *, *, #44982, .T. ) ;
#11261=DIRECTION ( 'NONE',  ( -1.000000000000000000, 0.000000000000000000, 4.625929269271542120E-16 ) ) ;
#11262=DIRECTION ( 'NONE',  ( -0.000000000000000000, -1.000000000000000000, -0.000000000000000000 ) ) ;
#11275=ORIENTED_EDGE ( 'NONE', *, *, #37546, .T. ) ;
#11285=CARTESIAN_POINT ( 'NONE',  ( -114.9999999999991047, 17.00000000000000000, 0.000000000000000000 ) ) ;
#11296=ADVANCED_FACE ( 'NONE', ( #36126 ), #44285, .F. ) ;
#11301=ORIENTED_EDGE ( 'NONE', *, *, #27508, .F. ) ;
#11303=CARTESIAN_POINT ( 'NONE',  ( -14.99999999999845812, 17.00000000000000000, 35.00000000000000000 ) ) ;
#11311=DIRECTION ( 'NONE',  ( 0.000000000000000000, 0.000000000000000000, 1.000000000000000000 ) ) ;
#11326=ORIENTED_EDGE ( 'NONE', *, *, #3052, .T. ) ;
#11327=ADVANCED_FACE ( 'NONE', ( #32020 ), #4555, .F. ) ;
#11334=VECTOR ( 'NONE', #7884, 1000.000000000000000 ) ;
#11346=ORIENTED_EDGE ( 'NONE', *, *, #49970, .F. ) ;
#11350=EDGE_LOOP ( 'NONE', ( #15039, #25372, #21533, #27221 ) ) ;
#11362=VECTOR ( 'NONE', #23716, 1000.000000000000000 ) ;
#11372=LINE ( 'NONE', #23441, #50026 ) ;
#11375=ADVANCED_FACE ( 'NONE', ( #4791 ), #30118, .F. ) ;
#11377=ORIENTED_EDGE ( 'NONE', *, *, #49483, .F. ) ;
#11383=ORIENTED_EDGE ( 'NONE', *, *, #2412, .T. ) ;
#11385=EDGE_CURVE ( 'NONE', #38545, #3838, #6760, .T. ) ;
#11386=EDGE_CURVE ( 'NONE', #49071, #42092, #15232, .T. ) ;
#11387=VERTEX_POINT ( 'NONE', #29864 ) ;
#11394=ADVANCED_FACE ( 'NONE', ( #22408 ), #45478, .F. ) ;
#11413=VECTOR ( 'NONE', #1336, 1000.000000000000000 ) ;
#11414=EDGE_CURVE ( 'NONE', #48563, #17047, #50317, .T. ) ;
#11415=EDGE_CURVE ( 'NONE', #29419, #9900, #38339, .T. ) ;
#11418=CARTESIAN_POINT ( 'NONE',  ( 135.0000000000009663, 16.00000000000000000, -24.99999999999999289 ) ) ;
#11438=ORIENTED_EDGE ( 'NONE', *, *, #27102, .T. ) ;
#11449=EDGE_CURVE ( 'NONE', #14316, #31951, #14463, .T. ) ;
#11450=ORIENTED_EDGE ( 'NONE', *, *, #35715, .T. ) ;
#11452=VECTOR ( 'NONE', #31498, 1000.000000000000000 ) ;
#11456=DIRECTION ( 'NONE',  ( 1.000000000000000000, 0.000000000000000000, 0.000000000000000000 ) ) ;
#11461=CARTESIAN_POINT ( 'NONE',  ( 135.0000000000012790, 16.00000000000000000, 30.00000000000000000 ) ) ;
#11470=LINE ( 'NONE', #11724, #45110 ) ;
#11478=FACE_OUTER_BOUND ( 'NONE', #7099, .T. ) ;
#11481=AXIS2_PLACEMENT_3D ( 'NONE', #41984, #49635, #14526 ) ;
#11485=ORIENTED_EDGE ( 'NONE', *, *, #25235, .T. ) ;
#11489=ORIENTED_EDGE ( 'NONE', *, *, #32741, .F. ) ;
#11491=VECTOR ( 'NONE', #8474, 1000.000000000000000 ) ;
#11493=LINE ( 'NONE', #3517, #46668 ) ;
#11500=CARTESIAN_POINT ( 'NONE',  ( -115.0000000000000284, 16.00000000000000000, -114.9999999999999858 ) ) ;
#11507=EDGE_CURVE ( 'NONE', #10961, #40535, #27021, .T. ) ;
#11508=VERTEX_POINT ( 'NONE', #20336 ) ;
#11510=CARTESIAN_POINT ( 'NONE',  ( 135.0000000000006253, 17.00000000000000000, -30.00000000000000000 ) ) ;
#11516=CARTESIAN_POINT ( 'NONE',  ( 0.000000000000000000, 17.00000000000000000, 0.000000000000000000 ) ) ;
#11517=ADVANCED_FACE ( 'NONE', ( #46987 ), #23437, .F. ) ;
#11520=CARTESIAN_POINT ( 'NONE',  ( -64.99999999999909051, 16.00000000000000000, 0.000000000000000000 ) ) ;
#11522=LINE ( 'NONE', #45865, #35701 ) ;
#11525=VECTOR ( 'NONE', #30702, 1000.000000000000000 ) ;
#11535=DIRECTION ( 'NONE',  ( -1.000000000000000000, 0.000000000000000000, 4.625929269271635797E-16 ) ) ;
#11546=DIRECTION ( 'NONE',  ( -1.000000000000000000, -0.000000000000000000, -0.000000000000000000 ) ) ;
#11560=ORIENTED_EDGE ( 'NONE', *, *, #10598, .T. ) ;
#11565=VECTOR ( 'NONE', #39949, 1000.000000000000000 ) ;
#11566=DIRECTION ( 'NONE',  ( -1.000000000000000000, -0.000000000000000000, -0.000000000000000000 ) ) ;
#11570=CARTESIAN_POINT ( 'NONE',  ( 164.9999999999999716, 17.00000000000000000, 59.99999999999999289 ) ) ;
#11575=ORIENTED_EDGE ( 'NONE', *, *, #21603, .T. ) ;
#11577=CARTESIAN_POINT ( 'NONE',  ( 130.0000000000008811, 16.00000000000000000, 0.000000000000000000 ) ) ;
#11582=ORIENTED_EDGE ( 'NONE', *, *, #12792, .F. ) ;
#11586=DIRECTION ( 'NONE',  ( 1.000000000000000000, 0.000000000000000000, 0.000000000000000000 ) ) ;
#11591=EDGE_CURVE ( 'NONE', #5571, #19596, #17248, .T. ) ;
#11595=CARTESIAN_POINT ( 'NONE',  ( 0.000000000000000000, 17.00000000000000000, 0.000000000000000000 ) ) ;
#11609=ORIENTED_EDGE ( 'NONE', *, *, #21739, .F. ) ;
#11614=DIRECTION ( 'NONE',  ( -0.000000000000000000, -1.000000000000000000, -0.000000000000000000 ) ) ;
#11624=DIRECTION ( 'NONE',  ( -1.000000000000000000, 0.000000000000000000, -0.000000000000000000 ) ) ;
#11627=ORIENTED_EDGE ( 'NONE', *, *, #11716, .F. ) ;
#11631=CARTESIAN_POINT ( 'NONE',  ( -119.9999999999981668, 17.00000000000000000, 65.00000000000000000 ) ) ;
#11635=FACE_OUTER_BOUND ( 'NONE', #3093, .T. ) ;
#11638=DIRECTION ( 'NONE',  ( 0.000000000000000000, 0.000000000000000000, 1.000000000000000000 ) ) ;
#11641=ORIENTED_EDGE ( 'NONE', *, *, #34464, .T. ) ;
#11656=ORIENTED_EDGE ( 'NONE', *, *, #27730, .T. ) ;
#11674=ORIENTED_EDGE ( 'NONE', *, *, #41643, .T. ) ;
#11684=VERTEX_POINT ( 'NONE', #36262 ) ;
#11716=EDGE_CURVE ( 'NONE', #950, #42829, #25450, .T. ) ;
#11718=EDGE_CURVE ( 'NONE', #26763, #38804, #32147, .T. ) ;
#11721=VECTOR ( 'NONE', #243, 1000.000000000000000 ) ;
#11724=CARTESIAN_POINT ( 'NONE',  ( -64.99999999999909051, 17.00000000000000000, 0.000000000000000000 ) ) ;
#11728=VECTOR ( 'NONE', #17334, 1000.000000000000000 ) ;
#11742=LINE ( 'NONE', #39461, #25908 ) ;
#11767=LINE ( 'NONE', #50195, #28287 ) ;
#11768=FACE_OUTER_BOUND ( 'NONE', #13353, .T. ) ;
#11769=DIRECTION ( 'NONE',  ( 0.000000000000000000, -0.000000000000000000, -1.000000000000000000 ) ) ;
#11772=EDGE_CURVE ( 'NONE', #22529, #8610, #2586, .T. ) ;
#11777=CARTESIAN_POINT ( 'NONE',  ( -164.9999999999994031, 17.00000000000000000, -30.00000000000000000 ) ) ;
#11791=LINE ( 'NONE', #11285, #11931 ) ;
#11796=CARTESIAN_POINT ( 'NONE',  ( 80.00000000000216005, 16.00000000000000000, 95.00000000000000000 ) ) ;
#11802=CARTESIAN_POINT ( 'NONE',  ( -19.99999999999908695, 17.00000000000000000, -24.99999999999999289 ) ) ;
#11806=VERTEX_POINT ( 'NONE', #49504 ) ;
#11818=VERTEX_POINT ( 'NONE', #6206 ) ;
#11820=DIRECTION ( 'NONE',  ( 0.000000000000000000, 0.000000000000000000, -1.000000000000000000 ) ) ;
#11828=DIRECTION ( 'NONE',  ( 0.000000000000000000, -1.000000000000000000, 0.000000000000000000 ) ) ;
#11830=ORIENTED_EDGE ( 'NONE', *, *, #38137, .T. ) ;
#11838=DIRECTION ( 'NONE',  ( -1.000000000000000000, -0.000000000000000000, -0.000000000000000000 ) ) ;
#11847=CARTESIAN_POINT ( 'NONE',  ( 85.00000000000029843, 17.00000000000000000, -84.99999999999998579 ) ) ;
#11848=CARTESIAN_POINT ( 'NONE',  ( -64.99999999999877787, 16.00000000000000000, 5.000000000000004441 ) ) ;
#11864=CARTESIAN_POINT ( 'NONE',  ( 80.00000000000122213, 16.00000000000000000, 30.00000000000000000 ) ) ;
#11866=ADVANCED_FACE ( 'NONE', ( #25966 ), #29543, .F. ) ;
#11867=CARTESIAN_POINT ( 'NONE',  ( 0.000000000000000000, 17.00000000000000000, 0.000000000000000000 ) ) ;
#11870=VERTEX_POINT ( 'NONE', #49246 ) ;
#11873=CARTESIAN_POINT ( 'NONE',  ( -165.0000000000000284, 16.00000000000000000, -114.9999999999999858 ) ) ;
#11892=CARTESIAN_POINT ( 'NONE',  ( -114.9999999999997158, 17.00000000000000000, -84.99999999999998579 ) ) ;
#11894=VECTOR ( 'NONE', #47851, 1000.000000000000000 ) ;
#11903=CARTESIAN_POINT ( 'NONE',  ( -14.99999999999782041, 17.00000000000000000, 95.00000000000000000 ) ) ;
#11907=DIRECTION ( 'NONE',  ( 0.000000000000000000, -1.000000000000000000, 0.000000000000000000 ) ) ;
#11912=VECTOR ( 'NONE', #4793, 1000.000000000000000 ) ;
#11918=PRODUCT_DEFINITION_FORMATION_WITH_SPECIFIED_SOURCE ( 'ANY', '', #49848, .NOT_KNOWN. ) ;
#11919=PLANE ( 'NONE',  #40061 ) ;
#11921=VECTOR ( 'NONE', #29560, 1000.000000000000000 ) ;
#11922=EDGE_CURVE ( 'NONE', #39269, #13970, #35445, .T. ) ;
#11928=ORIENTED_EDGE ( 'NONE', *, *, #6175, .F. ) ;
#11929=AXIS2_PLACEMENT_3D ( 'NONE', #15714, #46977, #43172 ) ;
#11931=VECTOR ( 'NONE', #42567, 1000.000000000000000 ) ;
#11935=VECTOR ( 'NONE', #10333, 1000.000000000000000 ) ;
#11936=ORIENTED_EDGE ( 'NONE', *, *, #33042, .F. ) ;
#11954=VECTOR ( 'NONE', #19664, 1000.000000000000000 ) ;
#11960=ORIENTED_EDGE ( 'NONE', *, *, #25215, .F. ) ;
#11964=DIRECTION ( 'NONE',  ( 0.000000000000000000, 0.000000000000000000, 1.000000000000000000 ) ) ;
#11969=ORIENTED_EDGE ( 'NONE', *, *, #9883, .T. ) ;
#11970=VECTOR ( 'NONE', #3852, 1000.000000000000000 ) ;
#11973=CARTESIAN_POINT ( 'NONE',  ( -64.99999999999783995, 17.00000000000000000, 115.0000000000000142 ) ) ;
#11979=ADVANCED_FACE ( 'NONE', ( #7983 ), #43358, .F. ) ;
#11989=CARTESIAN_POINT ( 'NONE',  ( -69.99999999999847944, 17.00000000000000000, 35.00000000000000000 ) ) ;
#11990=ORIENTED_EDGE ( 'NONE', *, *, #41822, .F. ) ;
#12007=CARTESIAN_POINT ( 'NONE',  ( -19.99999999999971223, 16.00000000000000000, -60.00000000000000000 ) ) ;
#12016=ORIENTED_EDGE ( 'NONE', *, *, #42133, .T. ) ;
#12021=ADVANCED_FACE ( 'NONE', ( #34943 ), #42851, .F. ) ;
#12022=ADVANCED_FACE ( 'NONE', ( #27975 ), #12317, .F. ) ;
#12034=FACE_OUTER_BOUND ( 'NONE', #25325, .T. ) ;
#12043=EDGE_CURVE ( 'NONE', #29675, #32627, #4634, .T. ) ;
#12045=ORIENTED_EDGE ( 'NONE', *, *, #35975, .T. ) ;
#12061=VECTOR ( 'NONE', #31135, 1000.000000000000000 ) ;
#12070=EDGE_CURVE ( 'NONE', #1878, #20271, #28237, .T. ) ;
#12101=EDGE_CURVE ( 'NONE', #2507, #36127, #44361, .T. ) ;
#12106=DIRECTION ( 'NONE',  ( -1.000000000000000000, -0.000000000000000000, -0.000000000000000000 ) ) ;
#12115=ORIENTED_EDGE ( 'NONE', *, *, #36525, .T. ) ;
#12126=ORIENTED_EDGE ( 'NONE', *, *, #39396, .T. ) ;
#12137=CARTESIAN_POINT ( 'NONE',  ( 135.0000000000019043, 17.00000000000000000, 90.00000000000000000 ) ) ;
#12142=ADVANCED_FACE ( 'NONE', ( #13324 ), #40043, .F. ) ;
#12148=ORIENTED_EDGE ( 'NONE', *, *, #6126, .F. ) ;
#12152=ORIENTED_EDGE ( 'NONE', *, *, #20330, .T. ) ;
#12158=EDGE_CURVE ( 'NONE', #45326, #15741, #44109, .T. ) ;
#12160=PLANE ( 'NONE',  #4536 ) ;
#12168=LINE ( 'NONE', #16525, #49800 ) ;
#12173=DIRECTION ( 'NONE',  ( 0.000000000000000000, 0.000000000000000000, 1.000000000000000000 ) ) ;
#12179=AXIS2_PLACEMENT_3D ( 'NONE', #32431, #4722, #9325 ) ;
#12184=ORIENTED_EDGE ( 'NONE', *, *, #2827, .F. ) ;
#12197=ADVANCED_FACE ( 'NONE', ( #9988 ), #45616, .F. ) ;
#12218=VECTOR ( 'NONE', #20453, 1000.000000000000000 ) ;
#12225=EDGE_CURVE ( 'NONE', #17811, #31254, #41285, .T. ) ;
#12233=PLANE ( 'NONE',  #3413 ) ;
#12238=ORIENTED_EDGE ( 'NONE', *, *, #27587, .F. ) ;
#12245=CARTESIAN_POINT ( 'NONE',  ( -164.9999999999978400, 17.00000000000000000, 95.00000000000000000 ) ) ;
#12249=AXIS2_PLACEMENT_3D ( 'NONE', #29207, #45577, #37427 ) ;
#12250=DIRECTION ( 'NONE',  ( -1.000000000000000000, 0.000000000000000000, 0.000000000000000000 ) ) ;
#12251=ORIENTED_EDGE ( 'NONE', *, *, #27728, .T. ) ;
#12279=AXIS2_PLACEMENT_3D ( 'NONE', #37871, #2689, #18834 ) ;
#12283=EDGE_CURVE ( 'NONE', #10058, #2811, #30498, .T. ) ;
#12286=CARTESIAN_POINT ( 'NONE',  ( 35.00000000000028422, 16.00000000000000000, -60.00000000000000000 ) ) ;
#12290=ORIENTED_EDGE ( 'NONE', *, *, #15348, .T. ) ;
#12296=PLANE ( 'NONE',  #20275 ) ;
#12299=ORIENTED_EDGE ( 'NONE', *, *, #42129, .F. ) ;
#12300=EDGE_CURVE ( 'NONE', #45326, #47156, #17922, .T. ) ;
#12302=LINE ( 'NONE', #39270, #9818 ) ;
#12309=DIRECTION ( 'NONE',  ( -1.000000000000000000, 0.000000000000000000, 0.000000000000000000 ) ) ;
#12317=PLANE ( 'NONE',  #25403 ) ;
#12327=FACE_OUTER_BOUND ( 'NONE', #19410, .T. ) ;
#12334=DIRECTION ( 'NONE',  ( 0.000000000000000000, -1.000000000000000000, 0.000000000000000000 ) ) ;
#12343=EDGE_CURVE ( 'NONE', #11870, #15720, #29741, .T. ) ;
#12346=EDGE_CURVE ( 'NONE', #10429, #9357, #34608, .T. ) ;
#12359=CARTESIAN_POINT ( 'NONE',  ( -164.9999999999997442, 17.00000000000000000, -84.99999999999998579 ) ) ;
#12361=CARTESIAN_POINT ( 'NONE',  ( 130.0000000000002842, 17.00000000000000000, -84.99999999999998579 ) ) ;
#12362=CARTESIAN_POINT ( 'NONE',  ( 0.000000000000000000, 17.00000000000000000, 0.000000000000000000 ) ) ;
#12368=EDGE_LOOP ( 'NONE', ( #22173, #12497, #28307, #9749 ) ) ;
#12369=DIRECTION ( 'NONE',  ( -0.000000000000000000, -1.000000000000000000, -0.000000000000000000 ) ) ;
#12379=VERTEX_POINT ( 'NONE', #23042 ) ;
#12381=EDGE_CURVE ( 'NONE', #31274, #33538, #27414, .T. ) ;
#12383=EDGE_CURVE ( 'NONE', #3452, #48040, #46372, .T. ) ;
#12395=CARTESIAN_POINT ( 'NONE',  ( -64.99999999999909051, 16.00000000000000000, 0.000000000000000000 ) ) ;
#12398=ADVANCED_FACE ( 'NONE', ( #16120 ), #31782, .F. ) ;
#12404=EDGE_CURVE ( 'NONE', #3395, #38611, #34876, .T. ) ;
#12410=ORIENTED_EDGE ( 'NONE', *, *, #25559, .F. ) ;
#12416=EDGE_CURVE ( 'NONE', #29858, #24991, #43045, .T. ) ;
#12422=EDGE_CURVE ( 'NONE', #19097, #36058, #8174, .T. ) ;
#12424=DIRECTION ( 'NONE',  ( -1.000000000000000000, -0.000000000000000000, -0.000000000000000000 ) ) ;
#12426=VECTOR ( 'NONE', #40326, 1000.000000000000000 ) ;
#12444=ADVANCED_FACE ( 'NONE', ( #717 ), #16882, .F. ) ;
#12452=EDGE_CURVE ( 'NONE', #40254, #18731, #48376, .T. ) ;
#12454=EDGE_LOOP ( 'NONE', ( #17852, #42109, #8344, #22731, #8116, #20496, #46844, #34906, #23353, #20313, #43168, #46319, #48181, #1556, #24225, #17226, #23759, #41035, #20881, #16617, #13935, #6497, #12702, #34280, #37590, #15750, #46140, #31955, #12299, #48739, #42613, #6651, #28917, #22318, #44828, #38839, #22701, #10276, #14521, #31019, #4451, #11090, #43779, #49192, #31180, #40832, #29123, #36862, #12503, #5567, #16105, #7706, #22, #3138, #26671, #821, #5044, #31666, #39116, #16987, #38437, #23083, #32235, #12148, #34602, #5096, #1535, #41394, #24261, #36271, #6130, #4098, #26274, #50703, #32838, #39845, #32013, #50280, #25222, #12757, #34326, #25269, #41020, #11969, #1067, #22562, #24205, #43283, #28722, #15172, #15760, #46144, #35887, #37881, #49491, #10020, #18849, #14403, #42324, #43488 ) ) ;
#12459=CARTESIAN_POINT ( 'NONE',  ( 0.000000000000000000, 17.00000000000000000, 0.000000000000000000 ) ) ;
#12468=DIRECTION ( 'NONE',  ( -1.000000000000000000, -0.000000000000000000, 9.251858538543084240E-16 ) ) ;
#12470=AXIS2_PLACEMENT_3D ( 'NONE', #2405, #18049, #6758 ) ;
#12472=DIRECTION ( 'NONE',  ( -0.000000000000000000, -1.000000000000000000, -0.000000000000000000 ) ) ;
#12477=ORIENTED_EDGE ( 'NONE', *, *, #28567, .T. ) ;
#12482=ORIENTED_EDGE ( 'NONE', *, *, #6786, .F. ) ;
#12485=ORIENTED_EDGE ( 'NONE', *, *, #14011, .T. ) ;
#12486=CARTESIAN_POINT ( 'NONE',  ( 135.0000000000015632, 17.00000000000000000, 35.00000000000000000 ) ) ;
#12489=EDGE_CURVE ( 'NONE', #39670, #31422, #981, .T. ) ;
#12491=VECTOR ( 'NONE', #45216, 1000.000000000000000 ) ;
#12493=DIRECTION ( 'NONE',  ( -1.000000000000000000, 0.000000000000000000, 0.000000000000000000 ) ) ;
#12497=ORIENTED_EDGE ( 'NONE', *, *, #48342, .F. ) ;
#12503=ORIENTED_EDGE ( 'NONE', *, *, #7771, .F. ) ;
#12504=CARTESIAN_POINT ( 'NONE',  ( 164.9999999999999716, 17.00000000000000000, 29.99999999999999289 ) ) ;
#12509=CARTESIAN_POINT ( 'NONE',  ( -69.99999999999972999, 17.00000000000000000, -84.99999999999998579 ) ) ;
#12512=FACE_OUTER_BOUND ( 'NONE', #6000, .T. ) ;
#12525=CARTESIAN_POINT ( 'NONE',  ( 0.000000000000000000, 17.00000000000000000, 0.000000000000000000 ) ) ;
#12548=ORIENTED_EDGE ( 'NONE', *, *, #4222, .T. ) ;
#12551=DIRECTION ( 'NONE',  ( -0.000000000000000000, -1.000000000000000000, -0.000000000000000000 ) ) ;
#12554=CARTESIAN_POINT ( 'NONE',  ( 80.00000000000153477, 17.00000000000000000, 35.00000000000000000 ) ) ;
#12561=CARTESIAN_POINT ( 'NONE',  ( 164.9999999999999716, 17.00000000000000000, -30.00000000000001421 ) ) ;
#12562=EDGE_LOOP ( 'NONE', ( #10430, #8768, #40903, #13453 ) ) ;
#12571=LINE ( 'NONE', #8492, #31691 ) ;
#12573=DIRECTION ( 'NONE',  ( 0.000000000000000000, 0.000000000000000000, -1.000000000000000000 ) ) ;
#12591=AXIS2_PLACEMENT_3D ( 'NONE', #40006, #47139, #47895 ) ;
#12597=AXIS2_PLACEMENT_3D ( 'NONE', #30783, #47137, #11535 ) ;
#12611=ORIENTED_EDGE ( 'NONE', *, *, #8634, .F. ) ;
#12612=CARTESIAN_POINT ( 'NONE',  ( 135.0000000000006253, 17.00000000000000000, -30.00000000000000000 ) ) ;
#12630=VECTOR ( 'NONE', #8238, 1000.000000000000000 ) ;
#12631=EDGE_CURVE ( 'NONE', #48700, #34291, #25836, .T. ) ;
#12633=EDGE_CURVE ( 'NONE', #45598, #15451, #6583, .T. ) ;
#12664=VECTOR ( 'NONE', #21781, 1000.000000000000000 ) ;
#12670=LINE ( 'NONE', #36561, #140 ) ;
#12675=DIRECTION ( 'NONE',  ( 0.000000000000000000, 0.000000000000000000, -1.000000000000000000 ) ) ;
#12685=ADVANCED_FACE ( 'NONE', ( #49134 ), #34050, .F. ) ;
#12686=EDGE_LOOP ( 'NONE', ( #4023, #47082, #29661, #22757 ) ) ;
#12702=ORIENTED_EDGE ( 'NONE', *, *, #49676, .T. ) ;
#12719=PLANE ( 'NONE',  #14395 ) ;
#12749=FACE_OUTER_BOUND ( 'NONE', #10978, .T. ) ;
#12752=DIRECTION ( 'NONE',  ( -1.000000000000000000, 0.000000000000000000, 2.312964634635864737E-16 ) ) ;
#12757=ORIENTED_EDGE ( 'NONE', *, *, #47146, .T. ) ;
#12760=CARTESIAN_POINT ( 'NONE',  ( 80.00000000000028422, 17.00000000000000000, -84.99999999999998579 ) ) ;
#12766=VECTOR ( 'NONE', #26582, 1000.000000000000000 ) ;
#12767=ORIENTED_EDGE ( 'NONE', *, *, #13290, .F. ) ;
#12783=LINE ( 'NONE', #5071, #30982 ) ;
#12788=EDGE_CURVE ( 'NONE', #36968, #47621, #30439, .T. ) ;
#12789=FACE_OUTER_BOUND ( 'NONE', #5217, .T. ) ;
#12792=EDGE_CURVE ( 'NONE', #49743, #11508, #162, .T. ) ;
#12797=EDGE_CURVE ( 'NONE', #48563, #34745, #34549, .T. ) ;
#12802=LINE ( 'NONE', #5086, #23752 ) ;
#12808=ORIENTED_EDGE ( 'NONE', *, *, #7538, .T. ) ;
#12820=CARTESIAN_POINT ( 'NONE',  ( -164.9999999999981526, 17.00000000000000000, 65.00000000000000000 ) ) ;
#12824=DIRECTION ( 'NONE',  ( 0.000000000000000000, -0.000000000000000000, -1.000000000000000000 ) ) ;
#12828=ORIENTED_EDGE ( 'NONE', *, *, #19528, .T. ) ;
#12834=CARTESIAN_POINT ( 'NONE',  ( -165.0000000000000284, 16.00000000000000000, 115.0000000000000142 ) ) ;
#12848=DIRECTION ( 'NONE',  ( -0.000000000000000000, -0.000000000000000000, -1.000000000000000000 ) ) ;
#12855=VECTOR ( 'NONE', #47612, 1000.000000000000000 ) ;
#12858=ORIENTED_EDGE ( 'NONE', *, *, #29293, .T. ) ;
#12864=FACE_OUTER_BOUND ( 'NONE', #18188, .T. ) ;
#12872=DIRECTION ( 'NONE',  ( 0.000000000000000000, 0.000000000000000000, 1.000000000000000000 ) ) ;
#12877=VERTEX_POINT ( 'NONE', #19894 ) ;
#12880=CARTESIAN_POINT ( 'NONE',  ( 164.9999999999999716, 16.00000000000000000, 115.0000000000000142 ) ) ;
#12887=FACE_OUTER_BOUND ( 'NONE', #26069, .T. ) ;
#12890=ORIENTED_EDGE ( 'NONE', *, *, #21435, .F. ) ;
#12894=DIRECTION ( 'NONE',  ( -0.000000000000000000, -1.000000000000000000, -0.000000000000000000 ) ) ;
#12900=CARTESIAN_POINT ( 'NONE',  ( 80.00000000000028422, 16.00000000000000000, -84.99999999999998579 ) ) ;
#12909=PLANE ( 'NONE',  #3964 ) ;
#12915=EDGE_CURVE ( 'NONE', #31020, #16052, #18084, .T. ) ;
#12921=CARTESIAN_POINT ( 'NONE',  ( -175.0000000000000000, 15.00000000000000000, -122.5000000000000000 ) ) ;
#12926=EDGE_LOOP ( 'NONE', ( #4407, #6903, #20738, #43199 ) ) ;
#12929=PLANE ( 'NONE',  #33718 ) ;
#12933=DIRECTION ( 'NONE',  ( 0.000000000000000000, -0.000000000000000000, -1.000000000000000000 ) ) ;
#12936=CARTESIAN_POINT ( 'NONE',  ( -14.99999999999970868, 17.00000000000000000, -60.00000000000000000 ) ) ;
#12948=ORIENTED_EDGE ( 'NONE', *, *, #37199, .F. ) ;
#12949=ORIENTED_EDGE ( 'NONE', *, *, #17043, .F. ) ;
#12952=EDGE_LOOP ( 'NONE', ( #32666, #35296, #31706, #24305 ) ) ;
#12954=LINE ( 'NONE', #36607, #17014 ) ;
#12960=DIRECTION ( 'NONE',  ( 0.000000000000000000, 0.000000000000000000, 1.000000000000000000 ) ) ;
#12972=LINE ( 'NONE', #44264, #11565 ) ;
#12984=VERTEX_POINT ( 'NONE', #17715 ) ;
#13003=VECTOR ( 'NONE', #35671, 1000.000000000000000 ) ;
#13010=AXIS2_PLACEMENT_3D ( 'NONE', #41538, #22537, #49937 ) ;
#13028=EDGE_CURVE ( 'NONE', #3789, #45615, #11021, .T. ) ;
#13038=EDGE_LOOP ( 'NONE', ( #40981, #22516, #12890, #13198 ) ) ;
#13048=FACE_OUTER_BOUND ( 'NONE', #9403, .T. ) ;
#13053=ORIENTED_EDGE ( 'NONE', *, *, #11772, .T. ) ;
#13056=LINE ( 'NONE', #44839, #8189 ) ;
#13063=ORIENTED_EDGE ( 'NONE', *, *, #48490, .F. ) ;
#13066=ORIENTED_EDGE ( 'NONE', *, *, #27810, .F. ) ;
#13068=DIRECTION ( 'NONE',  ( 0.000000000000000000, 0.000000000000000000, 1.000000000000000000 ) ) ;
#13070=VERTEX_POINT ( 'NONE', #42320 ) ;
#13077=AXIS2_PLACEMENT_3D ( 'NONE', #29724, #7139, #41524 ) ;
#13096=LINE ( 'NONE', #7294, #18295 ) ;
#13112=ORIENTED_EDGE ( 'NONE', *, *, #48424, .T. ) ;
#13137=DIRECTION ( 'NONE',  ( -0.000000000000000000, -0.000000000000000000, -1.000000000000000000 ) ) ;
#13141=FACE_OUTER_BOUND ( 'NONE', #37540, .T. ) ;
#13150=EDGE_CURVE ( 'NONE', #20047, #21591, #40504, .T. ) ;
#13155=LINE ( 'NONE', #28308, #26670 ) ;
#13158=( NAMED_UNIT ( * ) PLANE_ANGLE_UNIT ( ) SI_UNIT ( $, .RADIAN. ) );
#13159=PLANE ( 'NONE',  #19565 ) ;
#13161=DIRECTION ( 'NONE',  ( 0.000000000000000000, 0.000000000000000000, 1.000000000000000000 ) ) ;
#13173=ORIENTED_EDGE ( 'NONE', *, *, #38682, .F. ) ;
#13174=DIRECTION ( 'NONE',  ( -1.000000000000000000, 0.000000000000000000, -0.000000000000000000 ) ) ;
#13198=ORIENTED_EDGE ( 'NONE', *, *, #49346, .T. ) ;
#13202=PLANE ( 'NONE',  #48655 ) ;
#13207=CARTESIAN_POINT ( 'NONE',  ( -69.99999999999816680, 17.00000000000000000, 90.00000000000000000 ) ) ;
#13213=ORIENTED_EDGE ( 'NONE', *, *, #14692, .F. ) ;
#13233=FACE_OUTER_BOUND ( 'NONE', #20690, .T. ) ;
#13239=ORIENTED_EDGE ( 'NONE', *, *, #18370, .T. ) ;
#13241=DIRECTION ( 'NONE',  ( 0.000000000000000000, 0.000000000000000000, 1.000000000000000000 ) ) ;
#13246=ORIENTED_EDGE ( 'NONE', *, *, #49692, .T. ) ;
#13254=VECTOR ( 'NONE', #3634, 1000.000000000000000 ) ;
#13259=DIRECTION ( 'NONE',  ( -0.000000000000000000, -1.000000000000000000, -0.000000000000000000 ) ) ;
#13260=EDGE_CURVE ( 'NONE', #47621, #39178, #8199, .T. ) ;
#13261=CARTESIAN_POINT ( 'NONE',  ( -64.99999999999783995, 17.00000000000000000, 95.00000000000000000 ) ) ;
#13271=DIRECTION ( 'NONE',  ( 0.000000000000000000, 0.000000000000000000, 1.000000000000000000 ) ) ;
#13275=FACE_OUTER_BOUND ( 'NONE', #41252, .T. ) ;
#13285=DIRECTION ( 'NONE',  ( -0.000000000000000000, -0.000000000000000000, -1.000000000000000000 ) ) ;
#13290=EDGE_CURVE ( 'NONE', #41885, #10222, #33563, .T. ) ;
#13312=FACE_OUTER_BOUND ( 'NONE', #18532, .T. ) ;
#13324=FACE_OUTER_BOUND ( 'NONE', #7773, .T. ) ;
#13326=DIRECTION ( 'NONE',  ( -0.000000000000000000, -0.000000000000000000, 1.000000000000000000 ) ) ;
#13329=EDGE_CURVE ( 'NONE', #19934, #42661, #25605, .T. ) ;
#13344=ADVANCED_FACE ( 'NONE', ( #29963 ), #28946, .F. ) ;
#13351=DIRECTION ( 'NONE',  ( -1.000000000000000000, 0.000000000000000000, -0.000000000000000000 ) ) ;
#13353=EDGE_LOOP ( 'NONE', ( #14141, #47914, #1966, #11450 ) ) ;
#13354=DIRECTION ( 'NONE',  ( -0.000000000000000000, -1.000000000000000000, -0.000000000000000000 ) ) ;
#13364=( LENGTH_UNIT ( ) NAMED_UNIT ( * ) SI_UNIT ( .MILLI., .METRE. ) );
#13367=ADVANCED_FACE ( 'NONE', ( #17885 ), #4024, .F. ) ;
#13374=DIRECTION ( 'NONE',  ( -0.000000000000000000, -1.000000000000000000, -0.000000000000000000 ) ) ;
#13376=CARTESIAN_POINT ( 'NONE',  ( 135.0000000000003411, 17.00000000000000000, -60.00000000000000000 ) ) ;
#13398=DIRECTION ( 'NONE',  ( 0.000000000000000000, 0.000000000000000000, 1.000000000000000000 ) ) ;
#13409=ORIENTED_EDGE ( 'NONE', *, *, #38710, .F. ) ;
#13417=AXIS2_PLACEMENT_3D ( 'NONE', #48764, #37298, #22806 ) ;
#13432=LINE ( 'NONE', #1895, #26241 ) ;
#13438=AXIS2_PLACEMENT_3D ( 'NONE', #48643, #40501, #25602 ) ;
#13444=AXIS2_PLACEMENT_3D ( 'NONE', #17661, #40518, #41019 ) ;
#13452=ORIENTED_EDGE ( 'NONE', *, *, #9244, .F. ) ;
#13453=ORIENTED_EDGE ( 'NONE', *, *, #47690, .T. ) ;
#13456=LINE ( 'NONE', #45483, #48590 ) ;
#13459=ORIENTED_EDGE ( 'NONE', *, *, #39613, .F. ) ;
#13468=CARTESIAN_POINT ( 'NONE',  ( -19.99999999999908695, 17.00000000000000000, -24.99999999999999289 ) ) ;
#13469=CARTESIAN_POINT ( 'NONE',  ( 34.99999999999997868, 16.00000000000000000, -90.00000000000000000 ) ) ;
#13484=LINE ( 'NONE', #17088, #18099 ) ;
#13488=CARTESIAN_POINT ( 'NONE',  ( -114.9999999999978542, 16.00000000000000000, 95.00000000000000000 ) ) ;
#13492=PLANE ( 'NONE',  #2015 ) ;
#13497=DIRECTION ( 'NONE',  ( -1.000000000000000000, -0.000000000000000000, -0.000000000000000000 ) ) ;
#13501=CARTESIAN_POINT ( 'NONE',  ( 164.9999999999999716, 16.00000000000000000, 115.0000000000000142 ) ) ;
#13509=EDGE_LOOP ( 'NONE', ( #40529, #36898, #39777, #14009 ) ) ;
#13517=CARTESIAN_POINT ( 'NONE',  ( -120.0000000000000426, 16.00000000000000000, -114.9999999999999858 ) ) ;
#13540=AXIS2_PLACEMENT_3D ( 'NONE', #40495, #24588, #25341 ) ;
#13545=VERTEX_POINT ( 'NONE', #680 ) ;
#13549=DIRECTION ( 'NONE',  ( -0.000000000000000000, -1.000000000000000000, -0.000000000000000000 ) ) ;
#13552=ORIENTED_EDGE ( 'NONE', *, *, #12792, .T. ) ;
#13554=LINE ( 'NONE', #32126, #40190 ) ;
#13557=CARTESIAN_POINT ( 'NONE',  ( 135.0000000000015632, 17.00000000000000000, 60.00000000000000000 ) ) ;
#13572=VECTOR ( 'NONE', #2531, 1000.000000000000000 ) ;
#13589=DIRECTION ( 'NONE',  ( 0.000000000000000000, 0.000000000000000000, 1.000000000000000000 ) ) ;
#13594=LINE ( 'NONE', #2547, #4019 ) ;
#13598=VERTEX_POINT ( 'NONE', #48083 ) ;
#13601=VECTOR ( 'NONE', #21330, 1000.000000000000000 ) ;
#13602=DIRECTION ( 'NONE',  ( -1.000000000000000000, -0.000000000000000000, -0.000000000000000000 ) ) ;
#13621=PLANE ( 'NONE',  #37174 ) ;
#13622=VERTEX_POINT ( 'NONE', #17589 ) ;
#13635=VECTOR ( 'NONE', #25190, 1000.000000000000000 ) ;
#13646=CARTESIAN_POINT ( 'NONE',  ( 80.00000000000216005, 17.00000000000000000, 95.00000000000000000 ) ) ;
#13654=VERTEX_POINT ( 'NONE', #29642 ) ;
#13657=DIRECTION ( 'NONE',  ( 0.000000000000000000, 0.000000000000000000, 1.000000000000000000 ) ) ;
#13667=LINE ( 'NONE', #48775, #26692 ) ;
#13676=ORIENTED_EDGE ( 'NONE', *, *, #12070, .F. ) ;
#13678=CARTESIAN_POINT ( 'NONE',  ( 35.00000000000152767, 17.00000000000000000, 35.00000000000000000 ) ) ;
#13681=CARTESIAN_POINT ( 'NONE',  ( -114.9999999999987779, 16.00000000000000000, 30.00000000000000000 ) ) ;
#13684=CARTESIAN_POINT ( 'NONE',  ( -69.99999999999909051, 16.00000000000000000, -24.99999999999999289 ) ) ;
#13693=EDGE_LOOP ( 'NONE', ( #25741, #30810, #30183, #11260 ) ) ;
#13695=LINE ( 'NONE', #29358, #8412 ) ;
#13706=AXIS2_PLACEMENT_3D ( 'NONE', #13880, #21090, #6210 ) ;
#13738=VERTEX_POINT ( 'NONE', #19535 ) ;
#13753=ORIENTED_EDGE ( 'NONE', *, *, #35680, .T. ) ;
#13766=DIRECTION ( 'NONE',  ( 1.000000000000000000, 0.000000000000000000, 0.000000000000000000 ) ) ;
#13767=VERTEX_POINT ( 'NONE', #4410 ) ;
#13769=LINE ( 'NONE', #25840, #19028 ) ;
#13772=LINE ( 'NONE', #5575, #48414 ) ;
#13785=CARTESIAN_POINT ( 'NONE',  ( -164.9999999999990905, 16.00000000000000000, 0.000000000000000000 ) ) ;
#13787=FACE_OUTER_BOUND ( 'NONE', #39519, .T. ) ;
#13788=CARTESIAN_POINT ( 'NONE',  ( 30.00000000000187228, 17.00000000000000000, 65.00000000000000000 ) ) ;
#13791=CARTESIAN_POINT ( 'NONE',  ( 30.00000000000217781, 17.00000000000000000, 95.00000000000000000 ) ) ;
#13794=ORIENTED_EDGE ( 'NONE', *, *, #26633, .T. ) ;
#13797=ORIENTED_EDGE ( 'NONE', *, *, #10458, .T. ) ;
#13807=FACE_OUTER_BOUND ( 'NONE', #3867, .T. ) ;
#13811=FACE_OUTER_BOUND ( 'NONE', #10793, .T. ) ;
#13813=CARTESIAN_POINT ( 'NONE',  ( 35.00000000000186162, 17.00000000000000000, 65.00000000000000000 ) ) ;
#13817=ORIENTED_EDGE ( 'NONE', *, *, #14833, .T. ) ;
#13834=VECTOR ( 'NONE', #49968, 1000.000000000000000 ) ;
#13853=DIRECTION ( 'NONE',  ( 1.000000000000000000, 0.000000000000000000, 0.000000000000000000 ) ) ;
#13855=EDGE_LOOP ( 'NONE', ( #4543, #24552, #33388, #40524 ) ) ;
#13858=ORIENTED_EDGE ( 'NONE', *, *, #28790, .T. ) ;
#13874=ORIENTED_EDGE ( 'NONE', *, *, #35351, .F. ) ;
#13879=ORIENTED_EDGE ( 'NONE', *, *, #48708, .T. ) ;
#13880=CARTESIAN_POINT ( 'NONE',  ( 135.0000000000006253, 17.00000000000000000, -54.99999999999999289 ) ) ;
#13881=CARTESIAN_POINT ( 'NONE',  ( -114.9999999999981526, 17.00000000000000000, 90.00000000000000000 ) ) ;
#13883=VECTOR ( 'NONE', #14501, 1000.000000000000000 ) ;
#13885=ORIENTED_EDGE ( 'NONE', *, *, #38710, .T. ) ;
#13887=ORIENTED_EDGE ( 'NONE', *, *, #19976, .T. ) ;
#13890=EDGE_CURVE ( 'NONE', #3258, #49766, #32372, .T. ) ;
#13908=VECTOR ( 'NONE', #30051, 1000.000000000000000 ) ;
#13915=FACE_OUTER_BOUND ( 'NONE', #46248, .T. ) ;
#13917=VECTOR ( 'NONE', #49950, 1000.000000000000000 ) ;
#13924=CARTESIAN_POINT ( 'NONE',  ( 84.99999999999997158, 16.00000000000000000, -114.9999999999999858 ) ) ;
#13927=PLANE ( 'NONE',  #33622 ) ;
#13933=DIRECTION ( 'NONE',  ( -0.000000000000000000, -1.000000000000000000, -0.000000000000000000 ) ) ;
#13935=ORIENTED_EDGE ( 'NONE', *, *, #33053, .F. ) ;
#13936=ORIENTED_EDGE ( 'NONE', *, *, #4728, .T. ) ;
#13938=CARTESIAN_POINT ( 'NONE',  ( -14.99999999999906919, 17.00000000000000000, 0.000000000000000000 ) ) ;
#13945=LINE ( 'NONE', #49314, #48761 ) ;
#13946=VECTOR ( 'NONE', #36881, 1000.000000000000000 ) ;
#13947=DIRECTION ( 'NONE',  ( -0.000000000000000000, -0.000000000000000000, -1.000000000000000000 ) ) ;
#13970=VERTEX_POINT ( 'NONE', #10771 ) ;
#13976=LINE ( 'NONE', #33005, #23191 ) ;
#13981=CARTESIAN_POINT ( 'NONE',  ( 30.00000000000187228, 16.00000000000000000, 65.00000000000000000 ) ) ;
#13993=ORIENTED_EDGE ( 'NONE', *, *, #38119, .F. ) ;
#13994=VECTOR ( 'NONE', #16333, 1000.000000000000000 ) ;
#13995=ORIENTED_EDGE ( 'NONE', *, *, #35555, .F. ) ;
#14009=ORIENTED_EDGE ( 'NONE', *, *, #38401, .T. ) ;
#14011=EDGE_CURVE ( 'NONE', #45021, #36600, #41324, .T. ) ;
#14012=CARTESIAN_POINT ( 'NONE',  ( -120.0000000000000426, 17.00000000000000000, -114.9999999999999858 ) ) ;
#14014=ORIENTED_EDGE ( 'NONE', *, *, #36688, .T. ) ;
#14033=DIRECTION ( 'NONE',  ( 1.000000000000000000, 0.000000000000000000, 0.000000000000000000 ) ) ;
#14036=CARTESIAN_POINT ( 'NONE',  ( 80.00000000000186162, 17.00000000000000000, 65.00000000000000000 ) ) ;
#14042=EDGE_CURVE ( 'NONE', #46181, #23633, #50221, .T. ) ;
#14054=VERTEX_POINT ( 'NONE', #15395 ) ;
#14055=ORIENTED_EDGE ( 'NONE', *, *, #8275, .T. ) ;
#14071=DIRECTION ( 'NONE',  ( -0.000000000000000000, -1.000000000000000000, -0.000000000000000000 ) ) ;
#14073=LINE ( 'NONE', #49931, #32459 ) ;
#14076=CARTESIAN_POINT ( 'NONE',  ( 85.00000000000029843, 17.00000000000000000, -60.00000000000000000 ) ) ;
#14085=FACE_BOUND ( 'NONE', #37139, .T. ) ;
#14088=FACE_OUTER_BOUND ( 'NONE', #28870, .T. ) ;
#14092=VECTOR ( 'NONE', #38564, 1000.000000000000000 ) ;
#14099=LINE ( 'NONE', #36993, #24049 ) ;
#14105=CARTESIAN_POINT ( 'NONE',  ( -165.0000000000000284, 16.00000000000000000, 65.00000000000000000 ) ) ;
#14110=EDGE_LOOP ( 'NONE', ( #30884, #47950, #2278, #26267 ) ) ;
#14113=AXIS2_PLACEMENT_3D ( 'NONE', #28098, #39916, #650 ) ;
#14118=LINE ( 'NONE', #22083, #13908 ) ;
#14120=VECTOR ( 'NONE', #29192, 1000.000000000000000 ) ;
#14126=VERTEX_POINT ( 'NONE', #27699 ) ;
#14127=ORIENTED_EDGE ( 'NONE', *, *, #46529, .T. ) ;
#14131=CARTESIAN_POINT ( 'NONE',  ( 80.00000000000217426, 17.00000000000000000, 115.0000000000000142 ) ) ;
#14141=ORIENTED_EDGE ( 'NONE', *, *, #38548, .T. ) ;
#14143=DIRECTION ( 'NONE',  ( -1.000000000000000000, -0.000000000000000000, -0.000000000000000000 ) ) ;
#14161=CARTESIAN_POINT ( 'NONE',  ( -164.9999999999997442, 17.00000000000000000, -84.99999999999998579 ) ) ;
#14173=ORIENTED_EDGE ( 'NONE', *, *, #24434, .F. ) ;
#14175=VERTEX_POINT ( 'NONE', #46132 ) ;
#14181=EDGE_LOOP ( 'NONE', ( #33244, #5405, #47307, #512, #34428, #45728, #10469, #38789, #3474, #35448, #26654, #41206, #47094, #26944, #40847, #2976, #32472, #4493, #1038, #17660, #1776, #38624, #42273, #2390, #37908, #21573, #22614, #46661 ) ) ;
#14184=CARTESIAN_POINT ( 'NONE',  ( 85.00000000000029843, 16.00000000000000000, -60.00000000000000000 ) ) ;
#14188=LINE ( 'NONE', #22657, #38065 ) ;
#14192=ORIENTED_EDGE ( 'NONE', *, *, #10378, .F. ) ;
#14197=ADVANCED_FACE ( 'NONE', ( #44082 ), #36690, .F. ) ;
#14205=LINE ( 'NONE', #29873, #30606 ) ;
#14218=DIRECTION ( 'NONE',  ( 0.000000000000000000, 0.000000000000000000, 1.000000000000000000 ) ) ;
#14221=DIRECTION ( 'NONE',  ( 1.000000000000000000, 0.000000000000000000, -4.625929269271542120E-16 ) ) ;
#14222=ORIENTED_EDGE ( 'NONE', *, *, #6089, .F. ) ;
#14233=FACE_OUTER_BOUND ( 'NONE', #43673, .T. ) ;
#14261=CARTESIAN_POINT ( 'NONE',  ( 164.9999999999999716, 17.00000000000000000, 90.00000000000000000 ) ) ;
#14270=EDGE_CURVE ( 'NONE', #34291, #38172, #12802, .T. ) ;
#14271=ORIENTED_EDGE ( 'NONE', *, *, #17043, .T. ) ;
#14275=VECTOR ( 'NONE', #42303, 1000.000000000000000 ) ;
#14279=LINE ( 'NONE', #25590, #25995 ) ;
#14280=LINE ( 'NONE', #38416, #36003 ) ;
#14285=LINE ( 'NONE', #29951, #49575 ) ;
#14286=EDGE_CURVE ( 'NONE', #2288, #3452, #33827, .T. ) ;
#14292=CARTESIAN_POINT ( 'NONE',  ( 135.0000000000003411, 17.00000000000000000, -84.99999999999998579 ) ) ;
#14295=DIRECTION ( 'NONE',  ( -0.000000000000000000, -0.000000000000000000, -1.000000000000000000 ) ) ;
#14298=ORIENTED_EDGE ( 'NONE', *, *, #92, .T. ) ;
#14302=VECTOR ( 'NONE', #18923, 1000.000000000000000 ) ;
#14304=CARTESIAN_POINT ( 'NONE',  ( 164.9999999999999716, 16.00000000000000000, 115.0000000000000142 ) ) ;
#14305=DIRECTION ( 'NONE',  ( 0.000000000000000000, 0.000000000000000000, -1.000000000000000000 ) ) ;
#14309=CARTESIAN_POINT ( 'NONE',  ( 30.00000000000123279, 17.00000000000000000, 30.00000000000000000 ) ) ;
#14311=EDGE_LOOP ( 'NONE', ( #31858, #32717, #39437, #37216 ) ) ;
#14316=VERTEX_POINT ( 'NONE', #49416 ) ;
#14324=ORIENTED_EDGE ( 'NONE', *, *, #34401, .T. ) ;
#14327=FACE_OUTER_BOUND ( 'NONE', #36724, .T. ) ;
#14328=VECTOR ( 'NONE', #46526, 1000.000000000000000 ) ;
#14332=ORIENTED_EDGE ( 'NONE', *, *, #46919, .T. ) ;
#14334=VERTEX_POINT ( 'NONE', #18148 ) ;
#14337=CARTESIAN_POINT ( 'NONE',  ( -164.9999999999994031, 16.00000000000000000, -30.00000000000000000 ) ) ;
#14341=PLANE ( 'NONE',  #31336 ) ;
#14342=VECTOR ( 'NONE', #43951, 1000.000000000000000 ) ;
#14347=VECTOR ( 'NONE', #45786, 1000.000000000000000 ) ;
#14357=EDGE_CURVE ( 'NONE', #40535, #33858, #21758, .T. ) ;
#14361=CARTESIAN_POINT ( 'NONE',  ( -119.9999999999994174, 17.00000000000000000, -30.00000000000000000 ) ) ;
#14365=ADVANCED_FACE ( 'NONE', ( #37937 ), #29213, .F. ) ;
#14366=PLANE ( 'NONE',  #22014 ) ;
#14368=DIRECTION ( 'NONE',  ( -1.000000000000000000, 0.000000000000000000, 0.000000000000000000 ) ) ;
#14390=CARTESIAN_POINT ( 'NONE',  ( 35.00000000000152767, 16.00000000000000000, 60.00000000000000000 ) ) ;
#14392=ORIENTED_EDGE ( 'NONE', *, *, #9586, .T. ) ;
#14393=EDGE_LOOP ( 'NONE', ( #19448, #20148, #32225, #20808 ) ) ;
#14395=AXIS2_PLACEMENT_3D ( 'NONE', #28384, #10130, #22435 ) ;
#14402=DIRECTION ( 'NONE',  ( -0.000000000000000000, -0.000000000000000000, -1.000000000000000000 ) ) ;
#14403=ORIENTED_EDGE ( 'NONE', *, *, #2483, .F. ) ;
#14407=VECTOR ( 'NONE', #45406, 1000.000000000000000 ) ;
#14409=ORIENTED_EDGE ( 'NONE', *, *, #29114, .F. ) ;
#14421=VECTOR ( 'NONE', #20972, 1000.000000000000000 ) ;
#14425=FACE_OUTER_BOUND ( 'NONE', #49796, .T. ) ;
#14432=CARTESIAN_POINT ( 'NONE',  ( 85.00000000000056843, 17.00000000000000000, -30.00000000000000000 ) ) ;
#14435=LINE ( 'NONE', #36801, #36254 ) ;
#14437=DIRECTION ( 'NONE',  ( -1.000000000000000000, -0.000000000000000000, -0.000000000000000000 ) ) ;
#14438=ORIENTED_EDGE ( 'NONE', *, *, #3049, .T. ) ;
#14441=CARTESIAN_POINT ( 'NONE',  ( -114.9999999999991047, 16.00000000000000000, -24.99999999999999289 ) ) ;
#14450=CARTESIAN_POINT ( 'NONE',  ( -14.99999999999845812, 17.00000000000000000, 60.00000000000000000 ) ) ;
#14463=LINE ( 'NONE', #37836, #43185 ) ;
#14466=DIRECTION ( 'NONE',  ( 1.000000000000000000, 0.000000000000000000, 0.000000000000000000 ) ) ;
#14467=CARTESIAN_POINT ( 'NONE',  ( -165.0000000000000284, 16.00000000000000000, 0.000000000000000000 ) ) ;
#14475=VERTEX_POINT ( 'NONE', #30466 ) ;
#14478=VERTEX_POINT ( 'NONE', #11989 ) ;
#14481=DIRECTION ( 'NONE',  ( 0.000000000000000000, 0.000000000000000000, 1.000000000000000000 ) ) ;
#14499=CARTESIAN_POINT ( 'NONE',  ( 135.0000000000000000, 17.00000000000000000, -90.00000000000000000 ) ) ;
#14501=DIRECTION ( 'NONE',  ( 0.000000000000000000, 0.000000000000000000, 1.000000000000000000 ) ) ;
#14507=LINE ( 'NONE', #18344, #27523 ) ;
#14508=CARTESIAN_POINT ( 'NONE',  ( 164.9999999999999716, 16.00000000000000000, 90.00000000000000000 ) ) ;
#14509=ADVANCED_FACE ( 'NONE', ( #23540 ), #47085, .F. ) ;
#14521=ORIENTED_EDGE ( 'NONE', *, *, #36048, .F. ) ;
#14526=DIRECTION ( 'NONE',  ( 0.000000000000000000, -0.000000000000000000, -1.000000000000000000 ) ) ;
#14534=FACE_OUTER_BOUND ( 'NONE', #12686, .T. ) ;
#14555=VERTEX_POINT ( 'NONE', #19679 ) ;
#14556=CARTESIAN_POINT ( 'NONE',  ( -114.9999999999981526, 16.00000000000000000, 90.00000000000000000 ) ) ;
#14560=VECTOR ( 'NONE', #22188, 1000.000000000000000 ) ;
#14575=LINE ( 'NONE', #12936, #15769 ) ;
#14581=DIRECTION ( 'NONE',  ( 1.000000000000000000, 0.000000000000000000, -0.000000000000000000 ) ) ;
#14592=ADVANCED_FACE ( 'NONE', ( #13233 ), #31755, .F. ) ;
#14593=CARTESIAN_POINT ( 'NONE',  ( -165.0000000000000284, 16.00000000000000000, 115.0000000000000142 ) ) ;
#14594=FACE_OUTER_BOUND ( 'NONE', #44467, .T. ) ;
#14595=FACE_BOUND ( 'NONE', #47294, .T. ) ;
#14606=LINE ( 'NONE', #41807, #48765 ) ;
#14614=CARTESIAN_POINT ( 'NONE',  ( 0.000000000000000000, 17.00000000000000000, 0.000000000000000000 ) ) ;
#14632=EDGE_CURVE ( 'NONE', #33538, #156, #47596, .T. ) ;
#14635=EDGE_LOOP ( 'NONE', ( #44522, #30050, #23714, #3927 ) ) ;
#14646=EDGE_CURVE ( 'NONE', #27796, #7505, #5541, .T. ) ;
#14657=DIRECTION ( 'NONE',  ( 0.000000000000000000, 0.000000000000000000, -1.000000000000000000 ) ) ;
#14659=VECTOR ( 'NONE', #1003, 1000.000000000000000 ) ;
#14664=DIRECTION ( 'NONE',  ( -0.000000000000000000, -1.000000000000000000, -0.000000000000000000 ) ) ;
#14665=LINE ( 'NONE', #30324, #5121 ) ;
#14672=CARTESIAN_POINT ( 'NONE',  ( 85.00000000000029843, 17.00000000000000000, -84.99999999999998579 ) ) ;
#14674=CARTESIAN_POINT ( 'NONE',  ( -19.99999999999908695, 17.00000000000000000, -24.99999999999999289 ) ) ;
#14680=EDGE_CURVE ( 'NONE', #42413, #2747, #2450, .T. ) ;
#14686=CARTESIAN_POINT ( 'NONE',  ( 34.99999999999997868, 16.00000000000000000, -114.9999999999999858 ) ) ;
#14687=CARTESIAN_POINT ( 'NONE',  ( 164.9999999999999716, 17.00000000000000000, -30.00000000000001421 ) ) ;
#14688=ORIENTED_EDGE ( 'NONE', *, *, #14954, .F. ) ;
#14692=EDGE_CURVE ( 'NONE', #24182, #865, #49355, .T. ) ;
#14694=ORIENTED_EDGE ( 'NONE', *, *, #19266, .F. ) ;
#14703=LINE ( 'NONE', #6262, #7932 ) ;
#14704=CARTESIAN_POINT ( 'NONE',  ( -14.99999999999937472, 17.00000000000000000, -30.00000000000000000 ) ) ;
#14716=ORIENTED_EDGE ( 'NONE', *, *, #33766, .F. ) ;
#14732=ORIENTED_EDGE ( 'NONE', *, *, #11449, .T. ) ;
#14741=VECTOR ( 'NONE', #287, 1000.000000000000000 ) ;
#14744=DIRECTION ( 'NONE',  ( 0.000000000000000000, -1.000000000000000000, 0.000000000000000000 ) ) ;
#14758=ORIENTED_EDGE ( 'NONE', *, *, #8771, .F. ) ;
#14759=EDGE_LOOP ( 'NONE', ( #21385, #43174, #15137, #12477 ) ) ;
#14769=DIRECTION ( 'NONE',  ( 0.000000000000000000, 0.000000000000000000, 1.000000000000000000 ) ) ;
#14797=DIRECTION ( 'NONE',  ( -0.000000000000000000, -1.000000000000000000, -0.000000000000000000 ) ) ;
#14801=AXIS2_PLACEMENT_3D ( 'NONE', #37391, #18345, #45777 ) ;
#14826=FACE_OUTER_BOUND ( 'NONE', #10592, .T. ) ;
#14833=EDGE_CURVE ( 'NONE', #22540, #27098, #19098, .T. ) ;
#14851=VERTEX_POINT ( 'NONE', #46524 ) ;
#14855=FACE_BOUND ( 'NONE', #73, .T. ) ;
#14862=EDGE_CURVE ( 'NONE', #5959, #46304, #3965, .T. ) ;
#14884=ORIENTED_EDGE ( 'NONE', *, *, #33974, .T. ) ;
#14894=DIRECTION ( 'NONE',  ( -1.000000000000000000, 0.000000000000000000, 0.000000000000000000 ) ) ;
#14897=LINE ( 'NONE', #41589, #14407 ) ;
#14909=VECTOR ( 'NONE', #39738, 1000.000000000000000 ) ;
#14918=ORIENTED_EDGE ( 'NONE', *, *, #34426, .F. ) ;
#14942=LINE ( 'NONE', #41884, #14092 ) ;
#14954=EDGE_CURVE ( 'NONE', #31678, #22771, #33707, .T. ) ;
#14961=ORIENTED_EDGE ( 'NONE', *, *, #6719, .F. ) ;
#14979=VERTEX_POINT ( 'NONE', #37068 ) ;
#14984=LINE ( 'NONE', #50592, #44445 ) ;
#14989=PLANE ( 'NONE',  #22549 ) ;
#14990=LINE ( 'NONE', #37363, #38259 ) ;
#14991=CARTESIAN_POINT ( 'NONE',  ( -114.9999999999987779, 17.00000000000000000, 30.00000000000000000 ) ) ;
#14995=VECTOR ( 'NONE', #28062, 1000.000000000000000 ) ;
#15000=EDGE_CURVE ( 'NONE', #24319, #9357, #13432, .T. ) ;
#15004=EDGE_CURVE ( 'NONE', #45968, #43076, #33456, .T. ) ;
#15005=EDGE_CURVE ( 'NONE', #9471, #17930, #5985, .T. ) ;
#15009=EDGE_CURVE ( 'NONE', #39423, #45968, #33951, .T. ) ;
#15013=AXIS2_PLACEMENT_3D ( 'NONE', #37682, #26372, #49420 ) ;
#15020=VECTOR ( 'NONE', #47473, 1000.000000000000000 ) ;
#15029=EDGE_LOOP ( 'NONE', ( #28045, #20855, #37158, #29392 ) ) ;
#15035=AXIS2_PLACEMENT_3D ( 'NONE', #1617, #36276, #13398 ) ;
#15039=ORIENTED_EDGE ( 'NONE', *, *, #37546, .F. ) ;
#15041=CARTESIAN_POINT ( 'NONE',  ( 30.00000000000217781, 17.00000000000000000, 95.00000000000000000 ) ) ;
#15045=VERTEX_POINT ( 'NONE', #22391 ) ;
#15059=EDGE_CURVE ( 'NONE', #43076, #22294, #50558, .T. ) ;
#15078=VERTEX_POINT ( 'NONE', #26258 ) ;
#15081=ORIENTED_EDGE ( 'NONE', *, *, #31353, .T. ) ;
#15088=VECTOR ( 'NONE', #42330, 1000.000000000000000 ) ;
#15094=CARTESIAN_POINT ( 'NONE',  ( -69.99999999999783995, 17.00000000000000000, 115.0000000000000142 ) ) ;
#15096=VERTEX_POINT ( 'NONE', #27003 ) ;
#15105=ORIENTED_EDGE ( 'NONE', *, *, #49889, .F. ) ;
#15108=FACE_BOUND ( 'NONE', #4684, .T. ) ;
#15109=AXIS2_PLACEMENT_3D ( 'NONE', #18010, #37307, #17775 ) ;
#15112=DIRECTION ( 'NONE',  ( -0.000000000000000000, -1.000000000000000000, -0.000000000000000000 ) ) ;
#15118=PLANE ( 'NONE',  #12597 ) ;
#15126=LINE ( 'NONE', #4092, #48720 ) ;
#15127=CARTESIAN_POINT ( 'NONE',  ( -19.99999999999784706, 17.00000000000000000, 115.0000000000000142 ) ) ;
#15130=ORIENTED_EDGE ( 'NONE', *, *, #11507, .T. ) ;
#15136=ADVANCED_FACE ( 'NONE', ( #10843 ), #22644, .F. ) ;
#15137=ORIENTED_EDGE ( 'NONE', *, *, #26583, .F. ) ;
#15145=FACE_OUTER_BOUND ( 'NONE', #18684, .T. ) ;
#15150=CARTESIAN_POINT ( 'NONE',  ( -14.99999999999845812, 16.00000000000000000, 35.00000000000000000 ) ) ;
#15163=ORIENTED_EDGE ( 'NONE', *, *, #46826, .T. ) ;
#15172=ORIENTED_EDGE ( 'NONE', *, *, #43493, .F. ) ;
#15183=VECTOR ( 'NONE', #24054, 1000.000000000000000 ) ;
#15184=EDGE_CURVE ( 'NONE', #45555, #3395, #13554, .T. ) ;
#15188=VECTOR ( 'NONE', #20421, 1000.000000000000000 ) ;
#15193=AXIS2_PLACEMENT_3D ( 'NONE', #46442, #12334, #34962 ) ;
#15194=LINE ( 'NONE', #50027, #21212 ) ;
#15205=CARTESIAN_POINT ( 'NONE',  ( -119.9999999999981668, 16.00000000000000000, 65.00000000000000000 ) ) ;
#15206=PLANE ( 'NONE',  #27400 ) ;
#15214=EDGE_CURVE ( 'NONE', #26234, #325, #44837, .T. ) ;
#15218=EDGE_LOOP ( 'NONE', ( #15081, #25236, #9057, #13053 ) ) ;
#15226=EDGE_LOOP ( 'NONE', ( #47289, #47976, #4923, #24887 ) ) ;
#15228=DIRECTION ( 'NONE',  ( 0.000000000000000000, 0.000000000000000000, -1.000000000000000000 ) ) ;
#15230=ORIENTED_EDGE ( 'NONE', *, *, #14270, .T. ) ;
#15232=LINE ( 'NONE', #38082, #39907 ) ;
#15233=EDGE_CURVE ( 'NONE', #32189, #33102, #47481, .T. ) ;
#15261=EDGE_LOOP ( 'NONE', ( #28116, #7187, #706, #8824 ) ) ;
#15271=ORIENTED_EDGE ( 'NONE', *, *, #4927, .T. ) ;
#15280=LINE ( 'NONE', #11176, #14328 ) ;
#15283=ORIENTED_EDGE ( 'NONE', *, *, #50324, .F. ) ;
#15294=ORIENTED_EDGE ( 'NONE', *, *, #17702, .T. ) ;
#15305=CARTESIAN_POINT ( 'NONE',  ( 0.000000000000000000, 17.00000000000000000, 0.000000000000000000 ) ) ;
#15322=VERTEX_POINT ( 'NONE', #49919 ) ;
#15326=LINE ( 'NONE', #19146, #11334 ) ;
#15327=AXIS2_PLACEMENT_3D ( 'NONE', #22661, #3409, #41914 ) ;
#15334=ORIENTED_EDGE ( 'NONE', *, *, #27169, .T. ) ;
#15338=DIRECTION ( 'NONE',  ( 0.000000000000000000, 0.000000000000000000, 1.000000000000000000 ) ) ;
#15348=EDGE_CURVE ( 'NONE', #34745, #41862, #9710, .T. ) ;
#15349=ORIENTED_EDGE ( 'NONE', *, *, #31088, .T. ) ;
#15351=LINE ( 'NONE', #19174, #36826 ) ;
#15352=CARTESIAN_POINT ( 'NONE',  ( -64.99999999999971578, 17.00000000000000000, -60.00000000000000000 ) ) ;
#15365=DIRECTION ( 'NONE',  ( -0.000000000000000000, -0.000000000000000000, -1.000000000000000000 ) ) ;
#15366=EDGE_CURVE ( 'NONE', #22529, #16567, #3014, .T. ) ;
#15387=CARTESIAN_POINT ( 'NONE',  ( -165.0000000000000284, 16.00000000000000000, 115.0000000000000142 ) ) ;
#15395=CARTESIAN_POINT ( 'NONE',  ( 135.0000000000006253, 16.00000000000000000, -54.99999999999999289 ) ) ;
#15399=VERTEX_POINT ( 'NONE', #25369 ) ;
#15404=LINE ( 'NONE', #35931, #6519 ) ;
#15415=LINE ( 'NONE', #42595, #23985 ) ;
#15421=ORIENTED_EDGE ( 'NONE', *, *, #35913, .T. ) ;
#15423=CARTESIAN_POINT ( 'NONE',  ( 130.0000000000021032, 16.00000000000000000, 95.00000000000000000 ) ) ;
#15437=LINE ( 'NONE', #38556, #15996 ) ;
#15438=LINE ( 'NONE', #22370, #5132 ) ;
#15449=CARTESIAN_POINT ( 'NONE',  ( 80.00000000000122213, 17.00000000000000000, 5.000000000000004441 ) ) ;
#15450=DIRECTION ( 'NONE',  ( -1.000000000000000000, -0.000000000000000000, 4.625929269271687073E-16 ) ) ;
#15451=VERTEX_POINT ( 'NONE', #10473 ) ;
#15452=FACE_OUTER_BOUND ( 'NONE', #31590, .T. ) ;
#15453=DIRECTION ( 'NONE',  ( 1.000000000000000000, 0.000000000000000000, 0.000000000000000000 ) ) ;
#15456=DIRECTION ( 'NONE',  ( -1.000000000000000000, 0.000000000000000000, -0.000000000000000000 ) ) ;
#15459=ORIENTED_EDGE ( 'NONE', *, *, #46335, .T. ) ;
#15461=FACE_OUTER_BOUND ( 'NONE', #14311, .T. ) ;
#15463=VECTOR ( 'NONE', #29132, 1000.000000000000000 ) ;
#15465=EDGE_LOOP ( 'NONE', ( #43240, #45285, #30741, #20708 ) ) ;
#15472=CARTESIAN_POINT ( 'NONE',  ( 135.0000000000012790, 17.00000000000000000, 5.000000000000004441 ) ) ;
#15487=CARTESIAN_POINT ( 'NONE',  ( 30.00000000000029132, 16.00000000000000000, -84.99999999999998579 ) ) ;
#15517=VECTOR ( 'NONE', #6554, 1000.000000000000000 ) ;
#15548=CARTESIAN_POINT ( 'NONE',  ( -64.99999999999846523, 17.00000000000000000, 60.00000000000000000 ) ) ;
#15553=CARTESIAN_POINT ( 'NONE',  ( -114.9999999999987779, 16.00000000000000000, 5.000000000000004441 ) ) ;
#15559=VECTOR ( 'NONE', #44515, 1000.000000000000000 ) ;
#15564=CARTESIAN_POINT ( 'NONE',  ( 35.00000000000152767, 17.00000000000000000, 35.00000000000000000 ) ) ;
#15582=ORIENTED_EDGE ( 'NONE', *, *, #19728, .T. ) ;
#15589=EDGE_LOOP ( 'NONE', ( #29356, #36432, #18559, #13887 ) ) ;
#15596=ADVANCED_FACE ( 'NONE', ( #12749 ), #44524, .F. ) ;
#15604=VERTEX_POINT ( 'NONE', #28157 ) ;
#15617=LINE ( 'NONE', #43058, #34034 ) ;
#15625=CARTESIAN_POINT ( 'NONE',  ( 35.00000000000028422, 17.00000000000000000, -84.99999999999998579 ) ) ;
#15628=CARTESIAN_POINT ( 'NONE',  ( -64.99999999999846523, 17.00000000000000000, 35.00000000000000000 ) ) ;
#15634=CARTESIAN_POINT ( 'NONE',  ( 85.00000000000029843, 17.00000000000000000, -84.99999999999998579 ) ) ;
#15635=DIRECTION ( 'NONE',  ( 1.000000000000000000, 0.000000000000000000, 0.000000000000000000 ) ) ;
#15640=ORIENTED_EDGE ( 'NONE', *, *, #22992, .T. ) ;
#15653=CARTESIAN_POINT ( 'NONE',  ( 30.00000000000218492, 17.00000000000000000, 115.0000000000000142 ) ) ;
#15657=EDGE_LOOP ( 'NONE', ( #20614, #4539, #26329, #40733 ) ) ;
#15660=PLANE ( 'NONE',  #46849 ) ;
#15668=ADVANCED_FACE ( 'NONE', ( #37634 ), #40961, .F. ) ;
#15685=PLANE ( 'NONE',  #28311 ) ;
#15687=DIRECTION ( 'NONE',  ( 0.000000000000000000, -1.000000000000000000, 0.000000000000000000 ) ) ;
#15692=VECTOR ( 'NONE', #40079, 1000.000000000000000 ) ;
#15708=LINE ( 'NONE', #42642, #10564 ) ;
#15714=CARTESIAN_POINT ( 'NONE',  ( 85.00000000000152056, 17.00000000000000000, 35.00000000000000000 ) ) ;
#15720=VERTEX_POINT ( 'NONE', #14508 ) ;
#15724=DIRECTION ( 'NONE',  ( -0.000000000000000000, -1.000000000000000000, -0.000000000000000000 ) ) ;
#15728=DIRECTION ( 'NONE',  ( -1.000000000000000000, -0.000000000000000000, -0.000000000000000000 ) ) ;
#15739=ORIENTED_EDGE ( 'NONE', *, *, #36078, .F. ) ;
#15741=VERTEX_POINT ( 'NONE', #48608 ) ;
#15750=ORIENTED_EDGE ( 'NONE', *, *, #46471, .F. ) ;
#15760=ORIENTED_EDGE ( 'NONE', *, *, #46234, .F. ) ;
#15769=VECTOR ( 'NONE', #36065, 1000.000000000000000 ) ;
#15776=ORIENTED_EDGE ( 'NONE', *, *, #27154, .T. ) ;
#15777=VERTEX_POINT ( 'NONE', #29404 ) ;
#15780=FACE_OUTER_BOUND ( 'NONE', #42463, .T. ) ;
#15781=DIRECTION ( 'NONE',  ( 1.000000000000000000, 0.000000000000000000, 0.000000000000000000 ) ) ;
#15801=CARTESIAN_POINT ( 'NONE',  ( 35.00000000000216716, 17.00000000000000000, 95.00000000000000000 ) ) ;
#15808=DIRECTION ( 'NONE',  ( 0.000000000000000000, 0.000000000000000000, 1.000000000000000000 ) ) ;
#15811=FACE_OUTER_BOUND ( 'NONE', #30201, .T. ) ;
#15817=LINE ( 'NONE', #23527, #26893 ) ;
#15819=CARTESIAN_POINT ( 'NONE',  ( 130.0000000000008811, 16.00000000000000000, -24.99999999999999289 ) ) ;
#15834=ORIENTED_EDGE ( 'NONE', *, *, #9244, .T. ) ;
#15835=DIRECTION ( 'NONE',  ( -1.000000000000000000, 0.000000000000000000, -0.000000000000000000 ) ) ;
#15844=DIRECTION ( 'NONE',  ( 3.469446951953611231E-16, -0.000000000000000000, -1.000000000000000000 ) ) ;
#15849=EDGE_CURVE ( 'NONE', #22918, #3086, #23491, .T. ) ;
#15869=VECTOR ( 'NONE', #10526, 1000.000000000000000 ) ;
#15886=PLANE ( 'NONE',  #12591 ) ;
#15889=DIRECTION ( 'NONE',  ( 1.000000000000000000, 0.000000000000000000, 0.000000000000000000 ) ) ;
#15890=CARTESIAN_POINT ( 'NONE',  ( 85.00000000000029843, 17.00000000000000000, -60.00000000000000000 ) ) ;
#15893=PLANE ( 'NONE',  #41844 ) ;
#15898=VECTOR ( 'NONE', #9217, 1000.000000000000000 ) ;
#15911=DIRECTION ( 'NONE',  ( -0.000000000000000000, -1.000000000000000000, -0.000000000000000000 ) ) ;
#15916=CARTESIAN_POINT ( 'NONE',  ( 164.9999999999999716, 16.00000000000000000, -54.99999999999999289 ) ) ;
#15919=CARTESIAN_POINT ( 'NONE',  ( 85.00000000000029843, 16.00000000000000000, -60.00000000000000000 ) ) ;
#15923=ADVANCED_FACE ( 'NONE', ( #44470 ), #12929, .F. ) ;
#15924=DIRECTION ( 'NONE',  ( 0.000000000000000000, 0.000000000000000000, -1.000000000000000000 ) ) ;
#15938=ORIENTED_EDGE ( 'NONE', *, *, #32856, .F. ) ;
#15939=VECTOR ( 'NONE', #42151, 1000.000000000000000 ) ;
#15946=VECTOR ( 'NONE', #9054, 1000.000000000000000 ) ;
#15950=CARTESIAN_POINT ( 'NONE',  ( 30.00000000000092726, 17.00000000000000000, -24.99999999999999289 ) ) ;
#15963=EDGE_LOOP ( 'NONE', ( #32903, #50244, #15739, #27600 ) ) ;
#15969=EDGE_CURVE ( 'NONE', #26234, #43085, #2645, .T. ) ;
#15970=PLANE ( 'NONE',  #47412 ) ;
#15972=VERTEX_POINT ( 'NONE', #37075 ) ;
#15979=LINE ( 'NONE', #31650, #18524 ) ;
#15982=ORIENTED_EDGE ( 'NONE', *, *, #31550, .T. ) ;
#15984=DIRECTION ( 'NONE',  ( -0.000000000000000000, -1.000000000000000000, -0.000000000000000000 ) ) ;
#15994=EDGE_CURVE ( 'NONE', #37254, #4263, #41142, .T. ) ;
#15996=VECTOR ( 'NONE', #50278, 1000.000000000000000 ) ;
#16006=VERTEX_POINT ( 'NONE', #29857 ) ;
#16023=FACE_OUTER_BOUND ( 'NONE', #16245, .T. ) ;
#16027=LINE ( 'NONE', #42440, #46630 ) ;
#16028=VERTEX_POINT ( 'NONE', #21911 ) ;
#16051=VERTEX_POINT ( 'NONE', #10363 ) ;
#16052=VERTEX_POINT ( 'NONE', #48549 ) ;
#16058=LINE ( 'NONE', #47054, #6604 ) ;
#16065=VERTEX_POINT ( 'NONE', #14184 ) ;
#16072=LINE ( 'NONE', #15564, #6907 ) ;
#16073=VECTOR ( 'NONE', #14466, 1000.000000000000000 ) ;
#16074=ORIENTED_EDGE ( 'NONE', *, *, #24934, .T. ) ;
#16080=VECTOR ( 'NONE', #20539, 1000.000000000000000 ) ;
#16102=DIRECTION ( 'NONE',  ( -0.000000000000000000, -0.000000000000000000, -1.000000000000000000 ) ) ;
#16103=LINE ( 'NONE', #27912, #8545 ) ;
#16105=ORIENTED_EDGE ( 'NONE', *, *, #24275, .F. ) ;
#16120=FACE_OUTER_BOUND ( 'NONE', #5353, .T. ) ;
#16121=EDGE_CURVE ( 'NONE', #24878, #23700, #30365, .T. ) ;
#16125=AXIS2_PLACEMENT_3D ( 'NONE', #24135, #12309, #39782 ) ;
#16143=DIRECTION ( 'NONE',  ( -0.000000000000000000, -0.000000000000000000, -1.000000000000000000 ) ) ;
#16145=FACE_OUTER_BOUND ( 'NONE', #632, .T. ) ;
#16153=EDGE_CURVE ( 'NONE', #16517, #15399, #10852, .T. ) ;
#16154=ORIENTED_EDGE ( 'NONE', *, *, #30709, .F. ) ;
#16167=LINE ( 'NONE', #43343, #18813 ) ;
#16168=CARTESIAN_POINT ( 'NONE',  ( -64.99999999999971578, 17.00000000000000000, -60.00000000000000000 ) ) ;
#16174=PLANE ( 'NONE',  #16125 ) ;
#16184=DIRECTION ( 'NONE',  ( 0.000000000000000000, 0.000000000000000000, -1.000000000000000000 ) ) ;
#16192=DIRECTION ( 'NONE',  ( 1.000000000000000000, 0.000000000000000000, -0.000000000000000000 ) ) ;
#16206=DIRECTION ( 'NONE',  ( 0.000000000000000000, -1.000000000000000000, 0.000000000000000000 ) ) ;
#16212=VECTOR ( 'NONE', #20857, 1000.000000000000000 ) ;
#16217=LINE ( 'NONE', #8024, #8549 ) ;
#16218=EDGE_CURVE ( 'NONE', #42092, #35238, #4447, .T. ) ;
#16225=ORIENTED_EDGE ( 'NONE', *, *, #15849, .T. ) ;
#16235=DIRECTION ( 'NONE',  ( 0.000000000000000000, 0.000000000000000000, 1.000000000000000000 ) ) ;
#16245=EDGE_LOOP ( 'NONE', ( #35119, #4262, #3166, #34236 ) ) ;
#16250=CARTESIAN_POINT ( 'NONE',  ( 80.00000000000122213, 17.00000000000000000, 5.000000000000004441 ) ) ;
#16251=LINE ( 'NONE', #5203, #331 ) ;
#16253=DIRECTION ( 'NONE',  ( 0.000000000000000000, -1.000000000000000000, 0.000000000000000000 ) ) ;
#16259=DIRECTION ( 'NONE',  ( 0.000000000000000000, 0.000000000000000000, 1.000000000000000000 ) ) ;
#16279=ADVANCED_FACE ( 'NONE', ( #26787 ), #50330, .F. ) ;
#16286=LINE ( 'NONE', #8088, #28296 ) ;
#16288=ORIENTED_EDGE ( 'NONE', *, *, #32398, .F. ) ;
#16290=VERTEX_POINT ( 'NONE', #3936 ) ;
#16319=DIRECTION ( 'NONE',  ( 0.000000000000000000, -0.000000000000000000, 1.000000000000000000 ) ) ;
#16326=DIRECTION ( 'NONE',  ( -1.000000000000000000, 0.000000000000000000, 0.000000000000000000 ) ) ;
#16330=CARTESIAN_POINT ( 'NONE',  ( -69.99999999999816680, 16.00000000000000000, 65.00000000000000000 ) ) ;
#16333=DIRECTION ( 'NONE',  ( -0.000000000000000000, -0.000000000000000000, -1.000000000000000000 ) ) ;
#16351=ORIENTED_EDGE ( 'NONE', *, *, #30737, .F. ) ;
#16365=VERTEX_POINT ( 'NONE', #20596 ) ;
#16367=CARTESIAN_POINT ( 'NONE',  ( -19.99999999999908695, 17.00000000000000000, -24.99999999999999289 ) ) ;
#16372=LINE ( 'NONE', #7671, #14909 ) ;
#16379=PLANE ( 'NONE',  #27297 ) ;
#16381=VECTOR ( 'NONE', #9030, 1000.000000000000000 ) ;
#16383=PLANE ( 'NONE',  #31480 ) ;
#16388=LINE ( 'NONE', #12286, #44954 ) ;
#16389=CARTESIAN_POINT ( 'NONE',  ( 135.0000000000019043, 17.00000000000000000, 65.00000000000000000 ) ) ;
#16400=ORIENTED_EDGE ( 'NONE', *, *, #19527, .T. ) ;
#16403=ORIENTED_EDGE ( 'NONE', *, *, #39122, .T. ) ;
#16406=ORIENTED_EDGE ( 'NONE', *, *, #34690, .F. ) ;
#16410=CARTESIAN_POINT ( 'NONE',  ( 135.0000000000009663, 16.00000000000000000, 0.000000000000000000 ) ) ;
#16416=ORIENTED_EDGE ( 'NONE', *, *, #30737, .T. ) ;
#16423=CARTESIAN_POINT ( 'NONE',  ( -114.9999999999991047, 17.00000000000000000, 0.000000000000000000 ) ) ;
#16424=CARTESIAN_POINT ( 'NONE',  ( -119.9999999999997158, 17.00000000000000000, -84.99999999999998579 ) ) ;
#16427=AXIS2_PLACEMENT_3D ( 'NONE', #24080, #8684, #9169 ) ;
#16430=VECTOR ( 'NONE', #16642, 1000.000000000000000 ) ;
#16432=ORIENTED_EDGE ( 'NONE', *, *, #18044, .T. ) ;
#16437=PLANE ( 'NONE',  #34 ) ;
#16453=FACE_OUTER_BOUND ( 'NONE', #14181, .T. ) ;
#16460=EDGE_CURVE ( 'NONE', #44725, #42432, #26908, .T. ) ;
#16464=AXIS2_PLACEMENT_3D ( 'NONE', #24858, #24614, #27952 ) ;
#16471=CARTESIAN_POINT ( 'NONE',  ( 135.0000000000000000, 16.00000000000000000, -90.00000000000000000 ) ) ;
#16473=DIRECTION ( 'NONE',  ( 0.000000000000000000, 0.000000000000000000, 1.000000000000000000 ) ) ;
#16475=CARTESIAN_POINT ( 'NONE',  ( -115.0000000000000284, 17.00000000000000000, -114.9999999999999858 ) ) ;
#16479=CARTESIAN_POINT ( 'NONE',  ( 85.00000000000056843, 16.00000000000000000, -54.99999999999999289 ) ) ;
#16485=LINE ( 'NONE', #839, #47917 ) ;
#16488=PLANE ( 'NONE',  #39876 ) ;
#16492=LINE ( 'NONE', #12137, #34138 ) ;
#16495=ORIENTED_EDGE ( 'NONE', *, *, #36329, .T. ) ;
#16501=EDGE_CURVE ( 'NONE', #2288, #26701, #19458, .T. ) ;
#16517=VERTEX_POINT ( 'NONE', #3044 ) ;
#16519=CARTESIAN_POINT ( 'NONE',  ( -120.0000000000000426, 17.00000000000000000, -90.00000000000000000 ) ) ;
#16520=DIRECTION ( 'NONE',  ( -1.000000000000000000, 0.000000000000000000, 0.000000000000000000 ) ) ;
#16525=CARTESIAN_POINT ( 'NONE',  ( -64.99999999999971578, 16.00000000000000000, -60.00000000000000000 ) ) ;
#16535=ORIENTED_EDGE ( 'NONE', *, *, #15000, .F. ) ;
#16543=VECTOR ( 'NONE', #38946, 1000.000000000000000 ) ;
#16544=ORIENTED_EDGE ( 'NONE', *, *, #28537, .T. ) ;
#16547=EDGE_LOOP ( 'NONE', ( #50554, #49191, #22850, #9000 ) ) ;
#16567=VERTEX_POINT ( 'NONE', #40236 ) ;
#16605=VECTOR ( 'NONE', #49018, 1000.000000000000000 ) ;
#16608=CARTESIAN_POINT ( 'NONE',  ( -19.99999999999846523, 17.00000000000000000, 35.00000000000000000 ) ) ;
#16617=ORIENTED_EDGE ( 'NONE', *, *, #39122, .F. ) ;
#16621=EDGE_LOOP ( 'NONE', ( #42569, #1900, #20383, #27038 ) ) ;
#16637=DIRECTION ( 'NONE',  ( 0.000000000000000000, 0.000000000000000000, -1.000000000000000000 ) ) ;
#16642=DIRECTION ( 'NONE',  ( 1.000000000000000000, 0.000000000000000000, 0.000000000000000000 ) ) ;
#16653=ORIENTED_EDGE ( 'NONE', *, *, #12283, .F. ) ;
#16658=VECTOR ( 'NONE', #33274, 1000.000000000000000 ) ;
#16660=DIRECTION ( 'NONE',  ( 1.000000000000000000, 0.000000000000000000, 0.000000000000000000 ) ) ;
#16661=LINE ( 'NONE', #20761, #49590 ) ;
#16670=CARTESIAN_POINT ( 'NONE',  ( 35.00000000000186162, 17.00000000000000000, 65.00000000000000000 ) ) ;
#16672=CARTESIAN_POINT ( 'NONE',  ( -119.9999999999990905, 17.00000000000000000, 0.000000000000000000 ) ) ;
#16673=DIRECTION ( 'NONE',  ( -0.000000000000000000, -1.000000000000000000, -0.000000000000000000 ) ) ;
#16688=CARTESIAN_POINT ( 'NONE',  ( 30.00000000000217781, 16.00000000000000000, 95.00000000000000000 ) ) ;
#16695=LINE ( 'NONE', #48212, #7529 ) ;
#16717=EDGE_CURVE ( 'NONE', #35676, #35737, #48131, .T. ) ;
#16720=CARTESIAN_POINT ( 'NONE',  ( 84.99999999999997158, 16.00000000000000000, -114.9999999999999858 ) ) ;
#16732=CARTESIAN_POINT ( 'NONE',  ( -14.99999999999812594, 16.00000000000000000, 65.00000000000000000 ) ) ;
#16736=ORIENTED_EDGE ( 'NONE', *, *, #26240, .F. ) ;
#16744=DIRECTION ( 'NONE',  ( -0.000000000000000000, -1.000000000000000000, -0.000000000000000000 ) ) ;
#16745=CARTESIAN_POINT ( 'NONE',  ( 164.9999999999999716, 17.00000000000000000, -1.387778780781445676E-14 ) ) ;
#16747=EDGE_CURVE ( 'NONE', #46762, #2324, #40988, .T. ) ;
#16753=LINE ( 'NONE', #49261, #18518 ) ;
#16757=EDGE_CURVE ( 'NONE', #25407, #28907, #13772, .T. ) ;
#16762=CARTESIAN_POINT ( 'NONE',  ( -69.99999999999879208, 16.00000000000000000, 5.000000000000004441 ) ) ;
#16771=DIRECTION ( 'NONE',  ( -1.000000000000000000, 0.000000000000000000, 0.000000000000000000 ) ) ;
#16779=LINE ( 'NONE', #24486, #9026 ) ;
#16783=AXIS2_PLACEMENT_3D ( 'NONE', #20919, #31978, #40428 ) ;
#16784=EDGE_LOOP ( 'NONE', ( #10613, #18108, #34214, #21013 ) ) ;
#16788=DIRECTION ( 'NONE',  ( -1.000000000000000000, 0.000000000000000000, -0.000000000000000000 ) ) ;
#16792=EDGE_CURVE ( 'NONE', #32969, #27078, #7104, .T. ) ;
#16797=AXIS2_PLACEMENT_3D ( 'NONE', #2514, #45825, #21502 ) ;
#16799=ORIENTED_EDGE ( 'NONE', *, *, #37565, .F. ) ;
#16820=ORIENTED_EDGE ( 'NONE', *, *, #3004, .T. ) ;
#16826=CARTESIAN_POINT ( 'NONE',  ( 130.0000000000018474, 17.00000000000000000, 65.00000000000000000 ) ) ;
#16834=CARTESIAN_POINT ( 'NONE',  ( 35.00000000000186162, 16.00000000000000000, 65.00000000000000000 ) ) ;
#16835=VECTOR ( 'NONE', #42699, 1000.000000000000000 ) ;
#16837=VECTOR ( 'NONE', #3569, 1000.000000000000000 ) ;
#16843=VERTEX_POINT ( 'NONE', #42486 ) ;
#16848=DIRECTION ( 'NONE',  ( 0.000000000000000000, -1.000000000000000000, 0.000000000000000000 ) ) ;
#16850=VECTOR ( 'NONE', #21981, 1000.000000000000000 ) ;
#16865=PLANE ( 'NONE',  #38562 ) ;
#16866=VERTEX_POINT ( 'NONE', #50408 ) ;
#16868=EDGE_CURVE ( 'NONE', #23377, #43115, #14280, .T. ) ;
#16874=AXIS2_PLACEMENT_3D ( 'NONE', #2956, #49855, #39153 ) ;
#16882=PLANE ( 'NONE',  #16427 ) ;
#16892=AXIS2_PLACEMENT_3D ( 'NONE', #23887, #4389, #47447 ) ;
#16893=CARTESIAN_POINT ( 'NONE',  ( -19.99999999999815969, 17.00000000000000000, 65.00000000000000000 ) ) ;
#16894=CARTESIAN_POINT ( 'NONE',  ( -164.9999999999997442, 16.00000000000000000, -84.99999999999998579 ) ) ;
#16908=LINE ( 'NONE', #13785, #16430 ) ;
#16910=VECTOR ( 'NONE', #49306, 1000.000000000000000 ) ;
#16912=ADVANCED_FACE ( 'NONE', ( #14534 ), #46053, .F. ) ;
#16913=EDGE_CURVE ( 'NONE', #865, #16365, #19660, .T. ) ;
#16917=EDGE_LOOP ( 'NONE', ( #50591, #21579, #50526, #33889 ) ) ;
#16923=ORIENTED_EDGE ( 'NONE', *, *, #49599, .T. ) ;
#16929=CARTESIAN_POINT ( 'NONE',  ( 130.0000000000018474, 16.00000000000000000, 90.00000000000000000 ) ) ;
#16938=VECTOR ( 'NONE', #18489, 1000.000000000000000 ) ;
#16948=DIRECTION ( 'NONE',  ( 0.000000000000000000, -1.000000000000000000, 0.000000000000000000 ) ) ;
#16949=FACE_OUTER_BOUND ( 'NONE', #17375, .T. ) ;
#16963=DIRECTION ( 'NONE',  ( -1.000000000000000000, -0.000000000000000000, -0.000000000000000000 ) ) ;
#16967=AXIS2_PLACEMENT_3D ( 'NONE', #31010, #34595, #19700 ) ;
#16980=PLANE ( 'NONE',  #25393 ) ;
#16987=ORIENTED_EDGE ( 'NONE', *, *, #23993, .F. ) ;
#16988=CARTESIAN_POINT ( 'NONE',  ( -119.9999999999978400, 16.00000000000000000, 95.00000000000000000 ) ) ;
#16990=DIRECTION ( 'NONE',  ( 0.000000000000000000, 0.000000000000000000, -1.000000000000000000 ) ) ;
#17010=( NAMED_UNIT ( * ) SI_UNIT ( $, .STERADIAN. ) SOLID_ANGLE_UNIT ( ) );
#17011=LINE ( 'NONE', #36790, #20411 ) ;
#17014=VECTOR ( 'NONE', #44252, 1000.000000000000000 ) ;
#17026=VERTEX_POINT ( 'NONE', #20407 ) ;
#17031=ORIENTED_EDGE ( 'NONE', *, *, #12381, .T. ) ;
#17038=ADVANCED_FACE ( 'NONE', ( #39435 ), #23772, .F. ) ;
#17043=EDGE_CURVE ( 'NONE', #17726, #43380, #31225, .T. ) ;
#17047=VERTEX_POINT ( 'NONE', #43508 ) ;
#17054=VERTEX_POINT ( 'NONE', #27361 ) ;
#17062=EDGE_LOOP ( 'NONE', ( #9853, #3969, #13213, #28036 ) ) ;
#17066=FACE_OUTER_BOUND ( 'NONE', #17062, .T. ) ;
#17069=EDGE_CURVE ( 'NONE', #21648, #46923, #7877, .T. ) ;
#17080=CARTESIAN_POINT ( 'NONE',  ( -119.9999999999990905, 16.00000000000000000, -24.99999999999999289 ) ) ;
#17082=VECTOR ( 'NONE', #41123, 1000.000000000000000 ) ;
#17088=CARTESIAN_POINT ( 'NONE',  ( 135.0000000000012790, 17.00000000000000000, 5.000000000000004441 ) ) ;
#17091=EDGE_CURVE ( 'NONE', #35246, #7644, #28614, .T. ) ;
#17094=CARTESIAN_POINT ( 'NONE',  ( -164.9999999999987779, 17.00000000000000000, 5.000000000000004441 ) ) ;
#17110=VERTEX_POINT ( 'NONE', #41170 ) ;
#17115=LINE ( 'NONE', #9417, #49602 ) ;
#17119=ORIENTED_EDGE ( 'NONE', *, *, #8791, .T. ) ;
#17122=VERTEX_POINT ( 'NONE', #1683 ) ;
#17127=LINE ( 'NONE', #13517, #4538 ) ;
#17128=VERTEX_POINT ( 'NONE', #44995 ) ;
#17132=CARTESIAN_POINT ( 'NONE',  ( -64.99999999999815259, 16.00000000000000000, 65.00000000000000000 ) ) ;
#17133=ADVANCED_FACE ( 'NONE', ( #40433 ), #37365, .F. ) ;
#17138=PLANE ( 'NONE',  #45495 ) ;
#17163=CARTESIAN_POINT ( 'NONE',  ( -65.00000000000002842, 17.00000000000000000, -114.9999999999999858 ) ) ;
#17165=ORIENTED_EDGE ( 'NONE', *, *, #46483, .T. ) ;
#17168=CARTESIAN_POINT ( 'NONE',  ( -175.0000000000000000, 0.000000000000000000, -122.5000000000000000 ) ) ;
#17170=ORIENTED_EDGE ( 'NONE', *, *, #46152, .T. ) ;
#17184=ORIENTED_EDGE ( 'NONE', *, *, #49451, .F. ) ;
#17185=DIRECTION ( 'NONE',  ( -0.000000000000000000, -1.000000000000000000, -0.000000000000000000 ) ) ;
#17190=VECTOR ( 'NONE', #19743, 1000.000000000000000 ) ;
#17192=DIRECTION ( 'NONE',  ( 0.000000000000000000, 0.000000000000000000, 1.000000000000000000 ) ) ;
#17195=VECTOR ( 'NONE', #19032, 1000.000000000000000 ) ;
#17201=EDGE_CURVE ( 'NONE', #5410, #42631, #10390, .T. ) ;
#17204=ORIENTED_EDGE ( 'NONE', *, *, #13890, .F. ) ;
#17209=DIRECTION ( 'NONE',  ( 0.000000000000000000, 0.000000000000000000, -1.000000000000000000 ) ) ;
#17225=FACE_OUTER_BOUND ( 'NONE', #31455, .T. ) ;
#17226=ORIENTED_EDGE ( 'NONE', *, *, #33700, .F. ) ;
#17244=VERTEX_POINT ( 'NONE', #10629 ) ;
#17248=LINE ( 'NONE', #9049, #7387 ) ;
#17249=LINE ( 'NONE', #17497, #21825 ) ;
#17251=PLANE ( 'NONE',  #13706 ) ;
#17260=PLANE ( 'NONE',  #9329 ) ;
#17264=VECTOR ( 'NONE', #45830, 1000.000000000000000 ) ;
#17265=EDGE_LOOP ( 'NONE', ( #41646, #19848, #50387, #39155 ) ) ;
#17266=DIRECTION ( 'NONE',  ( -0.000000000000000000, -0.000000000000000000, -1.000000000000000000 ) ) ;
#17268=CARTESIAN_POINT ( 'NONE',  ( 35.00000000000061107, 17.00000000000000000, -54.99999999999999289 ) ) ;
#17272=CARTESIAN_POINT ( 'NONE',  ( -164.9999999999997442, 17.00000000000000000, -60.00000000000000000 ) ) ;
#17273=EDGE_LOOP ( 'NONE', ( #3198, #9953, #28796, #42069 ) ) ;
#17278=AXIS2_PLACEMENT_3D ( 'NONE', #44386, #2070, #13351 ) ;
#17286=CARTESIAN_POINT ( 'NONE',  ( -69.99999999999816680, 17.00000000000000000, 90.00000000000000000 ) ) ;
#17296=ADVANCED_FACE ( 'NONE', ( #41938 ), #46252, .F. ) ;
#17309=DIRECTION ( 'NONE',  ( -0.000000000000000000, -1.000000000000000000, -0.000000000000000000 ) ) ;
#17321=DIRECTION ( 'NONE',  ( 0.000000000000000000, 0.000000000000000000, 1.000000000000000000 ) ) ;
#17334=DIRECTION ( 'NONE',  ( 0.000000000000000000, 0.000000000000000000, 1.000000000000000000 ) ) ;
#17345=DIRECTION ( 'NONE',  ( 0.000000000000000000, -1.000000000000000000, 0.000000000000000000 ) ) ;
#17349=ADVANCED_FACE ( 'NONE', ( #10885 ), #38103, .F. ) ;
#17354=EDGE_CURVE ( 'NONE', #42166, #39210, #20102, .T. ) ;
#17361=VECTOR ( 'NONE', #18503, 1000.000000000000000 ) ;
#17368=AXIS2_PLACEMENT_3D ( 'NONE', #50604, #27574, #19350 ) ;
#17373=ORIENTED_EDGE ( 'NONE', *, *, #33766, .T. ) ;
#17374=CARTESIAN_POINT ( 'NONE',  ( 130.0000000000021032, 17.00000000000000000, 115.0000000000000142 ) ) ;
#17375=EDGE_LOOP ( 'NONE', ( #9909, #26028, #19517, #39259 ) ) ;
#17393=VECTOR ( 'NONE', #24836, 1000.000000000000000 ) ;
#17394=ORIENTED_EDGE ( 'NONE', *, *, #34464, .F. ) ;
#17408=LINE ( 'NONE', #40259, #37165 ) ;
#17431=LINE ( 'NONE', #13813, #49666 ) ;
#17432=CARTESIAN_POINT ( 'NONE',  ( -14.99999999999876366, 17.00000000000000000, 30.00000000000000000 ) ) ;
#17440=ORIENTED_EDGE ( 'NONE', *, *, #7340, .F. ) ;
#17449=DIRECTION ( 'NONE',  ( -0.000000000000000000, -1.000000000000000000, -0.000000000000000000 ) ) ;
#17451=PRODUCT_DEFINITION ( 'UNKNOWN', '', #11918, #4202 ) ;
#17455=DIRECTION ( 'NONE',  ( 0.000000000000000000, 0.000000000000000000, 1.000000000000000000 ) ) ;
#17460=CARTESIAN_POINT ( 'NONE',  ( -64.99999999999877787, 16.00000000000000000, 30.00000000000000000 ) ) ;
#17466=ORIENTED_EDGE ( 'NONE', *, *, #28847, .T. ) ;
#17469=DIRECTION ( 'NONE',  ( 1.000000000000000000, 0.000000000000000000, 0.000000000000000000 ) ) ;
#17471=PLANE ( 'NONE',  #28211 ) ;
#17475=CARTESIAN_POINT ( 'NONE',  ( -14.99999999999876366, 17.00000000000000000, 5.000000000000004441 ) ) ;
#17480=CARTESIAN_POINT ( 'NONE',  ( -19.99999999999940670, 17.00000000000000000, -54.99999999999999289 ) ) ;
#17494=EDGE_LOOP ( 'NONE', ( #45934, #1920, #10030, #608 ) ) ;
#17496=EDGE_CURVE ( 'NONE', #20578, #27386, #13667, .T. ) ;
#17497=CARTESIAN_POINT ( 'NONE',  ( 164.9999999999999716, 17.00000000000000000, -30.00000000000001421 ) ) ;
#17508=CARTESIAN_POINT ( 'NONE',  ( -19.99999999999815969, 17.00000000000000000, 90.00000000000000000 ) ) ;
#17509=VECTOR ( 'NONE', #7438, 1000.000000000000000 ) ;
#17539=EDGE_CURVE ( 'NONE', #16006, #31946, #43950, .T. ) ;
#17542=LINE ( 'NONE', #33215, #9895 ) ;
#17562=CARTESIAN_POINT ( 'NONE',  ( -115.0000000000000284, 17.00000000000000000, -114.9999999999999858 ) ) ;
#17577=AXIS2_PLACEMENT_3D ( 'NONE', #5181, #16990, #36006 ) ;
#17586=EDGE_CURVE ( 'NONE', #25002, #43342, #40625, .T. ) ;
#17589=CARTESIAN_POINT ( 'NONE',  ( -164.9999999999981526, 17.00000000000000000, 90.00000000000000000 ) ) ;
#17590=CARTESIAN_POINT ( 'NONE',  ( -119.9999999999990905, 16.00000000000000000, -24.99999999999999289 ) ) ;
#17591=DIRECTION ( 'NONE',  ( -0.000000000000000000, -0.000000000000000000, -1.000000000000000000 ) ) ;
#17596=AXIS2_PLACEMENT_3D ( 'NONE', #6415, #6925, #34387 ) ;
#17599=LINE ( 'NONE', #6556, #49522 ) ;
#17602=ORIENTED_EDGE ( 'NONE', *, *, #5113, .T. ) ;
#17622=ORIENTED_EDGE ( 'NONE', *, *, #24988, .T. ) ;
#17623=EDGE_LOOP ( 'NONE', ( #21089, #47045, #21870, #39460 ) ) ;
#17628=EDGE_CURVE ( 'NONE', #14555, #23499, #42113, .T. ) ;
#17634=CARTESIAN_POINT ( 'NONE',  ( 135.0000000000019043, 17.00000000000000000, 90.00000000000000000 ) ) ;
#17651=PLANE ( 'NONE',  #36117 ) ;
#17655=VERTEX_POINT ( 'NONE', #30329 ) ;
#17660=ORIENTED_EDGE ( 'NONE', *, *, #41934, .T. ) ;
#17661=CARTESIAN_POINT ( 'NONE',  ( -15.00000000000001421, 17.00000000000000000, -90.00000000000000000 ) ) ;
#17663=ORIENTED_EDGE ( 'NONE', *, *, #28332, .F. ) ;
#17670=VECTOR ( 'NONE', #11128, 1000.000000000000000 ) ;
#17671=ORIENTED_EDGE ( 'NONE', *, *, #5485, .T. ) ;
#17676=DIRECTION ( 'NONE',  ( 0.000000000000000000, -1.000000000000000000, 0.000000000000000000 ) ) ;
#17679=CARTESIAN_POINT ( 'NONE',  ( 0.000000000000000000, 17.00000000000000000, 0.000000000000000000 ) ) ;
#17687=ORIENTED_EDGE ( 'NONE', *, *, #49405, .F. ) ;
#17690=DIRECTION ( 'NONE',  ( -1.000000000000000000, -0.000000000000000000, -0.000000000000000000 ) ) ;
#17693=VECTOR ( 'NONE', #46846, 1000.000000000000000 ) ;
#17702=EDGE_CURVE ( 'NONE', #156, #3329, #2608, .T. ) ;
#17715=CARTESIAN_POINT ( 'NONE',  ( -164.9999999999987779, 17.00000000000000000, 5.000000000000004441 ) ) ;
#17719=DIRECTION ( 'NONE',  ( 1.000000000000000000, 0.000000000000000000, 0.000000000000000000 ) ) ;
#17720=VECTOR ( 'NONE', #6575, 1000.000000000000000 ) ;
#17722=DIRECTION ( 'NONE',  ( -0.000000000000000000, -0.000000000000000000, -1.000000000000000000 ) ) ;
#17726=VERTEX_POINT ( 'NONE', #38042 ) ;
#17730=ADVANCED_FACE ( 'NONE', ( #18515 ), #49770, .F. ) ;
#17734=CARTESIAN_POINT ( 'NONE',  ( -119.9999999999990905, 17.00000000000000000, -24.99999999999999289 ) ) ;
#17740=CARTESIAN_POINT ( 'NONE',  ( 164.9999999999999716, 16.00000000000000000, 60.00000000000000000 ) ) ;
#17742=ORIENTED_EDGE ( 'NONE', *, *, #17354, .T. ) ;
#17743=ORIENTED_EDGE ( 'NONE', *, *, #14632, .F. ) ;
#17750=ORIENTED_EDGE ( 'NONE', *, *, #17069, .F. ) ;
#17759=ORIENTED_EDGE ( 'NONE', *, *, #36924, .F. ) ;
#17767=AXIS2_PLACEMENT_3D ( 'NONE', #21918, #41410, #42403 ) ;
#17773=ADVANCED_FACE ( 'NONE', ( #26980 ), #31615, .F. ) ;
#17775=DIRECTION ( 'NONE',  ( 1.000000000000000000, 0.000000000000000000, -0.000000000000000000 ) ) ;
#17776=VERTEX_POINT ( 'NONE', #19271 ) ;
#17786=ORIENTED_EDGE ( 'NONE', *, *, #26806, .T. ) ;
#17793=CARTESIAN_POINT ( 'NONE',  ( 35.00000000000122213, 17.00000000000000000, 5.000000000000004441 ) ) ;
#17801=VERTEX_POINT ( 'NONE', #23126 ) ;
#17809=CARTESIAN_POINT ( 'NONE',  ( 0.000000000000000000, 17.00000000000000000, 0.000000000000000000 ) ) ;
#17811=VERTEX_POINT ( 'NONE', #15950 ) ;
#17813=DIRECTION ( 'NONE',  ( 0.000000000000000000, -1.000000000000000000, 0.000000000000000000 ) ) ;
#17814=CARTESIAN_POINT ( 'NONE',  ( -165.0000000000000284, 16.00000000000000000, 115.0000000000000142 ) ) ;
#17819=ORIENTED_EDGE ( 'NONE', *, *, #4856, .F. ) ;
#17824=EDGE_CURVE ( 'NONE', #23499, #3216, #19520, .T. ) ;
#17827=ORIENTED_EDGE ( 'NONE', *, *, #34684, .F. ) ;
#17832=FACE_OUTER_BOUND ( 'NONE', #46282, .T. ) ;
#17836=CARTESIAN_POINT ( 'NONE',  ( 35.00000000000061107, 16.00000000000000000, -54.99999999999999289 ) ) ;
#17843=PLANE ( 'NONE',  #9275 ) ;
#17848=EDGE_LOOP ( 'NONE', ( #20087, #16351, #7662, #28529 ) ) ;
#17849=ORIENTED_EDGE ( 'NONE', *, *, #246, .F. ) ;
#17850=DIRECTION ( 'NONE',  ( -0.000000000000000000, -1.000000000000000000, -0.000000000000000000 ) ) ;
#17852=ORIENTED_EDGE ( 'NONE', *, *, #3841, .F. ) ;
#17875=AXIS2_PLACEMENT_3D ( 'NONE', #48516, #18005, #40624 ) ;
#17877=CARTESIAN_POINT ( 'NONE',  ( 0.000000000000000000, 17.00000000000000000, 0.000000000000000000 ) ) ;
#17885=FACE_OUTER_BOUND ( 'NONE', #42745, .T. ) ;
#17890=LINE ( 'NONE', #1759, #19921 ) ;
#17905=CARTESIAN_POINT ( 'NONE',  ( 129.9999999999999432, 17.00000000000000000, -114.9999999999999858 ) ) ;
#17920=ORIENTED_EDGE ( 'NONE', *, *, #35426, .F. ) ;
#17922=LINE ( 'NONE', #22292, #41001 ) ;
#17923=DIRECTION ( 'NONE',  ( 1.000000000000000000, 0.000000000000000000, 0.000000000000000000 ) ) ;
#17930=VERTEX_POINT ( 'NONE', #21052 ) ;
#17933=CARTESIAN_POINT ( 'NONE',  ( 0.000000000000000000, 17.00000000000000000, 0.000000000000000000 ) ) ;
#17962=( NAMED_UNIT ( * ) PLANE_ANGLE_UNIT ( ) SI_UNIT ( $, .RADIAN. ) );
#17967=LINE ( 'NONE', #33644, #49899 ) ;
#17968=DIRECTION ( 'NONE',  ( -0.000000000000000000, -1.000000000000000000, -0.000000000000000000 ) ) ;
#17972=EDGE_CURVE ( 'NONE', #35976, #22721, #14606, .T. ) ;
#17979=VECTOR ( 'NONE', #47282, 1000.000000000000000 ) ;
#17980=ORIENTED_EDGE ( 'NONE', *, *, #766, .T. ) ;
#17996=ORIENTED_EDGE ( 'NONE', *, *, #246, .T. ) ;
#18005=DIRECTION ( 'NONE',  ( -1.000000000000000000, 0.000000000000000000, 0.000000000000000000 ) ) ;
#18010=CARTESIAN_POINT ( 'NONE',  ( -164.9999999999978400, 17.00000000000000000, 95.00000000000000000 ) ) ;
#18012=ORIENTED_EDGE ( 'NONE', *, *, #28332, .T. ) ;
#18015=CARTESIAN_POINT ( 'NONE',  ( 0.000000000000000000, 17.00000000000000000, 0.000000000000000000 ) ) ;
#18017=VECTOR ( 'NONE', #32266, 1000.000000000000000 ) ;
#18039=ORIENTED_EDGE ( 'NONE', *, *, #30939, .F. ) ;
#18044=EDGE_CURVE ( 'NONE', #25202, #10490, #6404, .T. ) ;
#18047=DIRECTION ( 'NONE',  ( -0.000000000000000000, -1.000000000000000000, -0.000000000000000000 ) ) ;
#18049=DIRECTION ( 'NONE',  ( 0.000000000000000000, 0.000000000000000000, 1.000000000000000000 ) ) ;
#18051=EDGE_CURVE ( 'NONE', #49743, #46654, #49463, .T. ) ;
#18055=LINE ( 'NONE', #17562, #4567 ) ;
#18062=DIRECTION ( 'NONE',  ( 0.000000000000000000, 0.000000000000000000, 1.000000000000000000 ) ) ;
#18069=CARTESIAN_POINT ( 'NONE',  ( 0.000000000000000000, 17.00000000000000000, 0.000000000000000000 ) ) ;
#18072=PLANE ( 'NONE',  #21129 ) ;
#18073=CARTESIAN_POINT ( 'NONE',  ( 30.00000000000187228, 17.00000000000000000, 65.00000000000000000 ) ) ;
#18084=LINE ( 'NONE', #17460, #24642 ) ;
#18092=AXIS2_PLACEMENT_3D ( 'NONE', #21762, #49669, #3008 ) ;
#18096=FACE_OUTER_BOUND ( 'NONE', #23563, .T. ) ;
#18099=VECTOR ( 'NONE', #24797, 1000.000000000000000 ) ;
#18101=FACE_OUTER_BOUND ( 'NONE', #5286, .T. ) ;
#18108=ORIENTED_EDGE ( 'NONE', *, *, #29071, .F. ) ;
#18110=ORIENTED_EDGE ( 'NONE', *, *, #12416, .F. ) ;
#18133=AXIS2_PLACEMENT_3D ( 'NONE', #45980, #31399, #27549 ) ;
#18148=CARTESIAN_POINT ( 'NONE',  ( -165.0000000000000284, 15.00000000000000000, 115.0000000000000142 ) ) ;
#18151=DIRECTION ( 'NONE',  ( 1.000000000000000000, 0.000000000000000000, 0.000000000000000000 ) ) ;
#18152=FACE_OUTER_BOUND ( 'NONE', #31568, .T. ) ;
#18158=EDGE_LOOP ( 'NONE', ( #49997, #14694, #35173, #16416 ) ) ;
#18186=FACE_BOUND ( 'NONE', #11350, .T. ) ;
#18188=EDGE_LOOP ( 'NONE', ( #2959, #6438, #12611, #27559 ) ) ;
#18189=DIRECTION ( 'NONE',  ( 0.000000000000000000, 0.000000000000000000, 1.000000000000000000 ) ) ;
#18193=DIRECTION ( 'NONE',  ( 0.000000000000000000, 0.000000000000000000, 1.000000000000000000 ) ) ;
#18199=CARTESIAN_POINT ( 'NONE',  ( -64.99999999999877787, 17.00000000000000000, 30.00000000000000000 ) ) ;
#18217=DIRECTION ( 'NONE',  ( 1.000000000000000000, 0.000000000000000000, 0.000000000000000000 ) ) ;
#18221=VECTOR ( 'NONE', #36403, 1000.000000000000000 ) ;
#18225=LINE ( 'NONE', #18725, #19170 ) ;
#18253=LINE ( 'NONE', #6975, #19486 ) ;
#18258=ORIENTED_EDGE ( 'NONE', *, *, #27728, .F. ) ;
#18260=AXIS2_PLACEMENT_3D ( 'NONE', #17933, #41303, #5896 ) ;
#18262=CARTESIAN_POINT ( 'NONE',  ( -69.99999999999972999, 16.00000000000000000, -84.99999999999998579 ) ) ;
#18265=ADVANCED_FACE ( 'NONE', ( #17832 ), #21942, .F. ) ;
#18271=LINE ( 'NONE', #6246, #17195 ) ;
#18284=ADVANCED_FACE ( 'NONE', ( #28886 ), #5280, .F. ) ;
#18293=DIRECTION ( 'NONE',  ( 0.000000000000000000, 0.000000000000000000, 1.000000000000000000 ) ) ;
#18295=VECTOR ( 'NONE', #40063, 1000.000000000000000 ) ;
#18299=CARTESIAN_POINT ( 'NONE',  ( 85.00000000000123634, 17.00000000000000000, 30.00000000000000000 ) ) ;
#18300=CARTESIAN_POINT ( 'NONE',  ( -14.99999999999782041, 16.00000000000000000, 95.00000000000000000 ) ) ;
#18303=VERTEX_POINT ( 'NONE', #40938 ) ;
#18304=CARTESIAN_POINT ( 'NONE',  ( 80.00000000000153477, 17.00000000000000000, 35.00000000000000000 ) ) ;
#18329=VECTOR ( 'NONE', #36417, 1000.000000000000000 ) ;
#18330=CARTESIAN_POINT ( 'NONE',  ( 135.0000000000009663, 16.00000000000000000, 0.000000000000000000 ) ) ;
#18334=EDGE_LOOP ( 'NONE', ( #33869, #40052, #27854, #2517 ) ) ;
#18344=CARTESIAN_POINT ( 'NONE',  ( 35.00000000000122213, 17.00000000000000000, 30.00000000000000000 ) ) ;
#18345=DIRECTION ( 'NONE',  ( 1.000000000000000000, -0.000000000000000000, 0.000000000000000000 ) ) ;
#18364=CARTESIAN_POINT ( 'NONE',  ( 130.0000000000012221, 17.00000000000000000, 5.000000000000004441 ) ) ;
#18370=EDGE_CURVE ( 'NONE', #46071, #12379, #41687, .T. ) ;
#18374=EDGE_LOOP ( 'NONE', ( #39664, #12948, #43163, #4105 ) ) ;
#18396=LINE ( 'NONE', #34077, #38127 ) ;
#18403=VECTOR ( 'NONE', #40153, 1000.000000000000000 ) ;
#18406=PLANE ( 'NONE',  #18092 ) ;
#18412=VERTEX_POINT ( 'NONE', #31687 ) ;
#18413=ORIENTED_EDGE ( 'NONE', *, *, #4974, .F. ) ;
#18416=ORIENTED_EDGE ( 'NONE', *, *, #48342, .T. ) ;
#18439=FACE_BOUND ( 'NONE', #33715, .T. ) ;
#18450=LINE ( 'NONE', #21299, #49439 ) ;
#18455=LINE ( 'NONE', #37984, #40484 ) ;
#18457=VERTEX_POINT ( 'NONE', #47277 ) ;
#18462=CARTESIAN_POINT ( 'NONE',  ( 130.0000000000018474, 17.00000000000000000, 65.00000000000000000 ) ) ;
#18466=VECTOR ( 'NONE', #33460, 1000.000000000000000 ) ;
#18468=ORIENTED_EDGE ( 'NONE', *, *, #24988, .F. ) ;
#18477=ORIENTED_EDGE ( 'NONE', *, *, #21582, .F. ) ;
#18481=CARTESIAN_POINT ( 'NONE',  ( 80.00000000000061107, 17.00000000000000000, -54.99999999999999289 ) ) ;
#18482=AXIS2_PLACEMENT_3D ( 'NONE', #47121, #27925, #27416 ) ;
#18484=DIRECTION ( 'NONE',  ( -0.000000000000000000, -1.000000000000000000, -0.000000000000000000 ) ) ;
#18486=ORIENTED_EDGE ( 'NONE', *, *, #47449, .F. ) ;
#18489=DIRECTION ( 'NONE',  ( 0.000000000000000000, 0.000000000000000000, 1.000000000000000000 ) ) ;
#18503=DIRECTION ( 'NONE',  ( -0.000000000000000000, -1.000000000000000000, -0.000000000000000000 ) ) ;
#18515=FACE_OUTER_BOUND ( 'NONE', #554, .T. ) ;
#18516=DIRECTION ( 'NONE',  ( -1.000000000000000000, -0.000000000000000000, -0.000000000000000000 ) ) ;
#18518=VECTOR ( 'NONE', #44431, 1000.000000000000000 ) ;
#18524=VECTOR ( 'NONE', #46468, 1000.000000000000000 ) ;
#18532=EDGE_LOOP ( 'NONE', ( #48537, #4391, #41619, #978 ) ) ;
#18533=VECTOR ( 'NONE', #37771, 1000.000000000000000 ) ;
#18537=AXIS2_PLACEMENT_3D ( 'NONE', #28802, #41102, #9296 ) ;
#18546=EDGE_LOOP ( 'NONE', ( #768, #40085, #46446, #44777 ) ) ;
#18548=LINE ( 'NONE', #26513, #5431 ) ;
#18550=VECTOR ( 'NONE', #5837, 1000.000000000000000 ) ;
#18552=ORIENTED_EDGE ( 'NONE', *, *, #49599, .F. ) ;
#18554=ORIENTED_EDGE ( 'NONE', *, *, #47784, .T. ) ;
#18558=VERTEX_POINT ( 'NONE', #36800 ) ;
#18559=ORIENTED_EDGE ( 'NONE', *, *, #40872, .F. ) ;
#18562=DIRECTION ( 'NONE',  ( -0.000000000000000000, -0.000000000000000000, -1.000000000000000000 ) ) ;
#18564=DIRECTION ( 'NONE',  ( -0.000000000000000000, -1.000000000000000000, -0.000000000000000000 ) ) ;
#18572=DIRECTION ( 'NONE',  ( 0.000000000000000000, 0.000000000000000000, 1.000000000000000000 ) ) ;
#18574=CARTESIAN_POINT ( 'NONE',  ( 30.00000000000187228, 17.00000000000000000, 90.00000000000000000 ) ) ;
#18579=DIRECTION ( 'NONE',  ( -0.000000000000000000, -0.000000000000000000, -1.000000000000000000 ) ) ;
#18580=EDGE_CURVE ( 'NONE', #39210, #10318, #48786, .T. ) ;
#18591=DIRECTION ( 'NONE',  ( -0.000000000000000000, -0.000000000000000000, 1.000000000000000000 ) ) ;
#18592=CARTESIAN_POINT ( 'NONE',  ( -14.99999999999937472, 17.00000000000000000, -54.99999999999999289 ) ) ;
#18605=ORIENTED_EDGE ( 'NONE', *, *, #23099, .T. ) ;
#18606=ORIENTED_EDGE ( 'NONE', *, *, #29930, .F. ) ;
#18653=CARTESIAN_POINT ( 'NONE',  ( -19.99999999999940670, 16.00000000000000000, -30.00000000000000000 ) ) ;
#18655=CARTESIAN_POINT ( 'NONE',  ( 164.9999999999999716, 17.00000000000000000, 29.99999999999999289 ) ) ;
#18659=DIRECTION ( 'NONE',  ( -0.000000000000000000, -1.000000000000000000, -0.000000000000000000 ) ) ;
#18660=ORIENTED_EDGE ( 'NONE', *, *, #9375, .F. ) ;
#18668=LINE ( 'NONE', #150, #6763 ) ;
#18670=PLANE ( 'NONE',  #16967 ) ;
#18672=CARTESIAN_POINT ( 'NONE',  ( 85.00000000000090949, 16.00000000000000000, -24.99999999999999289 ) ) ;
#18684=EDGE_LOOP ( 'NONE', ( #31146, #8954, #30393, #14014 ) ) ;
#18685=CARTESIAN_POINT ( 'NONE',  ( -14.99999999999906919, 17.00000000000000000, -24.99999999999999289 ) ) ;
#18691=DIRECTION ( 'NONE',  ( -1.000000000000000000, -0.000000000000000000, -0.000000000000000000 ) ) ;
#18700=CARTESIAN_POINT ( 'NONE',  ( -69.99999999999847944, 17.00000000000000000, 35.00000000000000000 ) ) ;
#18702=ORIENTED_EDGE ( 'NONE', *, *, #38119, .T. ) ;
#18707=LINE ( 'NONE', #30280, #27265 ) ;
#18720=PLANE ( 'NONE',  #19139 ) ;
#18721=ORIENTED_EDGE ( 'NONE', *, *, #25549, .F. ) ;
#18725=CARTESIAN_POINT ( 'NONE',  ( -164.9999999999987779, 17.00000000000000000, 5.000000000000004441 ) ) ;
#18731=VERTEX_POINT ( 'NONE', #18262 ) ;
#18742=VECTOR ( 'NONE', #39182, 1000.000000000000000 ) ;
#18748=EDGE_LOOP ( 'NONE', ( #41457, #35199, #12238, #18554 ) ) ;
#18753=ADVANCED_FACE ( 'NONE', ( #570 ), #47210, .F. ) ;
#18755=AXIS2_PLACEMENT_3D ( 'NONE', #23886, #27983, #36208 ) ;
#18756=ORIENTED_EDGE ( 'NONE', *, *, #37053, .F. ) ;
#18764=FACE_OUTER_BOUND ( 'NONE', #30410, .T. ) ;
#18767=ORIENTED_EDGE ( 'NONE', *, *, #6251, .T. ) ;
#18779=EDGE_CURVE ( 'NONE', #20500, #43501, #817, .T. ) ;
#18792=VECTOR ( 'NONE', #18591, 1000.000000000000000 ) ;
#18805=ORIENTED_EDGE ( 'NONE', *, *, #6195, .F. ) ;
#18806=ORIENTED_EDGE ( 'NONE', *, *, #43586, .T. ) ;
#18813=VECTOR ( 'NONE', #24129, 1000.000000000000000 ) ;
#18817=AXIS2_PLACEMENT_3D ( 'NONE', #43840, #20249, #21007 ) ;
#18820=CARTESIAN_POINT ( 'NONE',  ( -14.99999999999906919, 17.00000000000000000, -24.99999999999999289 ) ) ;
#18823=VECTOR ( 'NONE', #34010, 1000.000000000000000 ) ;
#18827=VECTOR ( 'NONE', #2285, 1000.000000000000000 ) ;
#18829=PLANE ( 'NONE',  #32657 ) ;
#18834=DIRECTION ( 'NONE',  ( 0.000000000000000000, -0.000000000000000000, -1.000000000000000000 ) ) ;
#18847=AXIS2_PLACEMENT_3D ( 'NONE', #47972, #17469, #40575 ) ;
#18849=ORIENTED_EDGE ( 'NONE', *, *, #35288, .F. ) ;
#18855=ORIENTED_EDGE ( 'NONE', *, *, #21435, .T. ) ;
#18857=VECTOR ( 'NONE', #29209, 1000.000000000000000 ) ;
#18877=DIRECTION ( 'NONE',  ( 0.000000000000000000, 0.000000000000000000, -1.000000000000000000 ) ) ;
#18880=CARTESIAN_POINT ( 'NONE',  ( 135.0000000000019043, 17.00000000000000000, 65.00000000000000000 ) ) ;
#18883=LINE ( 'NONE', #45570, #43645 ) ;
#18890=VECTOR ( 'NONE', #32318, 1000.000000000000000 ) ;
#18913=ORIENTED_EDGE ( 'NONE', *, *, #50536, .T. ) ;
#18916=DIRECTION ( 'NONE',  ( -1.000000000000000000, -0.000000000000000000, -0.000000000000000000 ) ) ;
#18923=DIRECTION ( 'NONE',  ( 1.000000000000000000, 0.000000000000000000, 0.000000000000000000 ) ) ;
#18926=ORIENTED_EDGE ( 'NONE', *, *, #19528, .F. ) ;
#18940=DIRECTION ( 'NONE',  ( -1.000000000000000000, 0.000000000000000000, -0.000000000000000000 ) ) ;
#18947=LINE ( 'NONE', #30779, #1880 ) ;
#18967=ADVANCED_FACE ( 'NONE', ( #44385 ), #40564, .F. ) ;
#18977=ORIENTED_EDGE ( 'NONE', *, *, #1090, .F. ) ;
#18978=LINE ( 'NONE', #19483, #38004 ) ;
#18987=ORIENTED_EDGE ( 'NONE', *, *, #19527, .F. ) ;
#18988=LINE ( 'NONE', #42345, #42302 ) ;
#18998=ORIENTED_EDGE ( 'NONE', *, *, #25509, .T. ) ;
#19003=VECTOR ( 'NONE', #27970, 1000.000000000000000 ) ;
#19015=DIRECTION ( 'NONE',  ( 0.000000000000000000, 0.000000000000000000, -1.000000000000000000 ) ) ;
#19028=VECTOR ( 'NONE', #45054, 1000.000000000000000 ) ;
#19032=DIRECTION ( 'NONE',  ( -1.000000000000000000, -0.000000000000000000, -0.000000000000000000 ) ) ;
#19033=VECTOR ( 'NONE', #37595, 1000.000000000000000 ) ;
#19044=ORIENTED_EDGE ( 'NONE', *, *, #30270, .F. ) ;
#19059=CARTESIAN_POINT ( 'NONE',  ( -64.99999999999783995, 16.00000000000000000, 95.00000000000000000 ) ) ;
#19067=VERTEX_POINT ( 'NONE', #41318 ) ;
#19070=LINE ( 'NONE', #42416, #41250 ) ;
#19071=EDGE_LOOP ( 'NONE', ( #35562, #43340, #44295, #13552 ) ) ;
#19074=VECTOR ( 'NONE', #28397, 1000.000000000000000 ) ;
#19090=EDGE_CURVE ( 'NONE', #24017, #7557, #45387, .T. ) ;
#19096=ADVANCED_FACE ( 'NONE', ( #49722 ), #42065, .F. ) ;
#19097=VERTEX_POINT ( 'NONE', #23848 ) ;
#19098=LINE ( 'NONE', #19616, #49948 ) ;
#19102=LINE ( 'NONE', #18592, #38123 ) ;
#19127=VERTEX_POINT ( 'NONE', #27946 ) ;
#19139=AXIS2_PLACEMENT_3D ( 'NONE', #3331, #14894, #49738 ) ;
#19140=DIRECTION ( 'NONE',  ( -1.000000000000000000, -0.000000000000000000, -0.000000000000000000 ) ) ;
#19145=LINE ( 'NONE', #21993, #39575 ) ;
#19146=CARTESIAN_POINT ( 'NONE',  ( -14.99999999999937472, 16.00000000000000000, -30.00000000000000000 ) ) ;
#19147=VECTOR ( 'NONE', #18659, 1000.000000000000000 ) ;
#19150=VERTEX_POINT ( 'NONE', #19986 ) ;
#19151=CARTESIAN_POINT ( 'NONE',  ( 30.00000000000123279, 17.00000000000000000, 5.000000000000004441 ) ) ;
#19157=ORIENTED_EDGE ( 'NONE', *, *, #28787, .F. ) ;
#19158=CARTESIAN_POINT ( 'NONE',  ( 35.00000000000122213, 17.00000000000000000, 5.000000000000004441 ) ) ;
#19162=CARTESIAN_POINT ( 'NONE',  ( 135.0000000000019043, 17.00000000000000000, 90.00000000000000000 ) ) ;
#19170=VECTOR ( 'NONE', #49496, 1000.000000000000000 ) ;
#19174=CARTESIAN_POINT ( 'NONE',  ( 80.00000000000153477, 16.00000000000000000, 35.00000000000000000 ) ) ;
#19189=PLANE ( 'NONE',  #44650 ) ;
#19193=AXIS2_PLACEMENT_3D ( 'NONE', #29570, #6232, #44935 ) ;
#19212=DIRECTION ( 'NONE',  ( 0.000000000000000000, -1.000000000000000000, 0.000000000000000000 ) ) ;
#19230=VECTOR ( 'NONE', #49671, 1000.000000000000000 ) ;
#19233=DIRECTION ( 'NONE',  ( 1.000000000000000000, 0.000000000000000000, -2.312964634635843537E-16 ) ) ;
#19243=EDGE_LOOP ( 'NONE', ( #49046, #22638, #44862, #8063 ) ) ;
#19250=EDGE_CURVE ( 'NONE', #7557, #21400, #7690, .T. ) ;
#19259=EDGE_CURVE ( 'NONE', #14478, #14555, #15126, .T. ) ;
#19260=EDGE_CURVE ( 'NONE', #23917, #39423, #11791, .T. ) ;
#19266=EDGE_CURVE ( 'NONE', #41913, #14475, #34904, .T. ) ;
#19271=CARTESIAN_POINT ( 'NONE',  ( -119.9999999999981668, 17.00000000000000000, 65.00000000000000000 ) ) ;
#19274=LINE ( 'NONE', #11848, #45399 ) ;
#19281=DIRECTION ( 'NONE',  ( -0.000000000000000000, -0.000000000000000000, -1.000000000000000000 ) ) ;
#19290=VECTOR ( 'NONE', #41287, 1000.000000000000000 ) ;
#19293=CARTESIAN_POINT ( 'NONE',  ( -114.9999999999981526, 17.00000000000000000, 65.00000000000000000 ) ) ;
#19309=DIRECTION ( 'NONE',  ( 0.000000000000000000, 0.000000000000000000, -1.000000000000000000 ) ) ;
#19324=LINE ( 'NONE', #18299, #38210 ) ;
#19325=CARTESIAN_POINT ( 'NONE',  ( -119.9999999999987921, 17.00000000000000000, 5.000000000000004441 ) ) ;
#19329=ORIENTED_EDGE ( 'NONE', *, *, #42198, .T. ) ;
#19332=ORIENTED_EDGE ( 'NONE', *, *, #44836, .T. ) ;
#19341=FACE_OUTER_BOUND ( 'NONE', #45169, .T. ) ;
#19350=DIRECTION ( 'NONE',  ( 0.000000000000000000, -0.000000000000000000, -1.000000000000000000 ) ) ;
#19353=CARTESIAN_POINT ( 'NONE',  ( -114.9999999999984652, 17.00000000000000000, 35.00000000000000000 ) ) ;
#19359=VECTOR ( 'NONE', #16744, 1000.000000000000000 ) ;
#19360=DIRECTION ( 'NONE',  ( 1.000000000000000000, 0.000000000000000000, 0.000000000000000000 ) ) ;
#19362=CARTESIAN_POINT ( 'NONE',  ( 0.000000000000000000, 17.00000000000000000, 0.000000000000000000 ) ) ;
#19379=DIRECTION ( 'NONE',  ( -0.000000000000000000, -1.000000000000000000, -0.000000000000000000 ) ) ;
#19383=CARTESIAN_POINT ( 'NONE',  ( -19.99999999999971223, 17.00000000000000000, -84.99999999999998579 ) ) ;
#19386=EDGE_CURVE ( 'NONE', #30294, #45615, #28458, .T. ) ;
#19392=VERTEX_POINT ( 'NONE', #20490 ) ;
#19397=EDGE_CURVE ( 'NONE', #29367, #35690, #1756, .T. ) ;
#19402=FACE_OUTER_BOUND ( 'NONE', #18374, .T. ) ;
#19407=CARTESIAN_POINT ( 'NONE',  ( 0.000000000000000000, 17.00000000000000000, 0.000000000000000000 ) ) ;
#19410=EDGE_LOOP ( 'NONE', ( #45845, #28591, #29370, #7865 ) ) ;
#19412=CARTESIAN_POINT ( 'NONE',  ( -119.9999999999984652, 17.00000000000000000, 60.00000000000000000 ) ) ;
#19416=CARTESIAN_POINT ( 'NONE',  ( 79.99999999999997158, 17.00000000000000000, -114.9999999999999858 ) ) ;
#19426=ORIENTED_EDGE ( 'NONE', *, *, #12043, .F. ) ;
#19427=DIRECTION ( 'NONE',  ( 0.000000000000000000, 0.000000000000000000, 1.000000000000000000 ) ) ;
#19430=CARTESIAN_POINT ( 'NONE',  ( 30.00000000000153833, 16.00000000000000000, 35.00000000000000000 ) ) ;
#19440=DIRECTION ( 'NONE',  ( 0.000000000000000000, 0.000000000000000000, 1.000000000000000000 ) ) ;
#19448=ORIENTED_EDGE ( 'NONE', *, *, #38878, .T. ) ;
#19456=CARTESIAN_POINT ( 'NONE',  ( -64.99999999999815259, 17.00000000000000000, 65.00000000000000000 ) ) ;
#19458=LINE ( 'NONE', #34368, #10765 ) ;
#19460=CARTESIAN_POINT ( 'NONE',  ( 84.99999999999997158, 16.00000000000000000, -90.00000000000000000 ) ) ;
#19472=FACE_OUTER_BOUND ( 'NONE', #6571, .T. ) ;
#19483=CARTESIAN_POINT ( 'NONE',  ( -15.00000000000001421, 16.00000000000000000, -90.00000000000000000 ) ) ;
#19485=EDGE_CURVE ( 'NONE', #3719, #37447, #49155, .T. ) ;
#19486=VECTOR ( 'NONE', #2853, 1000.000000000000000 ) ;
#19497=ORIENTED_EDGE ( 'NONE', *, *, #20192, .F. ) ;
#19517=ORIENTED_EDGE ( 'NONE', *, *, #30408, .F. ) ;
#19520=LINE ( 'NONE', #51, #38975 ) ;
#19527=EDGE_CURVE ( 'NONE', #16028, #44556, #18396, .T. ) ;
#19528=EDGE_CURVE ( 'NONE', #32184, #41885, #42008, .T. ) ;
#19535=CARTESIAN_POINT ( 'NONE',  ( 135.0000000000021600, 17.00000000000000000, 115.0000000000000142 ) ) ;
#19539=DIRECTION ( 'NONE',  ( -1.000000000000000000, 0.000000000000000000, 0.000000000000000000 ) ) ;
#19561=DIRECTION ( 'NONE',  ( -1.000000000000000000, 0.000000000000000000, -0.000000000000000000 ) ) ;
#19565=AXIS2_PLACEMENT_3D ( 'NONE', #21357, #39880, #43948 ) ;
#19570=AXIS2_PLACEMENT_3D ( 'NONE', #20538, #1046, #16192 ) ;
#19580=DIRECTION ( 'NONE',  ( 0.000000000000000000, 0.000000000000000000, -1.000000000000000000 ) ) ;
#19586=LINE ( 'NONE', #3683, #32985 ) ;
#19589=DIRECTION ( 'NONE',  ( 0.000000000000000000, -1.000000000000000000, 0.000000000000000000 ) ) ;
#19593=LINE ( 'NONE', #14991, #26027 ) ;
#19596=VERTEX_POINT ( 'NONE', #7626 ) ;
#19604=LINE ( 'NONE', #11160, #3438 ) ;
#19610=PLANE ( 'NONE',  #24595 ) ;
#19612=ORIENTED_EDGE ( 'NONE', *, *, #21872, .T. ) ;
#19616=CARTESIAN_POINT ( 'NONE',  ( 35.00000000000028422, 17.00000000000000000, -84.99999999999998579 ) ) ;
#19625=EDGE_CURVE ( 'NONE', #27056, #41220, #44263, .T. ) ;
#19635=ORIENTED_EDGE ( 'NONE', *, *, #7340, .T. ) ;
#19641=VECTOR ( 'NONE', #28328, 1000.000000000000000 ) ;
#19649=AXIS2_PLACEMENT_3D ( 'NONE', #1035, #28487, #44599 ) ;
#19658=FACE_OUTER_BOUND ( 'NONE', #18748, .T. ) ;
#19660=LINE ( 'NONE', #11973, #5643 ) ;
#19661=DIRECTION ( 'NONE',  ( -0.000000000000000000, -0.000000000000000000, -1.000000000000000000 ) ) ;
#19664=DIRECTION ( 'NONE',  ( -0.000000000000000000, -1.000000000000000000, -0.000000000000000000 ) ) ;
#19668=EDGE_LOOP ( 'NONE', ( #27279, #2500, #35006, #19674 ) ) ;
#19674=ORIENTED_EDGE ( 'NONE', *, *, #1503, .F. ) ;
#19679=CARTESIAN_POINT ( 'NONE',  ( -114.9999999999984652, 17.00000000000000000, 35.00000000000000000 ) ) ;
#19680=AXIS2_PLACEMENT_3D ( 'NONE', #40926, #4763, #17321 ) ;
#19681=ORIENTED_EDGE ( 'NONE', *, *, #19625, .T. ) ;
#19682=CARTESIAN_POINT ( 'NONE',  ( -69.99999999999847944, 16.00000000000000000, 60.00000000000000000 ) ) ;
#19692=EDGE_CURVE ( 'NONE', #7457, #30535, #43774, .T. ) ;
#19700=DIRECTION ( 'NONE',  ( 0.000000000000000000, 0.000000000000000000, -1.000000000000000000 ) ) ;
#19706=LINE ( 'NONE', #12504, #47229 ) ;
#19708=ORIENTED_EDGE ( 'NONE', *, *, #4484, .F. ) ;
#19719=DIRECTION ( 'NONE',  ( 1.000000000000000000, 0.000000000000000000, 0.000000000000000000 ) ) ;
#19728=EDGE_CURVE ( 'NONE', #13070, #44903, #4794, .T. ) ;
#19743=DIRECTION ( 'NONE',  ( -6.938893903907222461E-16, -0.000000000000000000, -1.000000000000000000 ) ) ;
#19753=ORIENTED_EDGE ( 'NONE', *, *, #50522, .T. ) ;
#19790=CARTESIAN_POINT ( 'NONE',  ( -20.00000000000003197, 17.00000000000000000, -114.9999999999999858 ) ) ;
#19811=PLANE ( 'NONE',  #40176 ) ;
#19826=ADVANCED_FACE ( 'NONE', ( #8673 ), #47870, .F. ) ;
#19833=DIRECTION ( 'NONE',  ( 0.000000000000000000, 0.000000000000000000, -1.000000000000000000 ) ) ;
#19834=CARTESIAN_POINT ( 'NONE',  ( -64.99999999999846523, 17.00000000000000000, 35.00000000000000000 ) ) ;
#19848=ORIENTED_EDGE ( 'NONE', *, *, #42550, .F. ) ;
#19852=CARTESIAN_POINT ( 'NONE',  ( 130.0000000000012221, 17.00000000000000000, 5.000000000000004441 ) ) ;
#19857=DIRECTION ( 'NONE',  ( -1.000000000000000000, 0.000000000000000000, -0.000000000000000000 ) ) ;
#19860=DIRECTION ( 'NONE',  ( 0.000000000000000000, 0.000000000000000000, 1.000000000000000000 ) ) ;
#19872=ORIENTED_EDGE ( 'NONE', *, *, #44457, .T. ) ;
#19880=PLANE ( 'NONE',  #47826 ) ;
#19892=ORIENTED_EDGE ( 'NONE', *, *, #6719, .T. ) ;
#19894=CARTESIAN_POINT ( 'NONE',  ( 80.00000000000092371, 17.00000000000000000, -24.99999999999999289 ) ) ;
#19905=LINE ( 'NONE', #16826, #40783 ) ;
#19914=CARTESIAN_POINT ( 'NONE',  ( 135.0000000000003411, 17.00000000000000000, -84.99999999999998579 ) ) ;
#19921=VECTOR ( 'NONE', #41010, 1000.000000000000000 ) ;
#19925=VECTOR ( 'NONE', #25670, 1000.000000000000000 ) ;
#19934=VERTEX_POINT ( 'NONE', #1968 ) ;
#19940=CARTESIAN_POINT ( 'NONE',  ( 130.0000000000008811, 17.00000000000000000, -24.99999999999999289 ) ) ;
#19946=DIRECTION ( 'NONE',  ( 1.000000000000000000, 0.000000000000000000, -2.312964634635864737E-16 ) ) ;
#19948=PLANE ( 'NONE',  #34987 ) ;
#19962=VECTOR ( 'NONE', #44316, 1000.000000000000000 ) ;
#19971=CARTESIAN_POINT ( 'NONE',  ( -175.0000000000000000, 15.00000000000000000, -122.5000000000000000 ) ) ;
#19973=DIRECTION ( 'NONE',  ( 0.000000000000000000, 0.000000000000000000, -1.000000000000000000 ) ) ;
#19976=EDGE_CURVE ( 'NONE', #37483, #16843, #41973, .T. ) ;
#19979=VECTOR ( 'NONE', #32930, 1000.000000000000000 ) ;
#19980=DIRECTION ( 'NONE',  ( 0.000000000000000000, 0.000000000000000000, 1.000000000000000000 ) ) ;
#19981=DIRECTION ( 'NONE',  ( -0.000000000000000000, -0.000000000000000000, -1.000000000000000000 ) ) ;
#19986=CARTESIAN_POINT ( 'NONE',  ( -165.0000000000000284, 16.00000000000000000, -84.99999999999998579 ) ) ;
#19993=AXIS2_PLACEMENT_3D ( 'NONE', #34032, #49370, #25821 ) ;
#20008=LINE ( 'NONE', #43856, #50438 ) ;
#20014=VECTOR ( 'NONE', #24093, 1000.000000000000000 ) ;
#20021=LINE ( 'NONE', #35192, #34151 ) ;
#20025=DIRECTION ( 'NONE',  ( -0.000000000000000000, -1.000000000000000000, -0.000000000000000000 ) ) ;
#20028=ADVANCED_FACE ( 'NONE', ( #7859 ), #22474, .F. ) ;
#20030=VECTOR ( 'NONE', #32391, 1000.000000000000000 ) ;
#20038=VECTOR ( 'NONE', #42981, 1000.000000000000000 ) ;
#20040=EDGE_CURVE ( 'NONE', #9900, #27596, #46295, .T. ) ;
#20047=VERTEX_POINT ( 'NONE', #7335 ) ;
#20065=DIRECTION ( 'NONE',  ( -0.000000000000000000, -1.000000000000000000, -0.000000000000000000 ) ) ;
#20073=ORIENTED_EDGE ( 'NONE', *, *, #16218, .T. ) ;
#20075=CARTESIAN_POINT ( 'NONE',  ( 84.99999999999997158, 17.00000000000000000, -90.00000000000000000 ) ) ;
#20087=ORIENTED_EDGE ( 'NONE', *, *, #33668, .T. ) ;
#20099=ORIENTED_EDGE ( 'NONE', *, *, #46152, .F. ) ;
#20102=LINE ( 'NONE', #20354, #36808 ) ;
#20108=VERTEX_POINT ( 'NONE', #40419 ) ;
#20110=CARTESIAN_POINT ( 'NONE',  ( -64.99999999999940314, 17.00000000000000000, -54.99999999999999289 ) ) ;
#20132=ORIENTED_EDGE ( 'NONE', *, *, #193, .F. ) ;
#20147=LINE ( 'NONE', #42719, #2503 ) ;
#20148=ORIENTED_EDGE ( 'NONE', *, *, #32213, .F. ) ;
#20153=EDGE_LOOP ( 'NONE', ( #26197, #22486, #902, #17165 ) ) ;
#20158=VECTOR ( 'NONE', #38518, 1000.000000000000000 ) ;
#20162=DIRECTION ( 'NONE',  ( -0.000000000000000000, -1.000000000000000000, -0.000000000000000000 ) ) ;
#20165=EDGE_CURVE ( 'NONE', #1474, #14334, #23751, .T. ) ;
#20166=CARTESIAN_POINT ( 'NONE',  ( -19.99999999999878142, 17.00000000000000000, 30.00000000000000000 ) ) ;
#20168=LINE ( 'NONE', #16834, #44915 ) ;
#20186=FACE_OUTER_BOUND ( 'NONE', #16917, .T. ) ;
#20192=EDGE_CURVE ( 'NONE', #23599, #3803, #48055, .T. ) ;
#20201=LINE ( 'NONE', #48108, #21321 ) ;
#20202=FACE_OUTER_BOUND ( 'NONE', #3279, .T. ) ;
#20215=ORIENTED_EDGE ( 'NONE', *, *, #2047, .F. ) ;
#20225=FACE_OUTER_BOUND ( 'NONE', #29854, .T. ) ;
#20226=EDGE_CURVE ( 'NONE', #38090, #42902, #18055, .T. ) ;
#20227=DIRECTION ( 'NONE',  ( -1.000000000000000000, 0.000000000000000000, 3.469446951953611724E-16 ) ) ;
#20229=EDGE_CURVE ( 'NONE', #50192, #29738, #13945, .T. ) ;
#20235=DIRECTION ( 'NONE',  ( 0.000000000000000000, -0.000000000000000000, -1.000000000000000000 ) ) ;
#20243=DIRECTION ( 'NONE',  ( 0.000000000000000000, 0.000000000000000000, 1.000000000000000000 ) ) ;
#20249=DIRECTION ( 'NONE',  ( 0.000000000000000000, 0.000000000000000000, 1.000000000000000000 ) ) ;
#20251=ORIENTED_EDGE ( 'NONE', *, *, #19090, .T. ) ;
#20252=PLANE ( 'NONE',  #16464 ) ;
#20265=DIRECTION ( 'NONE',  ( 0.000000000000000000, 0.000000000000000000, -1.000000000000000000 ) ) ;
#20267=ADVANCED_FACE ( 'NONE', ( #2172 ), #6510, .F. ) ;
#20271=VERTEX_POINT ( 'NONE', #45482 ) ;
#20275=AXIS2_PLACEMENT_3D ( 'NONE', #24861, #44571, #44087 ) ;
#20277=CARTESIAN_POINT ( 'NONE',  ( -64.99999999999783995, 16.00000000000000000, 115.0000000000000142 ) ) ;
#20285=EDGE_CURVE ( 'NONE', #20108, #23722, #9360, .T. ) ;
#20287=LINE ( 'NONE', #47192, #10560 ) ;
#20305=DIRECTION ( 'NONE',  ( -0.000000000000000000, -1.000000000000000000, -0.000000000000000000 ) ) ;
#20313=ORIENTED_EDGE ( 'NONE', *, *, #1844, .F. ) ;
#20317=EDGE_CURVE ( 'NONE', #46590, #2507, #19324, .T. ) ;
#20330=EDGE_CURVE ( 'NONE', #31946, #18303, #33975, .T. ) ;
#20331=ORIENTED_EDGE ( 'NONE', *, *, #29114, .T. ) ;
#20336=CARTESIAN_POINT ( 'NONE',  ( 35.00000000000216716, 17.00000000000000000, 115.0000000000000142 ) ) ;
#20354=CARTESIAN_POINT ( 'NONE',  ( 35.00000000000122213, 16.00000000000000000, 30.00000000000000000 ) ) ;
#20355=DIRECTION ( 'NONE',  ( 0.000000000000000000, 0.000000000000000000, 1.000000000000000000 ) ) ;
#20364=DIRECTION ( 'NONE',  ( -0.000000000000000000, -0.000000000000000000, -1.000000000000000000 ) ) ;
#20369=CARTESIAN_POINT ( 'NONE',  ( 135.0000000000009663, 17.00000000000000000, -24.99999999999999289 ) ) ;
#20370=VERTEX_POINT ( 'NONE', #30897 ) ;
#20382=ORIENTED_EDGE ( 'NONE', *, *, #45087, .F. ) ;
#20383=ORIENTED_EDGE ( 'NONE', *, *, #22870, .T. ) ;
#20385=LINE ( 'NONE', #8849, #18403 ) ;
#20386=CARTESIAN_POINT ( 'NONE',  ( -64.99999999999846523, 16.00000000000000000, 60.00000000000000000 ) ) ;
#20388=VERTEX_POINT ( 'NONE', #7026 ) ;
#20389=ORIENTED_EDGE ( 'NONE', *, *, #25839, .F. ) ;
#20390=EDGE_CURVE ( 'NONE', #7259, #38550, #45730, .T. ) ;
#20391=EDGE_LOOP ( 'NONE', ( #7093, #37236, #25028, #36470 ) ) ;
#20399=ORIENTED_EDGE ( 'NONE', *, *, #26633, .F. ) ;
#20404=ORIENTED_EDGE ( 'NONE', *, *, #15233, .F. ) ;
#20407=CARTESIAN_POINT ( 'NONE',  ( -14.99999999999782041, 16.00000000000000000, 95.00000000000000000 ) ) ;
#20411=VECTOR ( 'NONE', #9066, 1000.000000000000000 ) ;
#20418=LINE ( 'NONE', #16330, #27965 ) ;
#20421=DIRECTION ( 'NONE',  ( -0.000000000000000000, -1.000000000000000000, -0.000000000000000000 ) ) ;
#20444=VECTOR ( 'NONE', #28983, 1000.000000000000000 ) ;
#20446=ORIENTED_EDGE ( 'NONE', *, *, #39456, .T. ) ;
#20449=CARTESIAN_POINT ( 'NONE',  ( -14.99999999999970868, 17.00000000000000000, -60.00000000000000000 ) ) ;
#20453=DIRECTION ( 'NONE',  ( -1.000000000000000000, -0.000000000000000000, -0.000000000000000000 ) ) ;
#20474=DIRECTION ( 'NONE',  ( -1.000000000000000000, 0.000000000000000000, -0.000000000000000000 ) ) ;
#20476=PLANE ( 'NONE',  #37548 ) ;
#20488=AXIS2_PLACEMENT_3D ( 'NONE', #27420, #23827, #43052 ) ;
#20489=LINE ( 'NONE', #43831, #14659 ) ;
#20490=CARTESIAN_POINT ( 'NONE',  ( -114.9999999999978542, 17.00000000000000000, 115.0000000000000142 ) ) ;
#20496=ORIENTED_EDGE ( 'NONE', *, *, #28660, .F. ) ;
#20498=FACE_OUTER_BOUND ( 'NONE', #20765, .T. ) ;
#20500=VERTEX_POINT ( 'NONE', #39106 ) ;
#20505=EDGE_CURVE ( 'NONE', #25941, #24997, #39601, .T. ) ;
#20514=ADVANCED_FACE ( 'NONE', ( #12887 ), #31400, .F. ) ;
#20529=CARTESIAN_POINT ( 'NONE',  ( -115.0000000000000284, 17.00000000000000000, -114.9999999999999858 ) ) ;
#20530=VECTOR ( 'NONE', #17719, 1000.000000000000000 ) ;
#20538=CARTESIAN_POINT ( 'NONE',  ( 135.0000000000019043, 17.00000000000000000, 65.00000000000000000 ) ) ;
#20539=DIRECTION ( 'NONE',  ( -0.000000000000000000, -0.000000000000000000, -1.000000000000000000 ) ) ;
#20542=EDGE_CURVE ( 'NONE', #24694, #11870, #43186, .T. ) ;
#20551=CARTESIAN_POINT ( 'NONE',  ( -69.99999999999972999, 17.00000000000000000, -60.00000000000000000 ) ) ;
#20557=CARTESIAN_POINT ( 'NONE',  ( 135.0000000000012790, 17.00000000000000000, 30.00000000000000000 ) ) ;
#20560=AXIS2_PLACEMENT_3D ( 'NONE', #12612, #46719, #31888 ) ;
#20578=VERTEX_POINT ( 'NONE', #13881 ) ;
#20596=CARTESIAN_POINT ( 'NONE',  ( -19.99999999999784706, 17.00000000000000000, 115.0000000000000142 ) ) ;
#20597=AXIS2_PLACEMENT_3D ( 'NONE', #5583, #14033, #45574 ) ;
#20602=VERTEX_POINT ( 'NONE', #21091 ) ;
#20603=DIRECTION ( 'NONE',  ( 1.000000000000000000, 0.000000000000000000, 0.000000000000000000 ) ) ;
#20614=ORIENTED_EDGE ( 'NONE', *, *, #14042, .T. ) ;
#20617=DIRECTION ( 'NONE',  ( 0.000000000000000000, 0.000000000000000000, 1.000000000000000000 ) ) ;
#20619=ADVANCED_FACE ( 'NONE', ( #13141 ), #2348, .F. ) ;
#20642=VERTEX_POINT ( 'NONE', #13646 ) ;
#20653=FACE_OUTER_BOUND ( 'NONE', #35371, .T. ) ;
#20657=VECTOR ( 'NONE', #21538, 1000.000000000000000 ) ;
#20661=VECTOR ( 'NONE', #20364, 1000.000000000000000 ) ;
#20664=ORIENTED_EDGE ( 'NONE', *, *, #5993, .F. ) ;
#20666=CARTESIAN_POINT ( 'NONE',  ( -114.9999999999997158, 16.00000000000000000, -84.99999999999998579 ) ) ;
#20669=EDGE_CURVE ( 'NONE', #30589, #17110, #26213, .T. ) ;
#20680=ADVANCED_FACE ( 'NONE', ( #3099 ), #11060, .F. ) ;
#20688=CARTESIAN_POINT ( 'NONE',  ( 0.000000000000000000, 17.00000000000000000, 0.000000000000000000 ) ) ;
#20690=EDGE_LOOP ( 'NONE', ( #17466, #34250, #15582, #49927 ) ) ;
#20704=DIRECTION ( 'NONE',  ( 0.000000000000000000, 0.000000000000000000, 1.000000000000000000 ) ) ;
#20708=ORIENTED_EDGE ( 'NONE', *, *, #1694, .T. ) ;
#20717=ORIENTED_EDGE ( 'NONE', *, *, #17539, .T. ) ;
#20731=FACE_OUTER_BOUND ( 'NONE', #2580, .T. ) ;
#20733=CARTESIAN_POINT ( 'NONE',  ( 129.9999999999999432, 17.00000000000000000, -114.9999999999999858 ) ) ;
#20736=AXIS2_PLACEMENT_3D ( 'NONE', #28509, #15687, #1057 ) ;
#20737=CARTESIAN_POINT ( 'NONE',  ( 164.9999999999999716, 17.00000000000000000, -55.00000000000000711 ) ) ;
#20738=ORIENTED_EDGE ( 'NONE', *, *, #35913, .F. ) ;
#20761=CARTESIAN_POINT ( 'NONE',  ( 35.00000000000152767, 17.00000000000000000, 35.00000000000000000 ) ) ;
#20765=EDGE_LOOP ( 'NONE', ( #45713, #12016, #9478, #15163 ) ) ;
#20772=EDGE_LOOP ( 'NONE', ( #4821, #31533, #22403, #14271 ) ) ;
#20775=LINE ( 'NONE', #9232, #19290 ) ;
#20784=CARTESIAN_POINT ( 'NONE',  ( -164.9999999999984936, 17.00000000000000000, 35.00000000000000000 ) ) ;
#20786=ORIENTED_EDGE ( 'NONE', *, *, #1844, .T. ) ;
#20806=EDGE_LOOP ( 'NONE', ( #7205, #4882, #4685, #42828 ) ) ;
#20808=ORIENTED_EDGE ( 'NONE', *, *, #32856, .T. ) ;
#20811=EDGE_CURVE ( 'NONE', #1663, #25007, #31339, .T. ) ;
#20812=DIRECTION ( 'NONE',  ( -0.000000000000000000, -1.000000000000000000, -0.000000000000000000 ) ) ;
#20831=LINE ( 'NONE', #1348, #23323 ) ;
#20832=DIRECTION ( 'NONE',  ( -0.000000000000000000, -1.000000000000000000, -0.000000000000000000 ) ) ;
#20839=EDGE_CURVE ( 'NONE', #43085, #17801, #12571, .T. ) ;
#20850=CARTESIAN_POINT ( 'NONE',  ( -165.0000000000000284, 16.00000000000000000, 90.00000000000000000 ) ) ;
#20854=DIRECTION ( 'NONE',  ( -0.000000000000000000, -0.000000000000000000, -1.000000000000000000 ) ) ;
#20855=ORIENTED_EDGE ( 'NONE', *, *, #50220, .F. ) ;
#20857=DIRECTION ( 'NONE',  ( -0.000000000000000000, -0.000000000000000000, -1.000000000000000000 ) ) ;
#20873=ORIENTED_EDGE ( 'NONE', *, *, #2849, .T. ) ;
#20874=VECTOR ( 'NONE', #40663, 1000.000000000000000 ) ;
#20878=DIRECTION ( 'NONE',  ( -0.000000000000000000, -0.000000000000000000, -1.000000000000000000 ) ) ;
#20880=EDGE_LOOP ( 'NONE', ( #6368, #35779, #47023, #23583 ) ) ;
#20881=ORIENTED_EDGE ( 'NONE', *, *, #3463, .T. ) ;
#20883=PLANE ( 'NONE',  #9101 ) ;
#20888=EDGE_LOOP ( 'NONE', ( #13858, #35015, #11582, #21326 ) ) ;
#20889=PLANE ( 'NONE',  #4590 ) ;
#20901=VERTEX_POINT ( 'NONE', #46930 ) ;
#20905=DIRECTION ( 'NONE',  ( -0.000000000000000000, -1.000000000000000000, -0.000000000000000000 ) ) ;
#20911=ORIENTED_EDGE ( 'NONE', *, *, #6149, .F. ) ;
#20919=CARTESIAN_POINT ( 'NONE',  ( -64.99999999999783995, 17.00000000000000000, 95.00000000000000000 ) ) ;
#20928=ORIENTED_EDGE ( 'NONE', *, *, #5268, .T. ) ;
#20932=CARTESIAN_POINT ( 'NONE',  ( -165.0000000000000284, 16.00000000000000000, -30.00000000000000000 ) ) ;
#20941=LINE ( 'NONE', #5025, #49197 ) ;
#20946=VECTOR ( 'NONE', #28984, 1000.000000000000000 ) ;
#20951=VERTEX_POINT ( 'NONE', #49386 ) ;
#20958=ADVANCED_FACE ( 'NONE', ( #6336 ), #26081, .F. ) ;
#20972=DIRECTION ( 'NONE',  ( 1.000000000000000000, 0.000000000000000000, 0.000000000000000000 ) ) ;
#20983=LINE ( 'NONE', #17374, #8653 ) ;
#21007=DIRECTION ( 'NONE',  ( 1.000000000000000000, 0.000000000000000000, -0.000000000000000000 ) ) ;
#21013=ORIENTED_EDGE ( 'NONE', *, *, #49926, .T. ) ;
#21016=ORIENTED_EDGE ( 'NONE', *, *, #17201, .T. ) ;
#21021=ORIENTED_EDGE ( 'NONE', *, *, #32344, .F. ) ;
#21022=CARTESIAN_POINT ( 'NONE',  ( -114.9999999999994031, 17.00000000000000000, -54.99999999999999289 ) ) ;
#21036=CARTESIAN_POINT ( 'NONE',  ( 85.00000000000123634, 16.00000000000000000, 30.00000000000000000 ) ) ;
#21043=VECTOR ( 'NONE', #409, 1000.000000000000000 ) ;
#21052=CARTESIAN_POINT ( 'NONE',  ( 84.99999999999997158, 16.00000000000000000, -90.00000000000000000 ) ) ;
#21055=ORIENTED_EDGE ( 'NONE', *, *, #46925, .T. ) ;
#21069=DIRECTION ( 'NONE',  ( -0.000000000000000000, -1.000000000000000000, -0.000000000000000000 ) ) ;
#21089=ORIENTED_EDGE ( 'NONE', *, *, #8935, .T. ) ;
#21090=DIRECTION ( 'NONE',  ( 4.625929269271584521E-16, -0.000000000000000000, 1.000000000000000000 ) ) ;
#21091=CARTESIAN_POINT ( 'NONE',  ( -19.99999999999940670, 16.00000000000000000, -54.99999999999999289 ) ) ;
#21094=ORIENTED_EDGE ( 'NONE', *, *, #46000, .F. ) ;
#21095=ORIENTED_EDGE ( 'NONE', *, *, #46223, .T. ) ;
#21099=DIRECTION ( 'NONE',  ( -1.000000000000000000, 0.000000000000000000, 0.000000000000000000 ) ) ;
#21110=DIRECTION ( 'NONE',  ( 1.000000000000000000, 0.000000000000000000, 0.000000000000000000 ) ) ;
#21121=EDGE_CURVE ( 'NONE', #32184, #35676, #3998, .T. ) ;
#21129=AXIS2_PLACEMENT_3D ( 'NONE', #6292, #29880, #11149 ) ;
#21137=VERTEX_POINT ( 'NONE', #3221 ) ;
#21147=LINE ( 'NONE', #28594, #46211 ) ;
#21154=EDGE_LOOP ( 'NONE', ( #6664, #32116, #3563, #24625 ) ) ;
#21156=DIRECTION ( 'NONE',  ( -0.000000000000000000, -0.000000000000000000, -1.000000000000000000 ) ) ;
#21162=VERTEX_POINT ( 'NONE', #13207 ) ;
#21169=DIRECTION ( 'NONE',  ( -0.000000000000000000, -1.000000000000000000, -0.000000000000000000 ) ) ;
#21181=DIRECTION ( 'NONE',  ( -1.000000000000000000, 0.000000000000000000, 6.938893903907223447E-16 ) ) ;
#21184=DIRECTION ( 'NONE',  ( 0.000000000000000000, 0.000000000000000000, -1.000000000000000000 ) ) ;
#21189=ORIENTED_EDGE ( 'NONE', *, *, #34638, .F. ) ;
#21195=ORIENTED_EDGE ( 'NONE', *, *, #28847, .F. ) ;
#21198=ORIENTED_EDGE ( 'NONE', *, *, #22745, .F. ) ;
#21212=VECTOR ( 'NONE', #30856, 1000.000000000000000 ) ;
#21230=DIRECTION ( 'NONE',  ( -0.000000000000000000, -1.000000000000000000, -0.000000000000000000 ) ) ;
#21233=DIRECTION ( 'NONE',  ( 0.000000000000000000, -1.000000000000000000, 0.000000000000000000 ) ) ;
#21238=EDGE_CURVE ( 'NONE', #14475, #16065, #37846, .T. ) ;
#21243=ADVANCED_FACE ( 'NONE', ( #2663 ), #40917, .F. ) ;
#21249=EDGE_CURVE ( 'NONE', #970, #8813, #41158, .T. ) ;
#21251=LINE ( 'NONE', #36941, #48564 ) ;
#21254=ORIENTED_EDGE ( 'NONE', *, *, #16218, .F. ) ;
#21260=ORIENTED_EDGE ( 'NONE', *, *, #49422, .F. ) ;
#21281=CARTESIAN_POINT ( 'NONE',  ( -64.99999999999909051, 17.00000000000000000, -24.99999999999999289 ) ) ;
#21285=ADVANCED_FACE ( 'NONE', ( #21406 ), #49319, .F. ) ;
#21287=PLANE ( 'NONE',  #32325 ) ;
#21293=LINE ( 'NONE', #32607, #29196 ) ;
#21297=ORIENTED_EDGE ( 'NONE', *, *, #41831, .F. ) ;
#21299=CARTESIAN_POINT ( 'NONE',  ( -14.99999999999845812, 16.00000000000000000, 35.00000000000000000 ) ) ;
#21312=EDGE_LOOP ( 'NONE', ( #38392, #8073, #26626, #17671 ) ) ;
#21321=VECTOR ( 'NONE', #28412, 1000.000000000000000 ) ;
#21326=ORIENTED_EDGE ( 'NONE', *, *, #18051, .T. ) ;
#21330=DIRECTION ( 'NONE',  ( -1.000000000000000000, -0.000000000000000000, -0.000000000000000000 ) ) ;
#21341=ORIENTED_EDGE ( 'NONE', *, *, #20, .T. ) ;
#21349=EDGE_LOOP ( 'NONE', ( #31839, #28534, #30799, #11116 ) ) ;
#21357=CARTESIAN_POINT ( 'NONE',  ( -14.99999999999812594, 17.00000000000000000, 65.00000000000000000 ) ) ;
#21378=VERTEX_POINT ( 'NONE', #30639 ) ;
#21382=CARTESIAN_POINT ( 'NONE',  ( -64.99999999999971578, 16.00000000000000000, -84.99999999999998579 ) ) ;
#21385=ORIENTED_EDGE ( 'NONE', *, *, #12343, .T. ) ;
#21400=VERTEX_POINT ( 'NONE', #3680 ) ;
#21406=FACE_OUTER_BOUND ( 'NONE', #25443, .T. ) ;
#21414=CARTESIAN_POINT ( 'NONE',  ( 130.0000000000012221, 17.00000000000000000, 30.00000000000000000 ) ) ;
#21435=EDGE_CURVE ( 'NONE', #29552, #46590, #7034, .T. ) ;
#21436=CARTESIAN_POINT ( 'NONE',  ( -119.9999999999984652, 17.00000000000000000, 60.00000000000000000 ) ) ;
#21439=CARTESIAN_POINT ( 'NONE',  ( -14.99999999999970868, 16.00000000000000000, -84.99999999999998579 ) ) ;
#21452=VECTOR ( 'NONE', #38980, 1000.000000000000000 ) ;
#21461=CARTESIAN_POINT ( 'NONE',  ( 135.0000000000019043, 17.00000000000000000, 65.00000000000000000 ) ) ;
#21468=DIRECTION ( 'NONE',  ( -0.000000000000000000, -1.000000000000000000, -0.000000000000000000 ) ) ;
#21469=EDGE_CURVE ( 'NONE', #19127, #10318, #23698, .T. ) ;
#21470=ADVANCED_FACE ( 'NONE', ( #47255 ), #4198, .F. ) ;
#21473=CARTESIAN_POINT ( 'NONE',  ( -14.99999999999970868, 17.00000000000000000, -84.99999999999998579 ) ) ;
#21478=FACE_OUTER_BOUND ( 'NONE', #14759, .T. ) ;
#21480=FACE_OUTER_BOUND ( 'NONE', #36933, .T. ) ;
#21483=PLANE ( 'NONE',  #3115 ) ;
#21490=ORIENTED_EDGE ( 'NONE', *, *, #40312, .F. ) ;
#21499=DIRECTION ( 'NONE',  ( 1.000000000000000000, 0.000000000000000000, 0.000000000000000000 ) ) ;
#21502=DIRECTION ( 'NONE',  ( -1.000000000000000000, 0.000000000000000000, -0.000000000000000000 ) ) ;
#21504=DIRECTION ( 'NONE',  ( -0.000000000000000000, -1.000000000000000000, -0.000000000000000000 ) ) ;
#21511=CARTESIAN_POINT ( 'NONE',  ( 135.0000000000021600, 16.00000000000000000, 95.00000000000000000 ) ) ;
#21513=EDGE_CURVE ( 'NONE', #17122, #43110, #16753, .T. ) ;
#21520=DIRECTION ( 'NONE',  ( 0.000000000000000000, 0.000000000000000000, 1.000000000000000000 ) ) ;
#21521=ORIENTED_EDGE ( 'NONE', *, *, #48527, .F. ) ;
#21524=EDGE_LOOP ( 'NONE', ( #22930, #49173, #14758, #27943 ) ) ;
#21526=DIRECTION ( 'NONE',  ( 0.000000000000000000, 0.000000000000000000, -1.000000000000000000 ) ) ;
#21527=DIRECTION ( 'NONE',  ( -1.000000000000000000, -0.000000000000000000, -0.000000000000000000 ) ) ;
#21529=VERTEX_POINT ( 'NONE', #17508 ) ;
#21533=ORIENTED_EDGE ( 'NONE', *, *, #49351, .F. ) ;
#21534=ADVANCED_FACE ( 'NONE', ( #45426 ), #41363, .F. ) ;
#21535=LINE ( 'NONE', #12834, #28218 ) ;
#21538=DIRECTION ( 'NONE',  ( 1.000000000000000000, 0.000000000000000000, 0.000000000000000000 ) ) ;
#21544=ADVANCED_FACE ( 'NONE', ( #48257 ), #32661, .F. ) ;
#21561=EDGE_LOOP ( 'NONE', ( #20786, #44675, #27536, #47035 ) ) ;
#21566=VECTOR ( 'NONE', #34254, 1000.000000000000000 ) ;
#21573=ORIENTED_EDGE ( 'NONE', *, *, #20505, .F. ) ;
#21574=DIRECTION ( 'NONE',  ( 1.000000000000000000, 0.000000000000000000, -0.000000000000000000 ) ) ;
#21577=CARTESIAN_POINT ( 'NONE',  ( 135.0000000000021600, 17.00000000000000000, 115.0000000000000142 ) ) ;
#21579=ORIENTED_EDGE ( 'NONE', *, *, #23968, .F. ) ;
#21582=EDGE_CURVE ( 'NONE', #22540, #47191, #25207, .T. ) ;
#21591=VERTEX_POINT ( 'NONE', #37537 ) ;
#21592=DIRECTION ( 'NONE',  ( -0.000000000000000000, -0.000000000000000000, -1.000000000000000000 ) ) ;
#21595=LINE ( 'NONE', #16745, #15946 ) ;
#21603=EDGE_CURVE ( 'NONE', #2324, #23722, #50267, .T. ) ;
#21605=VECTOR ( 'NONE', #37489, 1000.000000000000000 ) ;
#21606=DIRECTION ( 'NONE',  ( 0.000000000000000000, 0.000000000000000000, -1.000000000000000000 ) ) ;
#21610=CARTESIAN_POINT ( 'NONE',  ( 164.9999999999999716, 17.00000000000000000, 29.99999999999999289 ) ) ;
#21612=VECTOR ( 'NONE', #28451, 1000.000000000000000 ) ;
#21617=PLANE ( 'NONE',  #19193 ) ;
#21618=DIRECTION ( 'NONE',  ( -0.000000000000000000, -1.000000000000000000, -0.000000000000000000 ) ) ;
#21626=ORIENTED_EDGE ( 'NONE', *, *, #7309, .T. ) ;
#21637=DIRECTION ( 'NONE',  ( 0.000000000000000000, 0.000000000000000000, -1.000000000000000000 ) ) ;
#21638=VECTOR ( 'NONE', #14769, 1000.000000000000000 ) ;
#21648=VERTEX_POINT ( 'NONE', #3106 ) ;
#21680=CARTESIAN_POINT ( 'NONE',  ( 0.000000000000000000, 15.00000000000000000, 0.000000000000000000 ) ) ;
#21683=LINE ( 'NONE', #17836, #8963 ) ;
#21690=VECTOR ( 'NONE', #13549, 1000.000000000000000 ) ;
#21694=LINE ( 'NONE', #29650, #15517 ) ;
#21705=CARTESIAN_POINT ( 'NONE',  ( 85.00000000000184741, 17.00000000000000000, 65.00000000000000000 ) ) ;
#21713=CARTESIAN_POINT ( 'NONE',  ( -69.99999999999783995, 16.00000000000000000, 95.00000000000000000 ) ) ;
#21727=LINE ( 'NONE', #37413, #14120 ) ;
#21733=VECTOR ( 'NONE', #5050, 1000.000000000000000 ) ;
#21739=EDGE_CURVE ( 'NONE', #34745, #1405, #8997, .T. ) ;
#21743=VECTOR ( 'NONE', #18516, 1000.000000000000000 ) ;
#21757=ADVANCED_FACE ( 'NONE', ( #40054 ), #8243, .F. ) ;
#21758=LINE ( 'NONE', #48904, #4080 ) ;
#21762=CARTESIAN_POINT ( 'NONE',  ( 135.0000000000003411, 17.00000000000000000, -84.99999999999998579 ) ) ;
#21765=ORIENTED_EDGE ( 'NONE', *, *, #5797, .F. ) ;
#21766=LINE ( 'NONE', #33578, #43726 ) ;
#21775=CARTESIAN_POINT ( 'NONE',  ( 79.99999999999997158, 16.00000000000000000, -114.9999999999999858 ) ) ;
#21778=EDGE_CURVE ( 'NONE', #37670, #26648, #39804, .T. ) ;
#21779=ORIENTED_EDGE ( 'NONE', *, *, #25874, .T. ) ;
#21780=CARTESIAN_POINT ( 'NONE',  ( -19.99999999999971223, 17.00000000000000000, -60.00000000000000000 ) ) ;
#21781=DIRECTION ( 'NONE',  ( 0.000000000000000000, 0.000000000000000000, 1.000000000000000000 ) ) ;
#21782=DIRECTION ( 'NONE',  ( 0.000000000000000000, 0.000000000000000000, -1.000000000000000000 ) ) ;
#21791=ORIENTED_EDGE ( 'NONE', *, *, #7694, .F. ) ;
#21815=CARTESIAN_POINT ( 'NONE',  ( 30.00000000000217781, 16.00000000000000000, 95.00000000000000000 ) ) ;
#21822=DIRECTION ( 'NONE',  ( 0.000000000000000000, 0.000000000000000000, 1.000000000000000000 ) ) ;
#21825=VECTOR ( 'NONE', #33170, 1000.000000000000000 ) ;
#21831=DIRECTION ( 'NONE',  ( -0.000000000000000000, -1.000000000000000000, -0.000000000000000000 ) ) ;
#21834=EDGE_CURVE ( 'NONE', #36968, #5585, #45118, .T. ) ;
#21835=CARTESIAN_POINT ( 'NONE',  ( 164.9999999999999716, 17.00000000000000000, -90.00000000000002842 ) ) ;
#21836=CARTESIAN_POINT ( 'NONE',  ( -14.99999999999906919, 17.00000000000000000, -24.99999999999999289 ) ) ;
#21843=EDGE_CURVE ( 'NONE', #46680, #14316, #21293, .T. ) ;
#21850=CARTESIAN_POINT ( 'NONE',  ( -119.9999999999978400, 17.00000000000000000, 95.00000000000000000 ) ) ;
#21853=LINE ( 'NONE', #9776, #16938 ) ;
#21859=VECTOR ( 'NONE', #18062, 1000.000000000000000 ) ;
#21869=ORIENTED_EDGE ( 'NONE', *, *, #29694, .T. ) ;
#21870=ORIENTED_EDGE ( 'NONE', *, *, #21778, .F. ) ;
#21872=EDGE_CURVE ( 'NONE', #7557, #17122, #44864, .T. ) ;
#21875=ORIENTED_EDGE ( 'NONE', *, *, #46826, .F. ) ;
#21880=DIRECTION ( 'NONE',  ( -1.000000000000000000, -0.000000000000000000, -0.000000000000000000 ) ) ;
#21887=DIRECTION ( 'NONE',  ( 0.000000000000000000, -0.000000000000000000, -1.000000000000000000 ) ) ;
#21892=VECTOR ( 'NONE', #21230, 1000.000000000000000 ) ;
#21896=PLANE ( 'NONE',  #45064 ) ;
#21899=LINE ( 'NONE', #14687, #8343 ) ;
#21909=ORIENTED_EDGE ( 'NONE', *, *, #6454, .T. ) ;
#21911=CARTESIAN_POINT ( 'NONE',  ( -64.99999999999815259, 17.00000000000000000, 65.00000000000000000 ) ) ;
#21916=FACE_OUTER_BOUND ( 'NONE', #18158, .T. ) ;
#21918=CARTESIAN_POINT ( 'NONE',  ( -114.9999999999984652, 17.00000000000000000, 35.00000000000000000 ) ) ;
#21921=LINE ( 'NONE', #41414, #10141 ) ;
#21937=LINE ( 'NONE', #37604, #25770 ) ;
#21942=PLANE ( 'NONE',  #41334 ) ;
#21953=LINE ( 'NONE', #46271, #13883 ) ;
#21954=EDGE_CURVE ( 'NONE', #2747, #343, #41800, .T. ) ;
#21979=DIRECTION ( 'NONE',  ( 1.000000000000000000, 0.000000000000000000, 0.000000000000000000 ) ) ;
#21981=DIRECTION ( 'NONE',  ( 1.000000000000000000, 0.000000000000000000, 0.000000000000000000 ) ) ;
#21982=VERTEX_POINT ( 'NONE', #50202 ) ;
#21992=DIRECTION ( 'NONE',  ( 0.000000000000000000, 0.000000000000000000, 1.000000000000000000 ) ) ;
#21993=CARTESIAN_POINT ( 'NONE',  ( -15.00000000000001421, 16.00000000000000000, -114.9999999999999858 ) ) ;
#22005=CARTESIAN_POINT ( 'NONE',  ( -64.99999999999940314, 17.00000000000000000, -30.00000000000000000 ) ) ;
#22014=AXIS2_PLACEMENT_3D ( 'NONE', #14614, #19212, #2807 ) ;
#22027=LINE ( 'NONE', #49689, #30807 ) ;
#22050=ORIENTED_EDGE ( 'NONE', *, *, #46571, .T. ) ;
#22062=CARTESIAN_POINT ( 'NONE',  ( 164.9999999999999716, 16.00000000000000000, -84.99999999999998579 ) ) ;
#22064=ADVANCED_FACE ( 'NONE', ( #12034 ), #39745, .F. ) ;
#22081=DIRECTION ( 'NONE',  ( -1.000000000000000000, -0.000000000000000000, -0.000000000000000000 ) ) ;
#22082=VERTEX_POINT ( 'NONE', #732 ) ;
#22083=CARTESIAN_POINT ( 'NONE',  ( -114.9999999999978542, 17.00000000000000000, 95.00000000000000000 ) ) ;
#22084=LINE ( 'NONE', #45656, #23245 ) ;
#22086=DIRECTION ( 'NONE',  ( -0.000000000000000000, -1.000000000000000000, -0.000000000000000000 ) ) ;
#22093=AXIS2_PLACEMENT_3D ( 'NONE', #7567, #23203, #19857 ) ;
#22095=CARTESIAN_POINT ( 'NONE',  ( 35.00000000000061107, 17.00000000000000000, -54.99999999999999289 ) ) ;
#22099=VECTOR ( 'NONE', #13137, 1000.000000000000000 ) ;
#22112=ORIENTED_EDGE ( 'NONE', *, *, #19728, .F. ) ;
#22118=PLANE ( 'NONE',  #24231 ) ;
#22122=CARTESIAN_POINT ( 'NONE',  ( -64.99999999999877787, 16.00000000000000000, 30.00000000000000000 ) ) ;
#22127=VERTEX_POINT ( 'NONE', #8934 ) ;
#22138=ADVANCED_FACE ( 'NONE', ( #40746 ), #48636, .F. ) ;
#22162=EDGE_CURVE ( 'NONE', #38611, #19150, #40990, .T. ) ;
#22167=VECTOR ( 'NONE', #33333, 1000.000000000000000 ) ;
#22173=ORIENTED_EDGE ( 'NONE', *, *, #39613, .T. ) ;
#22180=AXIS2_PLACEMENT_3D ( 'NONE', #34388, #14368, #11026 ) ;
#22182=ADVANCED_FACE ( 'NONE', ( #6593 ), #6852, .F. ) ;
#22188=DIRECTION ( 'NONE',  ( 0.000000000000000000, 0.000000000000000000, 1.000000000000000000 ) ) ;
#22190=CARTESIAN_POINT ( 'NONE',  ( 35.00000000000091660, 17.00000000000000000, -24.99999999999999289 ) ) ;
#22195=EDGE_CURVE ( 'NONE', #29367, #24694, #46320, .T. ) ;
#22197=PLANE ( 'NONE',  #48999 ) ;
#22201=CARTESIAN_POINT ( 'NONE',  ( -165.0000000000000284, 17.00000000000000000, 115.0000000000000142 ) ) ;
#22203=DIRECTION ( 'NONE',  ( 1.000000000000000000, 0.000000000000000000, 0.000000000000000000 ) ) ;
#22220=ORIENTED_EDGE ( 'NONE', *, *, #26579, .T. ) ;
#22231=DIRECTION ( 'NONE',  ( -0.000000000000000000, -1.000000000000000000, -0.000000000000000000 ) ) ;
#22234=CARTESIAN_POINT ( 'NONE',  ( 85.00000000000152056, 17.00000000000000000, 60.00000000000000000 ) ) ;
#22250=CARTESIAN_POINT ( 'NONE',  ( -69.99999999999909051, 17.00000000000000000, -24.99999999999999289 ) ) ;
#22273=ORIENTED_EDGE ( 'NONE', *, *, #15009, .F. ) ;
#22274=ADVANCED_FACE ( 'NONE', ( #28819 ), #12160, .F. ) ;
#22283=EDGE_LOOP ( 'NONE', ( #1344, #3806, #6157, #49934 ) ) ;
#22292=CARTESIAN_POINT ( 'NONE',  ( -64.99999999999909051, 17.00000000000000000, -24.99999999999999289 ) ) ;
#22293=LINE ( 'NONE', #6901, #43060 ) ;
#22294=VERTEX_POINT ( 'NONE', #4717 ) ;
#22297=FACE_BOUND ( 'NONE', #38913, .T. ) ;
#22300=CARTESIAN_POINT ( 'NONE',  ( -15.00000000000001421, 17.00000000000000000, -114.9999999999999858 ) ) ;
#22302=ADVANCED_FACE ( 'NONE', ( #9070 ), #39883, .F. ) ;
#22303=CARTESIAN_POINT ( 'NONE',  ( 30.00000000000153833, 17.00000000000000000, 35.00000000000000000 ) ) ;
#22316=ORIENTED_EDGE ( 'NONE', *, *, #45625, .T. ) ;
#22318=ORIENTED_EDGE ( 'NONE', *, *, #3846, .T. ) ;
#22323=PLANE ( 'NONE',  #10658 ) ;
#22328=FACE_OUTER_BOUND ( 'NONE', #2707, .T. ) ;
#22329=ORIENTED_EDGE ( 'NONE', *, *, #34146, .T. ) ;
#22335=LINE ( 'NONE', #15150, #3613 ) ;
#22337=ORIENTED_EDGE ( 'NONE', *, *, #36641, .F. ) ;
#22357=EDGE_CURVE ( 'NONE', #37670, #34164, #35794, .T. ) ;
#22370=CARTESIAN_POINT ( 'NONE',  ( 35.00000000000091660, 16.00000000000000000, -24.99999999999999289 ) ) ;
#22375=LINE ( 'NONE', #38311, #33532 ) ;
#22384=DIRECTION ( 'NONE',  ( 0.000000000000000000, 0.000000000000000000, 1.000000000000000000 ) ) ;
#22391=CARTESIAN_POINT ( 'NONE',  ( -164.9999999999990905, 17.00000000000000000, 0.000000000000000000 ) ) ;
#22395=ADVANCED_FACE ( 'NONE', ( #14425 ), #1876, .F. ) ;
#22398=ORIENTED_EDGE ( 'NONE', *, *, #16460, .T. ) ;
#22399=ORIENTED_EDGE ( 'NONE', *, *, #15184, .T. ) ;
#22403=ORIENTED_EDGE ( 'NONE', *, *, #46187, .F. ) ;
#22408=FACE_OUTER_BOUND ( 'NONE', #50069, .T. ) ;
#22418=EDGE_LOOP ( 'NONE', ( #20873, #13066, #37302, #40080 ) ) ;
#22423=DIRECTION ( 'NONE',  ( 1.000000000000000000, 0.000000000000000000, 0.000000000000000000 ) ) ;
#22424=ORIENTED_EDGE ( 'NONE', *, *, #17702, .F. ) ;
#22435=DIRECTION ( 'NONE',  ( 0.000000000000000000, -0.000000000000000000, -1.000000000000000000 ) ) ;
#22437=DIRECTION ( 'NONE',  ( 0.000000000000000000, -0.000000000000000000, -1.000000000000000000 ) ) ;
#22445=VECTOR ( 'NONE', #40752, 1000.000000000000000 ) ;
#22466=ORIENTED_EDGE ( 'NONE', *, *, #4921, .F. ) ;
#22474=PLANE ( 'NONE',  #475 ) ;
#22483=DIRECTION ( 'NONE',  ( -1.000000000000000000, -0.000000000000000000, -0.000000000000000000 ) ) ;
#22486=ORIENTED_EDGE ( 'NONE', *, *, #43264, .F. ) ;
#22487=ORIENTED_EDGE ( 'NONE', *, *, #17354, .F. ) ;
#22494=LINE ( 'NONE', #45306, #8569 ) ;
#22496=DIRECTION ( 'NONE',  ( 0.000000000000000000, -1.000000000000000000, 0.000000000000000000 ) ) ;
#22506=EDGE_CURVE ( 'NONE', #41895, #41913, #50277, .T. ) ;
#22509=VECTOR ( 'NONE', #48869, 1000.000000000000000 ) ;
#22516=ORIENTED_EDGE ( 'NONE', *, *, #20317, .F. ) ;
#22520=ADVANCED_FACE ( 'NONE', ( #30849 ), #15685, .F. ) ;
#22528=DIRECTION ( 'NONE',  ( 0.000000000000000000, -0.000000000000000000, -1.000000000000000000 ) ) ;
#22529=VERTEX_POINT ( 'NONE', #42619 ) ;
#22533=CARTESIAN_POINT ( 'NONE',  ( 130.0000000000021032, 16.00000000000000000, 115.0000000000000142 ) ) ;
#22537=DIRECTION ( 'NONE',  ( -1.000000000000000000, 0.000000000000000000, 0.000000000000000000 ) ) ;
#22538=EDGE_LOOP ( 'NONE', ( #45905, #30235, #35615, #9509 ) ) ;
#22540=VERTEX_POINT ( 'NONE', #3116 ) ;
#22541=VERTEX_POINT ( 'NONE', #11078 ) ;
#22546=FACE_BOUND ( 'NONE', #8846, .T. ) ;
#22549=AXIS2_PLACEMENT_3D ( 'NONE', #47264, #11907, #47521 ) ;
#22562=ORIENTED_EDGE ( 'NONE', *, *, #24874, .F. ) ;
#22577=DIRECTION ( 'NONE',  ( 0.000000000000000000, 0.000000000000000000, -1.000000000000000000 ) ) ;
#22585=CARTESIAN_POINT ( 'NONE',  ( -19.99999999999783995, 16.00000000000000000, 95.00000000000000000 ) ) ;
#22591=CARTESIAN_POINT ( 'NONE',  ( -19.99999999999908695, 17.00000000000000000, 0.000000000000000000 ) ) ;
#22601=LINE ( 'NONE', #42590, #12491 ) ;
#22607=LINE ( 'NONE', #42354, #44765 ) ;
#22608=ORIENTED_EDGE ( 'NONE', *, *, #34641, .F. ) ;
#22611=DIRECTION ( 'NONE',  ( -1.000000000000000000, 0.000000000000000000, 0.000000000000000000 ) ) ;
#22614=ORIENTED_EDGE ( 'NONE', *, *, #25235, .F. ) ;
#22620=ADVANCED_FACE ( 'NONE', ( #16453 ), #4146, .F. ) ;
#22630=CARTESIAN_POINT ( 'NONE',  ( -64.99999999999846523, 17.00000000000000000, 35.00000000000000000 ) ) ;
#22638=ORIENTED_EDGE ( 'NONE', *, *, #740, .T. ) ;
#22640=DIRECTION ( 'NONE',  ( -0.000000000000000000, -1.000000000000000000, -0.000000000000000000 ) ) ;
#22641=CARTESIAN_POINT ( 'NONE',  ( 30.00000000000092726, 17.00000000000000000, -24.99999999999999289 ) ) ;
#22642=ORIENTED_EDGE ( 'NONE', *, *, #21513, .F. ) ;
#22644=PLANE ( 'NONE',  #32000 ) ;
#22657=CARTESIAN_POINT ( 'NONE',  ( 35.00000000000186162, 17.00000000000000000, 90.00000000000000000 ) ) ;
#22661=CARTESIAN_POINT ( 'NONE',  ( 35.00000000000186162, 17.00000000000000000, 65.00000000000000000 ) ) ;
#22679=EDGE_LOOP ( 'NONE', ( #27355, #3499, #44821, #7134 ) ) ;
#22696=CARTESIAN_POINT ( 'NONE',  ( 85.00000000000184741, 16.00000000000000000, 90.00000000000000000 ) ) ;
#22701=ORIENTED_EDGE ( 'NONE', *, *, #46919, .F. ) ;
#22714=VECTOR ( 'NONE', #21592, 1000.000000000000000 ) ;
#22721=VERTEX_POINT ( 'NONE', #46856 ) ;
#22731=ORIENTED_EDGE ( 'NONE', *, *, #12343, .F. ) ;
#22745=EDGE_CURVE ( 'NONE', #37254, #302, #42530, .T. ) ;
#22747=ORIENTED_EDGE ( 'NONE', *, *, #9317, .T. ) ;
#22757=ORIENTED_EDGE ( 'NONE', *, *, #35761, .T. ) ;
#22763=EDGE_CURVE ( 'NONE', #20370, #47244, #26388, .T. ) ;
#22765=VERTEX_POINT ( 'NONE', #42034 ) ;
#22769=LINE ( 'NONE', #19162, #32369 ) ;
#22771=VERTEX_POINT ( 'NONE', #37701 ) ;
#22780=CARTESIAN_POINT ( 'NONE',  ( 30.00000000000123279, 17.00000000000000000, 30.00000000000000000 ) ) ;
#22786=FACE_OUTER_BOUND ( 'NONE', #47197, .T. ) ;
#22790=PLANE ( 'NONE',  #31724 ) ;
#22792=ORIENTED_EDGE ( 'NONE', *, *, #31926, .T. ) ;
#22800=FACE_OUTER_BOUND ( 'NONE', #12454, .T. ) ;
#22806=DIRECTION ( 'NONE',  ( 1.000000000000000000, 0.000000000000000000, -0.000000000000000000 ) ) ;
#22808=ADVANCED_FACE ( 'NONE', ( #22786 ), #33595, .F. ) ;
#22809=DIRECTION ( 'NONE',  ( 0.000000000000000000, 0.000000000000000000, 1.000000000000000000 ) ) ;
#22811=ADVANCED_FACE ( 'NONE', ( #14327 ), #2277, .F. ) ;
#22813=FACE_OUTER_BOUND ( 'NONE', #47237, .T. ) ;
#22817=ORIENTED_EDGE ( 'NONE', *, *, #23279, .T. ) ;
#22825=VERTEX_POINT ( 'NONE', #22533 ) ;
#22845=ADVANCED_FACE ( 'NONE', ( #13811 ), #38463, .F. ) ;
#22850=ORIENTED_EDGE ( 'NONE', *, *, #2203, .T. ) ;
#22853=VERTEX_POINT ( 'NONE', #38218 ) ;
#22858=EDGE_CURVE ( 'NONE', #28153, #40717, #14073, .T. ) ;
#22870=EDGE_CURVE ( 'NONE', #20500, #2288, #6380, .T. ) ;
#22872=ADVANCED_FACE ( 'NONE', ( #25639 ), #25896, .F. ) ;
#22878=DIRECTION ( 'NONE',  ( 0.000000000000000000, -0.000000000000000000, -1.000000000000000000 ) ) ;
#22880=EDGE_CURVE ( 'NONE', #35976, #1474, #22027, .T. ) ;
#22884=CARTESIAN_POINT ( 'NONE',  ( 130.0000000000012221, 17.00000000000000000, 30.00000000000000000 ) ) ;
#22896=FACE_OUTER_BOUND ( 'NONE', #3914, .T. ) ;
#22904=ORIENTED_EDGE ( 'NONE', *, *, #19976, .F. ) ;
#22909=VECTOR ( 'NONE', #37572, 1000.000000000000000 ) ;
#22916=EDGE_LOOP ( 'NONE', ( #32279, #19426, #40171, #25565 ) ) ;
#22918=VERTEX_POINT ( 'NONE', #3798 ) ;
#22928=ORIENTED_EDGE ( 'NONE', *, *, #4974, .T. ) ;
#22930=ORIENTED_EDGE ( 'NONE', *, *, #33997, .T. ) ;
#22931=DIRECTION ( 'NONE',  ( -1.000000000000000000, 0.000000000000000000, -0.000000000000000000 ) ) ;
#22939=ORIENTED_EDGE ( 'NONE', *, *, #23116, .F. ) ;
#22943=CARTESIAN_POINT ( 'NONE',  ( 0.000000000000000000, 17.00000000000000000, 0.000000000000000000 ) ) ;
#22968=VECTOR ( 'NONE', #15365, 1000.000000000000000 ) ;
#22969=VERTEX_POINT ( 'NONE', #50449 ) ;
#22976=DIRECTION ( 'NONE',  ( 0.000000000000000000, -1.000000000000000000, 0.000000000000000000 ) ) ;
#22986=CARTESIAN_POINT ( 'NONE',  ( -114.9999999999997158, 16.00000000000000000, -60.00000000000000000 ) ) ;
#22992=EDGE_CURVE ( 'NONE', #23347, #27632, #8421, .T. ) ;
#23006=ORIENTED_EDGE ( 'NONE', *, *, #44331, .F. ) ;
#23025=CARTESIAN_POINT ( 'NONE',  ( 35.00000000000122213, 17.00000000000000000, 30.00000000000000000 ) ) ;
#23034=CARTESIAN_POINT ( 'NONE',  ( -114.9999999999997158, 17.00000000000000000, -84.99999999999998579 ) ) ;
#23041=ORIENTED_EDGE ( 'NONE', *, *, #29071, .T. ) ;
#23042=CARTESIAN_POINT ( 'NONE',  ( -20.00000000000001776, 16.00000000000000000, -114.9999999999999858 ) ) ;
#23045=VECTOR ( 'NONE', #8026, 1000.000000000000000 ) ;
#23054=EDGE_CURVE ( 'NONE', #49813, #15078, #17115, .T. ) ;
#23064=VERTEX_POINT ( 'NONE', #709 ) ;
#23068=AXIS2_PLACEMENT_3D ( 'NONE', #44625, #45382, #44876 ) ;
#23073=ORIENTED_EDGE ( 'NONE', *, *, #8929, .F. ) ;
#23076=VECTOR ( 'NONE', #4400, 1000.000000000000000 ) ;
#23083=ORIENTED_EDGE ( 'NONE', *, *, #23108, .F. ) ;
#23089=DIRECTION ( 'NONE',  ( 0.000000000000000000, 0.000000000000000000, 1.000000000000000000 ) ) ;
#23090=LINE ( 'NONE', #18481, #30623 ) ;
#23099=EDGE_CURVE ( 'NONE', #22082, #26763, #8674, .T. ) ;
#23101=ORIENTED_EDGE ( 'NONE', *, *, #6445, .F. ) ;
#23105=ORIENTED_EDGE ( 'NONE', *, *, #20165, .T. ) ;
#23106=DIRECTION ( 'NONE',  ( 1.000000000000000000, 0.000000000000000000, 0.000000000000000000 ) ) ;
#23108=EDGE_CURVE ( 'NONE', #31779, #614, #44289, .T. ) ;
#23116=EDGE_CURVE ( 'NONE', #2839, #10058, #32278, .T. ) ;
#23126=CARTESIAN_POINT ( 'NONE',  ( -14.99999999999845812, 17.00000000000000000, 35.00000000000000000 ) ) ;
#23128=LINE ( 'NONE', #42778, #19230 ) ;
#23129=PLANE ( 'NONE',  #33826 ) ;
#23137=DIRECTION ( 'NONE',  ( -0.000000000000000000, -1.000000000000000000, -0.000000000000000000 ) ) ;
#23138=EDGE_LOOP ( 'NONE', ( #11674, #21189, #41830, #3742 ) ) ;
#23147=CARTESIAN_POINT ( 'NONE',  ( -20.00000000000003197, 17.00000000000000000, -114.9999999999999858 ) ) ;
#23150=DIRECTION ( 'NONE',  ( -1.000000000000000000, 0.000000000000000000, -0.000000000000000000 ) ) ;
#23157=ORIENTED_EDGE ( 'NONE', *, *, #10322, .T. ) ;
#23175=PLANE ( 'NONE',  #18133 ) ;
#23187=CARTESIAN_POINT ( 'NONE',  ( -14.99999999999937472, 17.00000000000000000, -30.00000000000000000 ) ) ;
#23191=VECTOR ( 'NONE', #45512, 1000.000000000000000 ) ;
#23194=ORIENTED_EDGE ( 'NONE', *, *, #5261, .T. ) ;
#23195=CARTESIAN_POINT ( 'NONE',  ( 135.0000000000012790, 17.00000000000000000, 5.000000000000004441 ) ) ;
#23203=DIRECTION ( 'NONE',  ( 0.000000000000000000, 0.000000000000000000, -1.000000000000000000 ) ) ;
#23211=ORIENTED_EDGE ( 'NONE', *, *, #6631, .T. ) ;
#23214=VECTOR ( 'NONE', #20812, 1000.000000000000000 ) ;
#23233=ORIENTED_EDGE ( 'NONE', *, *, #20229, .T. ) ;
#23245=VECTOR ( 'NONE', #34404, 1000.000000000000000 ) ;
#23251=CARTESIAN_POINT ( 'NONE',  ( -69.99999999999879208, 16.00000000000000000, 5.000000000000004441 ) ) ;
#23254=AXIS2_PLACEMENT_3D ( 'NONE', #15625, #31297, #50473 ) ;
#23279=EDGE_CURVE ( 'NONE', #11818, #33150, #45041, .T. ) ;
#23282=ORIENTED_EDGE ( 'NONE', *, *, #44608, .F. ) ;
#23290=EDGE_LOOP ( 'NONE', ( #41779, #42846, #35033, #50109 ) ) ;
#23296=DIRECTION ( 'NONE',  ( -0.000000000000000000, -1.000000000000000000, -0.000000000000000000 ) ) ;
#23303=DIRECTION ( 'NONE',  ( 0.000000000000000000, 0.000000000000000000, -1.000000000000000000 ) ) ;
#23307=AXIS2_PLACEMENT_3D ( 'NONE', #50022, #27498, #34704 ) ;
#23323=VECTOR ( 'NONE', #8542, 1000.000000000000000 ) ;
#23347=VERTEX_POINT ( 'NONE', #46297 ) ;
#23349=CARTESIAN_POINT ( 'NONE',  ( -70.00000000000002842, 16.00000000000000000, -90.00000000000000000 ) ) ;
#23353=ORIENTED_EDGE ( 'NONE', *, *, #48359, .F. ) ;
#23354=DIRECTION ( 'NONE',  ( -1.000000000000000000, -0.000000000000000000, -0.000000000000000000 ) ) ;
#23356=ADVANCED_FACE ( 'NONE', ( #42715 ), #7592, .F. ) ;
#23358=VERTEX_POINT ( 'NONE', #32397 ) ;
#23363=VERTEX_POINT ( 'NONE', #3468 ) ;
#23367=ORIENTED_EDGE ( 'NONE', *, *, #34932, .F. ) ;
#23369=LINE ( 'NONE', #38993, #25725 ) ;
#23374=FACE_OUTER_BOUND ( 'NONE', #24657, .T. ) ;
#23377=VERTEX_POINT ( 'NONE', #7860 ) ;
#23390=LINE ( 'NONE', #23643, #38898 ) ;
#23395=CARTESIAN_POINT ( 'NONE',  ( -69.99999999999909051, 17.00000000000000000, 0.000000000000000000 ) ) ;
#23403=ORIENTED_EDGE ( 'NONE', *, *, #7437, .F. ) ;
#23412=FACE_OUTER_BOUND ( 'NONE', #16784, .T. ) ;
#23414=DIRECTION ( 'NONE',  ( -1.000000000000000000, 0.000000000000000000, 9.251858538542979716E-16 ) ) ;
#23418=CARTESIAN_POINT ( 'NONE',  ( 80.00000000000092371, 17.00000000000000000, 0.000000000000000000 ) ) ;
#23420=CARTESIAN_POINT ( 'NONE',  ( 30.00000000000153833, 17.00000000000000000, 60.00000000000000000 ) ) ;
#23421=ORIENTED_EDGE ( 'NONE', *, *, #40875, .T. ) ;
#23435=VECTOR ( 'NONE', #2961, 1000.000000000000000 ) ;
#23437=PLANE ( 'NONE',  #38300 ) ;
#23440=AXIS2_PLACEMENT_3D ( 'NONE', #33258, #12960, #49091 ) ;
#23441=CARTESIAN_POINT ( 'NONE',  ( -165.0000000000000284, 17.00000000000000000, -114.9999999999999858 ) ) ;
#23443=LINE ( 'NONE', #46736, #38658 ) ;
#23446=ORIENTED_EDGE ( 'NONE', *, *, #41822, .T. ) ;
#23456=CARTESIAN_POINT ( 'NONE',  ( -64.99999999999783995, 17.00000000000000000, 115.0000000000000142 ) ) ;
#23470=EDGE_CURVE ( 'NONE', #36660, #21982, #17249, .T. ) ;
#23471=AXIS2_PLACEMENT_3D ( 'NONE', #2886, #15228, #19561 ) ;
#23473=AXIS2_PLACEMENT_3D ( 'NONE', #36966, #21526, #5372 ) ;
#23474=AXIS2_PLACEMENT_3D ( 'NONE', #11892, #23939, #8553 ) ;
#23491=LINE ( 'NONE', #39147, #47587 ) ;
#23493=VERTEX_POINT ( 'NONE', #48992 ) ;
#23499=VERTEX_POINT ( 'NONE', #50254 ) ;
#23504=EDGE_LOOP ( 'NONE', ( #25677, #48053, #45991, #18913 ) ) ;
#23514=UNCERTAINTY_MEASURE_WITH_UNIT (LENGTH_MEASURE( 1.000000000000000082E-05 ), #13364, 'distance_accuracy_value', 'NONE');
#23515=EDGE_LOOP ( 'NONE', ( #6461, #13676, #21297, #5377, #31649, #20399, #2096, #19681, #37638, #32824, #32966, #39535, #7493, #44987, #21254, #33719, #8148, #49214, #43879, #5442, #25381, #2374, #21195, #18767, #35034, #31831, #50380, #48940, #37143, #8261, #47978, #9457 ) ) ;
#23518=ORIENTED_EDGE ( 'NONE', *, *, #16501, .F. ) ;
#23520=CARTESIAN_POINT ( 'NONE',  ( 84.99999999999997158, 17.00000000000000000, -114.9999999999999858 ) ) ;
#23521=CARTESIAN_POINT ( 'NONE',  ( -14.99999999999812594, 17.00000000000000000, 65.00000000000000000 ) ) ;
#23527=CARTESIAN_POINT ( 'NONE',  ( 30.00000000000062172, 17.00000000000000000, -54.99999999999999289 ) ) ;
#23534=DIRECTION ( 'NONE',  ( -1.000000000000000000, 0.000000000000000000, 0.000000000000000000 ) ) ;
#23536=LINE ( 'NONE', #39446, #42674 ) ;
#23540=FACE_OUTER_BOUND ( 'NONE', #28842, .T. ) ;
#23542=DIRECTION ( 'NONE',  ( 0.000000000000000000, 0.000000000000000000, -1.000000000000000000 ) ) ;
#23563=EDGE_LOOP ( 'NONE', ( #32952, #10301, #32470, #40200 ) ) ;
#23580=CARTESIAN_POINT ( 'NONE',  ( 35.00000000000216716, 17.00000000000000000, 95.00000000000000000 ) ) ;
#23583=ORIENTED_EDGE ( 'NONE', *, *, #40232, .T. ) ;
#23595=LINE ( 'NONE', #7452, #29527 ) ;
#23599=VERTEX_POINT ( 'NONE', #3606 ) ;
#23601=ORIENTED_EDGE ( 'NONE', *, *, #5993, .T. ) ;
#23613=EDGE_CURVE ( 'NONE', #40073, #31274, #33915, .T. ) ;
#23621=LINE ( 'NONE', #32345, #35813 ) ;
#23625=DIRECTION ( 'NONE',  ( 0.000000000000000000, -1.000000000000000000, 0.000000000000000000 ) ) ;
#23633=VERTEX_POINT ( 'NONE', #30068 ) ;
#23643=CARTESIAN_POINT ( 'NONE',  ( -69.99999999999783995, 17.00000000000000000, 95.00000000000000000 ) ) ;
#23647=EDGE_CURVE ( 'NONE', #11684, #26946, #22607, .T. ) ;
#23656=APPLICATION_CONTEXT ( 'automotive_design' ) ;
#23665=CARTESIAN_POINT ( 'NONE',  ( 164.9999999999999716, 17.00000000000000000, -25.00000000000000711 ) ) ;
#23675=EDGE_CURVE ( 'NONE', #49920, #11818, #20021, .T. ) ;
#23677=AXIS2_PLACEMENT_3D ( 'NONE', #15890, #35413, #23847 ) ;
#23681=CARTESIAN_POINT ( 'NONE',  ( -119.9999999999997158, 16.00000000000000000, -60.00000000000000000 ) ) ;
#23682=ORIENTED_EDGE ( 'NONE', *, *, #16153, .T. ) ;
#23689=CARTESIAN_POINT ( 'NONE',  ( 30.00000000000092726, 16.00000000000000000, -24.99999999999999289 ) ) ;
#23691=CARTESIAN_POINT ( 'NONE',  ( 135.0000000000019043, 16.00000000000000000, 65.00000000000000000 ) ) ;
#23695=ORIENTED_EDGE ( 'NONE', *, *, #33045, .T. ) ;
#23698=LINE ( 'NONE', #16250, #31629 ) ;
#23700=VERTEX_POINT ( 'NONE', #4378 ) ;
#23706=CARTESIAN_POINT ( 'NONE',  ( 164.9999999999999716, 15.00000000000000000, 115.0000000000000142 ) ) ;
#23714=ORIENTED_EDGE ( 'NONE', *, *, #3916, .T. ) ;
#23716=DIRECTION ( 'NONE',  ( -0.000000000000000000, -1.000000000000000000, -0.000000000000000000 ) ) ;
#23722=VERTEX_POINT ( 'NONE', #4130 ) ;
#23732=DIRECTION ( 'NONE',  ( -1.000000000000000000, -0.000000000000000000, -0.000000000000000000 ) ) ;
#23735=CARTESIAN_POINT ( 'NONE',  ( 0.000000000000000000, 17.00000000000000000, 0.000000000000000000 ) ) ;
#23747=ORIENTED_EDGE ( 'NONE', *, *, #20839, .T. ) ;
#23749=AXIS2_PLACEMENT_3D ( 'NONE', #40772, #5100, #24377 ) ;
#23751=LINE ( 'NONE', #24509, #37374 ) ;
#23752=VECTOR ( 'NONE', #1268, 1000.000000000000000 ) ;
#23753=EDGE_CURVE ( 'NONE', #35737, #2212, #23621, .T. ) ;
#23758=DIRECTION ( 'NONE',  ( -1.000000000000000000, -0.000000000000000000, -0.000000000000000000 ) ) ;
#23759=ORIENTED_EDGE ( 'NONE', *, *, #38878, .F. ) ;
#23772=PLANE ( 'NONE',  #31896 ) ;
#23775=LINE ( 'NONE', #11461, #40635 ) ;
#23785=VECTOR ( 'NONE', #2941, 1000.000000000000000 ) ;
#23791=LINE ( 'NONE', #43018, #16543 ) ;
#23794=CARTESIAN_POINT ( 'NONE',  ( 79.99999999999997158, 17.00000000000000000, -114.9999999999999858 ) ) ;
#23799=ORIENTED_EDGE ( 'NONE', *, *, #38401, .F. ) ;
#23807=EDGE_CURVE ( 'NONE', #9256, #16065, #40540, .T. ) ;
#23809=ORIENTED_EDGE ( 'NONE', *, *, #18580, .T. ) ;
#23811=EDGE_CURVE ( 'NONE', #19067, #38090, #44362, .T. ) ;
#23815=ORIENTED_EDGE ( 'NONE', *, *, #39589, .T. ) ;
#23817=LINE ( 'NONE', #4317, #12218 ) ;
#23827=DIRECTION ( 'NONE',  ( -1.000000000000000000, 0.000000000000000000, 0.000000000000000000 ) ) ;
#23829=AXIS2_PLACEMENT_3D ( 'NONE', #41254, #21499, #49164 ) ;
#23835=CARTESIAN_POINT ( 'NONE',  ( -14.99999999999782041, 17.00000000000000000, 95.00000000000000000 ) ) ;
#23836=AXIS2_PLACEMENT_3D ( 'NONE', #49758, #7221, #14657 ) ;
#23838=VECTOR ( 'NONE', #15635, 1000.000000000000000 ) ;
#23847=DIRECTION ( 'NONE',  ( -1.000000000000000000, 0.000000000000000000, -0.000000000000000000 ) ) ;
#23848=CARTESIAN_POINT ( 'NONE',  ( 35.00000000000091660, 17.00000000000000000, -24.99999999999999289 ) ) ;
#23850=EDGE_CURVE ( 'NONE', #15777, #22294, #20775, .T. ) ;
#23856=DIRECTION ( 'NONE',  ( 1.000000000000000000, 0.000000000000000000, -0.000000000000000000 ) ) ;
#23857=CARTESIAN_POINT ( 'NONE',  ( -119.9999999999997158, 17.00000000000000000, -60.00000000000000000 ) ) ;
#23868=VECTOR ( 'NONE', #3412, 1000.000000000000000 ) ;
#23870=VECTOR ( 'NONE', #12472, 1000.000000000000000 ) ;
#23877=CARTESIAN_POINT ( 'NONE',  ( 0.000000000000000000, 17.00000000000000000, 0.000000000000000000 ) ) ;
#23886=CARTESIAN_POINT ( 'NONE',  ( 0.000000000000000000, 17.00000000000000000, 0.000000000000000000 ) ) ;
#23887=CARTESIAN_POINT ( 'NONE',  ( 135.0000000000009663, 17.00000000000000000, -24.99999999999999289 ) ) ;
#23890=ORIENTED_EDGE ( 'NONE', *, *, #15994, .F. ) ;
#23904=EDGE_LOOP ( 'NONE', ( #45073, #166, #23890, #49695 ) ) ;
#23905=CARTESIAN_POINT ( 'NONE',  ( 35.00000000000061107, 17.00000000000000000, -30.00000000000000000 ) ) ;
#23917=VERTEX_POINT ( 'NONE', #29491 ) ;
#23939=DIRECTION ( 'NONE',  ( 0.000000000000000000, 0.000000000000000000, 1.000000000000000000 ) ) ;
#23940=EDGE_CURVE ( 'NONE', #42175, #4762, #32857, .T. ) ;
#23947=DIRECTION ( 'NONE',  ( 0.000000000000000000, 0.000000000000000000, -1.000000000000000000 ) ) ;
#23957=CARTESIAN_POINT ( 'NONE',  ( 85.00000000000056843, 17.00000000000000000, -54.99999999999999289 ) ) ;
#23960=CARTESIAN_POINT ( 'NONE',  ( 135.0000000000000000, 17.00000000000000000, -114.9999999999999858 ) ) ;
#23962=VERTEX_POINT ( 'NONE', #45358 ) ;
#23968=EDGE_CURVE ( 'NONE', #37688, #20047, #22293, .T. ) ;
#23978=CARTESIAN_POINT ( 'NONE',  ( -114.9999999999994031, 16.00000000000000000, -54.99999999999999289 ) ) ;
#23985=VECTOR ( 'NONE', #34174, 1000.000000000000000 ) ;
#23993=EDGE_CURVE ( 'NONE', #31669, #20047, #37970, .T. ) ;
#23994=ORIENTED_EDGE ( 'NONE', *, *, #48664, .F. ) ;
#23997=DIRECTION ( 'NONE',  ( 1.000000000000000000, 0.000000000000000000, -0.000000000000000000 ) ) ;
#24009=ORIENTED_EDGE ( 'NONE', *, *, #48063, .T. ) ;
#24012=VERTEX_POINT ( 'NONE', #49196 ) ;
#24017=VERTEX_POINT ( 'NONE', #43562 ) ;
#24027=ADVANCED_FACE ( 'NONE', ( #31022 ), #19189, .F. ) ;
#24033=CARTESIAN_POINT ( 'NONE',  ( 80.00000000000092371, 16.00000000000000000, -24.99999999999999289 ) ) ;
#24049=VECTOR ( 'NONE', #25163, 1000.000000000000000 ) ;
#24054=DIRECTION ( 'NONE',  ( -0.000000000000000000, -1.000000000000000000, -0.000000000000000000 ) ) ;
#24058=ORIENTED_EDGE ( 'NONE', *, *, #43451, .T. ) ;
#24059=VERTEX_POINT ( 'NONE', #43303 ) ;
#24067=DIRECTION ( 'NONE',  ( 0.000000000000000000, 0.000000000000000000, 1.000000000000000000 ) ) ;
#24072=ORIENTED_EDGE ( 'NONE', *, *, #29686, .T. ) ;
#24073=DIRECTION ( 'NONE',  ( 0.000000000000000000, 0.000000000000000000, -1.000000000000000000 ) ) ;
#24080=CARTESIAN_POINT ( 'NONE',  ( -14.99999999999876366, 17.00000000000000000, 5.000000000000004441 ) ) ;
#24090=DIRECTION ( 'NONE',  ( 3.469446951953611724E-16, 0.000000000000000000, 1.000000000000000000 ) ) ;
#24093=DIRECTION ( 'NONE',  ( -0.000000000000000000, -0.000000000000000000, 1.000000000000000000 ) ) ;
#24096=CARTESIAN_POINT ( 'NONE',  ( -64.99999999999877787, 17.00000000000000000, 5.000000000000004441 ) ) ;
#24111=ADVANCED_FACE ( 'NONE', ( #12512 ), #50458, .F. ) ;
#24113=ORIENTED_EDGE ( 'NONE', *, *, #14270, .F. ) ;
#24117=VECTOR ( 'NONE', #43792, 1000.000000000000000 ) ;
#24129=DIRECTION ( 'NONE',  ( 1.000000000000000000, 0.000000000000000000, 0.000000000000000000 ) ) ;
#24135=CARTESIAN_POINT ( 'NONE',  ( -69.99999999999879208, 17.00000000000000000, 5.000000000000004441 ) ) ;
#24138=AXIS2_PLACEMENT_3D ( 'NONE', #17634, #30189, #7359 ) ;
#24143=DIRECTION ( 'NONE',  ( 1.000000000000000000, 0.000000000000000000, 0.000000000000000000 ) ) ;
#24149=FACE_OUTER_BOUND ( 'NONE', #11082, .T. ) ;
#24153=DIRECTION ( 'NONE',  ( 1.000000000000000000, 0.000000000000000000, 0.000000000000000000 ) ) ;
#24162=DIRECTION ( 'NONE',  ( 1.000000000000000000, 0.000000000000000000, -0.000000000000000000 ) ) ;
#24166=CARTESIAN_POINT ( 'NONE',  ( 135.0000000000015632, 17.00000000000000000, 35.00000000000000000 ) ) ;
#24171=VECTOR ( 'NONE', #37859, 1000.000000000000000 ) ;
#24180=CARTESIAN_POINT ( 'NONE',  ( 175.0000000000000000, 0.000000000000000000, 122.5000000000000142 ) ) ;
#24182=VERTEX_POINT ( 'NONE', #13261 ) ;
#24187=VECTOR ( 'NONE', #44456, 1000.000000000000000 ) ;
#24194=AXIS2_PLACEMENT_3D ( 'NONE', #2977, #49139, #45053 ) ;
#24205=ORIENTED_EDGE ( 'NONE', *, *, #9676, .F. ) ;
#24218=CARTESIAN_POINT ( 'NONE',  ( 80.00000000000153477, 17.00000000000000000, 60.00000000000000000 ) ) ;
#24225=ORIENTED_EDGE ( 'NONE', *, *, #5237, .T. ) ;
#24227=DIRECTION ( 'NONE',  ( 1.000000000000000000, 0.000000000000000000, -4.625929269271687073E-16 ) ) ;
#24231=AXIS2_PLACEMENT_3D ( 'NONE', #5705, #1871, #5958 ) ;
#24237=DIRECTION ( 'NONE',  ( 0.000000000000000000, -0.000000000000000000, -1.000000000000000000 ) ) ;
#24245=EDGE_CURVE ( 'NONE', #48040, #22825, #20983, .T. ) ;
#24248=ORIENTED_EDGE ( 'NONE', *, *, #31088, .F. ) ;
#24256=DIRECTION ( 'NONE',  ( 0.000000000000000000, -1.000000000000000000, 0.000000000000000000 ) ) ;
#24260=VECTOR ( 'NONE', #14664, 1000.000000000000000 ) ;
#24261=ORIENTED_EDGE ( 'NONE', *, *, #7871, .T. ) ;
#24265=EDGE_CURVE ( 'NONE', #40248, #970, #9171, .T. ) ;
#24271=EDGE_LOOP ( 'NONE', ( #29227, #6388, #36454, #26742 ) ) ;
#24275=EDGE_CURVE ( 'NONE', #27078, #15078, #17127, .T. ) ;
#24278=ORIENTED_EDGE ( 'NONE', *, *, #31353, .F. ) ;
#24290=PLANE ( 'NONE',  #11143 ) ;
#24294=DIRECTION ( 'NONE',  ( -0.000000000000000000, -0.000000000000000000, -1.000000000000000000 ) ) ;
#24304=VECTOR ( 'NONE', #8794, 1000.000000000000000 ) ;
#24305=ORIENTED_EDGE ( 'NONE', *, *, #28027, .T. ) ;
#24312=ORIENTED_EDGE ( 'NONE', *, *, #38242, .T. ) ;
#24319=VERTEX_POINT ( 'NONE', #25086 ) ;
#24323=AXIS2_PLACEMENT_3D ( 'NONE', #5760, #29121, #44985 ) ;
#24331=ADVANCED_FACE ( 'NONE', ( #45051 ), #26595, .F. ) ;
#24334=CARTESIAN_POINT ( 'NONE',  ( 35.00000000000061107, 17.00000000000000000, -54.99999999999999289 ) ) ;
#24336=EDGE_LOOP ( 'NONE', ( #46565, #45214, #38814, #45989 ) ) ;
#24338=ORIENTED_EDGE ( 'NONE', *, *, #32113, .F. ) ;
#24344=VECTOR ( 'NONE', #9470, 1000.000000000000000 ) ;
#24346=DIRECTION ( 'NONE',  ( 0.000000000000000000, 0.000000000000000000, 1.000000000000000000 ) ) ;
#24347=LINE ( 'NONE', #4578, #21452 ) ;
#24351=CARTESIAN_POINT ( 'NONE',  ( 175.0000000000000000, 15.00000000000000000, 122.5000000000000142 ) ) ;
#24358=CARTESIAN_POINT ( 'NONE',  ( 135.0000000000003411, 16.00000000000000000, -84.99999999999998579 ) ) ;
#24361=DIRECTION ( 'NONE',  ( -0.000000000000000000, -0.000000000000000000, -1.000000000000000000 ) ) ;
#24363=LINE ( 'NONE', #44324, #48353 ) ;
#24368=CARTESIAN_POINT ( 'NONE',  ( 85.00000000000184741, 17.00000000000000000, 90.00000000000000000 ) ) ;
#24377=DIRECTION ( 'NONE',  ( 0.000000000000000000, 0.000000000000000000, -1.000000000000000000 ) ) ;
#24381=LINE ( 'NONE', #21022, #11491 ) ;
#24383=CARTESIAN_POINT ( 'NONE',  ( 85.00000000000123634, 16.00000000000000000, 30.00000000000000000 ) ) ;
#24387=EDGE_CURVE ( 'NONE', #17244, #34689, #49387, .T. ) ;
#24394=CARTESIAN_POINT ( 'NONE',  ( 164.9999999999999716, 16.00000000000000000, -114.9999999999999858 ) ) ;
#24410=DIRECTION ( 'NONE',  ( 0.000000000000000000, -0.000000000000000000, -1.000000000000000000 ) ) ;
#24417=CARTESIAN_POINT ( 'NONE',  ( -20.00000000000003197, 16.00000000000000000, -90.00000000000000000 ) ) ;
#24418=FACE_OUTER_BOUND ( 'NONE', #40721, .T. ) ;
#24434=EDGE_CURVE ( 'NONE', #46422, #50318, #46808, .T. ) ;
#24438=DIRECTION ( 'NONE',  ( 0.000000000000000000, 0.000000000000000000, 1.000000000000000000 ) ) ;
#24459=ORIENTED_EDGE ( 'NONE', *, *, #21843, .F. ) ;
#24470=ORIENTED_EDGE ( 'NONE', *, *, #37323, .F. ) ;
#24486=CARTESIAN_POINT ( 'NONE',  ( -14.99999999999876366, 17.00000000000000000, 5.000000000000004441 ) ) ;
#24495=CARTESIAN_POINT ( 'NONE',  ( -120.0000000000000426, 16.00000000000000000, -90.00000000000000000 ) ) ;
#24504=CARTESIAN_POINT ( 'NONE',  ( -65.00000000000002842, 16.00000000000000000, -114.9999999999999858 ) ) ;
#24509=CARTESIAN_POINT ( 'NONE',  ( -165.0000000000000284, 16.00000000000000000, 115.0000000000000142 ) ) ;
#24510=DIRECTION ( 'NONE',  ( 1.000000000000000000, 0.000000000000000000, 0.000000000000000000 ) ) ;
#24520=VECTOR ( 'NONE', #5408, 1000.000000000000000 ) ;
#24525=CARTESIAN_POINT ( 'NONE',  ( -69.99999999999847944, 17.00000000000000000, 60.00000000000000000 ) ) ;
#24529=EDGE_LOOP ( 'NONE', ( #186, #28016, #9845, #34454 ) ) ;
#24552=ORIENTED_EDGE ( 'NONE', *, *, #19485, .F. ) ;
#24563=DIRECTION ( 'NONE',  ( -1.000000000000000000, 0.000000000000000000, 0.000000000000000000 ) ) ;
#24564=VERTEX_POINT ( 'NONE', #3746 ) ;
#24568=ORIENTED_EDGE ( 'NONE', *, *, #40872, .T. ) ;
#24588=DIRECTION ( 'NONE',  ( 0.000000000000000000, 0.000000000000000000, -1.000000000000000000 ) ) ;
#24589=CARTESIAN_POINT ( 'NONE',  ( -19.99999999999908695, 16.00000000000000000, -24.99999999999999289 ) ) ;
#24593=DIRECTION ( 'NONE',  ( -0.000000000000000000, -1.000000000000000000, -0.000000000000000000 ) ) ;
#24595=AXIS2_PLACEMENT_3D ( 'NONE', #19362, #35045, #24237 ) ;
#24596=LINE ( 'NONE', #24358, #34747 ) ;
#24605=CARTESIAN_POINT ( 'NONE',  ( 85.00000000000184741, 16.00000000000000000, 65.00000000000000000 ) ) ;
#24606=AXIS2_PLACEMENT_3D ( 'NONE', #12554, #32586, #35934 ) ;
#24614=DIRECTION ( 'NONE',  ( 0.000000000000000000, 0.000000000000000000, -1.000000000000000000 ) ) ;
#24623=FACE_OUTER_BOUND ( 'NONE', #13038, .T. ) ;
#24625=ORIENTED_EDGE ( 'NONE', *, *, #9375, .T. ) ;
#24634=VECTOR ( 'NONE', #47729, 1000.000000000000000 ) ;
#24639=DIRECTION ( 'NONE',  ( 0.000000000000000000, 0.000000000000000000, 1.000000000000000000 ) ) ;
#24642=VECTOR ( 'NONE', #45882, 1000.000000000000000 ) ;
#24651=ORIENTED_EDGE ( 'NONE', *, *, #20390, .T. ) ;
#24653=CARTESIAN_POINT ( 'NONE',  ( 30.00000000000217781, 17.00000000000000000, 95.00000000000000000 ) ) ;
#24657=EDGE_LOOP ( 'NONE', ( #45354, #6008, #24058, #2582 ) ) ;
#24672=EDGE_CURVE ( 'NONE', #25002, #22721, #29369, .T. ) ;
#24677=CARTESIAN_POINT ( 'NONE',  ( -70.00000000000002842, 17.00000000000000000, -114.9999999999999858 ) ) ;
#24685=PLANE ( 'NONE',  #9759 ) ;
#24694=VERTEX_POINT ( 'NONE', #41422 ) ;
#24696=LINE ( 'NONE', #40591, #24304 ) ;
#24709=CARTESIAN_POINT ( 'NONE',  ( -114.9999999999978542, 17.00000000000000000, 95.00000000000000000 ) ) ;
#24719=VECTOR ( 'NONE', #2385, 1000.000000000000000 ) ;
#24726=DIRECTION ( 'NONE',  ( -1.000000000000000000, 0.000000000000000000, 0.000000000000000000 ) ) ;
#24730=CARTESIAN_POINT ( 'NONE',  ( 135.0000000000000000, 16.00000000000000000, -90.00000000000000000 ) ) ;
#24742=EDGE_CURVE ( 'NONE', #9083, #20951, #14205, .T. ) ;
#24753=LINE ( 'NONE', #4235, #8675 ) ;
#24754=EDGE_CURVE ( 'NONE', #17122, #46071, #2417, .T. ) ;
#24765=ORIENTED_EDGE ( 'NONE', *, *, #34641, .T. ) ;
#24773=ORIENTED_EDGE ( 'NONE', *, *, #7349, .T. ) ;
#24787=AXIS2_PLACEMENT_3D ( 'NONE', #17679, #5112, #8978 ) ;
#24797=DIRECTION ( 'NONE',  ( 0.000000000000000000, 0.000000000000000000, 1.000000000000000000 ) ) ;
#24805=AXIS2_PLACEMENT_3D ( 'NONE', #28249, #799, #24410 ) ;
#24813=AXIS2_PLACEMENT_3D ( 'NONE', #11595, #46190, #22878 ) ;
#24821=CARTESIAN_POINT ( 'NONE',  ( -114.9999999999987779, 17.00000000000000000, 30.00000000000000000 ) ) ;
#24824=ORIENTED_EDGE ( 'NONE', *, *, #28787, .T. ) ;
#24836=DIRECTION ( 'NONE',  ( -1.000000000000000000, -0.000000000000000000, -0.000000000000000000 ) ) ;
#24843=CARTESIAN_POINT ( 'NONE',  ( -64.99999999999940314, 16.00000000000000000, -54.99999999999999289 ) ) ;
#24854=ORIENTED_EDGE ( 'NONE', *, *, #14286, .F. ) ;
#24855=DIRECTION ( 'NONE',  ( 0.000000000000000000, -1.000000000000000000, 0.000000000000000000 ) ) ;
#24858=CARTESIAN_POINT ( 'NONE',  ( -165.0000000000000284, 17.00000000000000000, -90.00000000000000000 ) ) ;
#24861=CARTESIAN_POINT ( 'NONE',  ( -69.99999999999909051, 17.00000000000000000, -24.99999999999999289 ) ) ;
#24868=LINE ( 'NONE', #40773, #39638 ) ;
#24869=VECTOR ( 'NONE', #19233, 1000.000000000000000 ) ;
#24873=VECTOR ( 'NONE', #13602, 1000.000000000000000 ) ;
#24874=EDGE_CURVE ( 'NONE', #42829, #38545, #19070, .T. ) ;
#24878=VERTEX_POINT ( 'NONE', #19834 ) ;
#24882=EDGE_LOOP ( 'NONE', ( #10242, #10100, #984, #26658 ) ) ;
#24884=DIRECTION ( 'NONE',  ( 1.000000000000000000, 0.000000000000000000, 0.000000000000000000 ) ) ;
#24885=DIRECTION ( 'NONE',  ( -0.000000000000000000, -1.000000000000000000, -0.000000000000000000 ) ) ;
#24886=ORIENTED_EDGE ( 'NONE', *, *, #45267, .T. ) ;
#24887=ORIENTED_EDGE ( 'NONE', *, *, #34638, .T. ) ;
#24888=EDGE_LOOP ( 'NONE', ( #15640, #42397, #32032, #13753 ) ) ;
#24899=ORIENTED_EDGE ( 'NONE', *, *, #11182, .F. ) ;
#24901=DIRECTION ( 'NONE',  ( 1.000000000000000000, 0.000000000000000000, 0.000000000000000000 ) ) ;
#24902=EDGE_CURVE ( 'NONE', #8001, #36506, #35020, .T. ) ;
#24908=CARTESIAN_POINT ( 'NONE',  ( -164.9999999999984936, 17.00000000000000000, 60.00000000000000000 ) ) ;
#24911=CARTESIAN_POINT ( 'NONE',  ( -14.99999999999937472, 17.00000000000000000, -54.99999999999999289 ) ) ;
#24914=CARTESIAN_POINT ( 'NONE',  ( -165.0000000000000284, 15.00000000000000000, -114.9999999999999858 ) ) ;
#24929=CARTESIAN_POINT ( 'NONE',  ( 84.99999999999997158, 17.00000000000000000, -114.9999999999999858 ) ) ;
#24930=ADVANCED_FACE ( 'NONE', ( #40116 ), #17260, .F. ) ;
#24934=EDGE_CURVE ( 'NONE', #33254, #40248, #8811, .T. ) ;
#24935=VECTOR ( 'NONE', #29061, 1000.000000000000000 ) ;
#24938=LINE ( 'NONE', #44403, #27856 ) ;
#24941=DIRECTION ( 'NONE',  ( -0.000000000000000000, -0.000000000000000000, -1.000000000000000000 ) ) ;
#24943=ORIENTED_EDGE ( 'NONE', *, *, #39405, .T. ) ;
#24950=ADVANCED_FACE ( 'NONE', ( #4942 ), #1370, .F. ) ;
#24964=ORIENTED_EDGE ( 'NONE', *, *, #30859, .T. ) ;
#24984=DIRECTION ( 'NONE',  ( -1.000000000000000000, 0.000000000000000000, 0.000000000000000000 ) ) ;
#24986=CARTESIAN_POINT ( 'NONE',  ( -14.99999999999937472, 17.00000000000000000, -30.00000000000000000 ) ) ;
#24988=EDGE_CURVE ( 'NONE', #10222, #2212, #16251, .T. ) ;
#24991=VERTEX_POINT ( 'NONE', #28049 ) ;
#24997=VERTEX_POINT ( 'NONE', #9061 ) ;
#25002=VERTEX_POINT ( 'NONE', #20850 ) ;
#25004=DIRECTION ( 'NONE',  ( 0.000000000000000000, 0.000000000000000000, -1.000000000000000000 ) ) ;
#25007=VERTEX_POINT ( 'NONE', #44187 ) ;
#25012=CARTESIAN_POINT ( 'NONE',  ( -119.9999999999981668, 16.00000000000000000, 65.00000000000000000 ) ) ;
#25017=CARTESIAN_POINT ( 'NONE',  ( 135.0000000000003411, 16.00000000000000000, -84.99999999999998579 ) ) ;
#25028=ORIENTED_EDGE ( 'NONE', *, *, #27794, .F. ) ;
#25030=VECTOR ( 'NONE', #20603, 1000.000000000000000 ) ;
#25031=ADVANCED_FACE ( 'NONE', ( #40615 ), #42308, .F. ) ;
#25035=ADVANCED_FACE ( 'NONE', ( #1867 ), #50467, .F. ) ;
#25036=CARTESIAN_POINT ( 'NONE',  ( 85.00000000000184741, 16.00000000000000000, 90.00000000000000000 ) ) ;
#25038=LINE ( 'NONE', #44994, #6349 ) ;
#25045=CARTESIAN_POINT ( 'NONE',  ( -19.99999999999783995, 17.00000000000000000, 95.00000000000000000 ) ) ;
#25052=ORIENTED_EDGE ( 'NONE', *, *, #14680, .F. ) ;
#25059=DIRECTION ( 'NONE',  ( -0.000000000000000000, -0.000000000000000000, -1.000000000000000000 ) ) ;
#25061=EDGE_LOOP ( 'NONE', ( #12858, #32605, #48054, #18702 ) ) ;
#25063=ORIENTED_EDGE ( 'NONE', *, *, #19259, .F. ) ;
#25086=CARTESIAN_POINT ( 'NONE',  ( -114.9999999999994031, 17.00000000000000000, -30.00000000000000000 ) ) ;
#25092=EDGE_CURVE ( 'NONE', #27259, #15078, #9798, .T. ) ;
#25108=DIRECTION ( 'NONE',  ( -0.000000000000000000, -1.000000000000000000, -0.000000000000000000 ) ) ;
#25111=CARTESIAN_POINT ( 'NONE',  ( -114.9999999999987779, 17.00000000000000000, 5.000000000000004441 ) ) ;
#25114=VECTOR ( 'NONE', #32150, 1000.000000000000000 ) ;
#25121=ORIENTED_EDGE ( 'NONE', *, *, #7437, .T. ) ;
#25129=VECTOR ( 'NONE', #14797, 1000.000000000000000 ) ;
#25152=VECTOR ( 'NONE', #10731, 1000.000000000000000 ) ;
#25157=VERTEX_POINT ( 'NONE', #29557 ) ;
#25163=DIRECTION ( 'NONE',  ( -1.000000000000000000, -0.000000000000000000, -0.000000000000000000 ) ) ;
#25165=PLANE ( 'NONE',  #23068 ) ;
#25184=LINE ( 'NONE', #44160, #3713 ) ;
#25188=DIRECTION ( 'NONE',  ( 1.000000000000000000, 0.000000000000000000, 0.000000000000000000 ) ) ;
#25190=DIRECTION ( 'NONE',  ( -1.000000000000000000, -0.000000000000000000, -0.000000000000000000 ) ) ;
#25202=VERTEX_POINT ( 'NONE', #29817 ) ;
#25207=LINE ( 'NONE', #5953, #6233 ) ;
#25215=EDGE_CURVE ( 'NONE', #11044, #14334, #28189, .T. ) ;
#25219=VECTOR ( 'NONE', #14481, 1000.000000000000000 ) ;
#25221=DIRECTION ( 'NONE',  ( -0.000000000000000000, -1.000000000000000000, -0.000000000000000000 ) ) ;
#25222=ORIENTED_EDGE ( 'NONE', *, *, #18044, .F. ) ;
#25224=DIRECTION ( 'NONE',  ( 0.000000000000000000, -1.000000000000000000, 0.000000000000000000 ) ) ;
#25235=EDGE_CURVE ( 'NONE', #1878, #25941, #31795, .T. ) ;
#25236=ORIENTED_EDGE ( 'NONE', *, *, #42017, .T. ) ;
#25243=LINE ( 'NONE', #48545, #18466 ) ;
#25246=ORIENTED_EDGE ( 'NONE', *, *, #36140, .F. ) ;
#25255=ORIENTED_EDGE ( 'NONE', *, *, #29840, .T. ) ;
#25257=ORIENTED_EDGE ( 'NONE', *, *, #11177, .T. ) ;
#25269=ORIENTED_EDGE ( 'NONE', *, *, #43112, .F. ) ;
#25284=CARTESIAN_POINT ( 'NONE',  ( 35.00000000000028422, 17.00000000000000000, -84.99999999999998579 ) ) ;
#25320=VERTEX_POINT ( 'NONE', #16893 ) ;
#25325=EDGE_LOOP ( 'NONE', ( #27512, #3934, #32590, #24072 ) ) ;
#25336=VECTOR ( 'NONE', #47727, 1000.000000000000000 ) ;
#25341=DIRECTION ( 'NONE',  ( -1.000000000000000000, 0.000000000000000000, -0.000000000000000000 ) ) ;
#25345=FACE_OUTER_BOUND ( 'NONE', #9556, .T. ) ;
#25354=VECTOR ( 'NONE', #49834, 1000.000000000000000 ) ;
#25361=DIRECTION ( 'NONE',  ( -1.000000000000000000, -0.000000000000000000, -0.000000000000000000 ) ) ;
#25369=CARTESIAN_POINT ( 'NONE',  ( -14.99999999999937472, 16.00000000000000000, -30.00000000000000000 ) ) ;
#25372=ORIENTED_EDGE ( 'NONE', *, *, #17201, .F. ) ;
#25373=PLANE ( 'NONE',  #23749 ) ;
#25379=CARTESIAN_POINT ( 'NONE',  ( 29.99999999999998579, 17.00000000000000000, -114.9999999999999858 ) ) ;
#25380=FACE_OUTER_BOUND ( 'NONE', #29220, .T. ) ;
#25381=ORIENTED_EDGE ( 'NONE', *, *, #10829, .F. ) ;
#25393=AXIS2_PLACEMENT_3D ( 'NONE', #29283, #24438, #21574 ) ;
#25400=VERTEX_POINT ( 'NONE', #5836 ) ;
#25403=AXIS2_PLACEMENT_3D ( 'NONE', #8488, #24143, #3349 ) ;
#25404=ADVANCED_FACE ( 'NONE', ( #21478 ), #37167, .F. ) ;
#25407=VERTEX_POINT ( 'NONE', #50142 ) ;
#25413=ORIENTED_EDGE ( 'NONE', *, *, #15348, .F. ) ;
#25418=LINE ( 'NONE', #9013, #25442 ) ;
#25423=ORIENTED_EDGE ( 'NONE', *, *, #13890, .T. ) ;
#25430=VECTOR ( 'NONE', #44890, 1000.000000000000000 ) ;
#25438=VECTOR ( 'NONE', #6389, 1000.000000000000000 ) ;
#25440=VECTOR ( 'NONE', #39488, 1000.000000000000000 ) ;
#25442=VECTOR ( 'NONE', #32618, 1000.000000000000000 ) ;
#25443=EDGE_LOOP ( 'NONE', ( #35175, #11656, #929, #11830 ) ) ;
#25449=ORIENTED_EDGE ( 'NONE', *, *, #49405, .T. ) ;
#25450=LINE ( 'NONE', #2105, #4088 ) ;
#25471=AXIS2_PLACEMENT_3D ( 'NONE', #49419, #14305, #3505 ) ;
#25473=FACE_OUTER_BOUND ( 'NONE', #21524, .T. ) ;
#25474=DIRECTION ( 'NONE',  ( -1.000000000000000000, -0.000000000000000000, -0.000000000000000000 ) ) ;
#25481=ORIENTED_EDGE ( 'NONE', *, *, #50220, .T. ) ;
#25485=DIRECTION ( 'NONE',  ( 0.000000000000000000, 0.000000000000000000, 1.000000000000000000 ) ) ;
#25488=CARTESIAN_POINT ( 'NONE',  ( -119.9999999999994174, 17.00000000000000000, -54.99999999999999289 ) ) ;
#25509=EDGE_CURVE ( 'NONE', #38550, #325, #49143, .T. ) ;
#25525=EDGE_CURVE ( 'NONE', #37470, #8001, #22494, .T. ) ;
#25527=DIRECTION ( 'NONE',  ( 1.000000000000000000, 0.000000000000000000, 0.000000000000000000 ) ) ;
#25531=EDGE_LOOP ( 'NONE', ( #22220, #36721, #39087, #32585 ) ) ;
#25533=DIRECTION ( 'NONE',  ( 0.000000000000000000, 0.000000000000000000, 1.000000000000000000 ) ) ;
#25538=DIRECTION ( 'NONE',  ( 0.000000000000000000, 0.000000000000000000, -1.000000000000000000 ) ) ;
#25549=EDGE_CURVE ( 'NONE', #47191, #45593, #31477, .T. ) ;
#25555=EDGE_CURVE ( 'NONE', #8813, #33254, #16072, .T. ) ;
#25559=EDGE_CURVE ( 'NONE', #16843, #18731, #39683, .T. ) ;
#25565=ORIENTED_EDGE ( 'NONE', *, *, #32741, .T. ) ;
#25568=AXIS2_PLACEMENT_3D ( 'NONE', #19456, #35895, #27421 ) ;
#25590=CARTESIAN_POINT ( 'NONE',  ( 85.00000000000090949, 17.00000000000000000, -24.99999999999999289 ) ) ;
#25602=DIRECTION ( 'NONE',  ( 0.000000000000000000, 0.000000000000000000, 1.000000000000000000 ) ) ;
#25605=LINE ( 'NONE', #14036, #34384 ) ;
#25607=DIRECTION ( 'NONE',  ( -1.000000000000000000, -0.000000000000000000, -0.000000000000000000 ) ) ;
#25609=VECTOR ( 'NONE', #50218, 1000.000000000000000 ) ;
#25617=DIRECTION ( 'NONE',  ( 0.000000000000000000, 0.000000000000000000, 1.000000000000000000 ) ) ;
#25619=DIRECTION ( 'NONE',  ( 0.000000000000000000, 0.000000000000000000, 1.000000000000000000 ) ) ;
#25627=LINE ( 'NONE', #42281, #10620 ) ;
#25631=PLANE ( 'NONE',  #32819 ) ;
#25639=FACE_OUTER_BOUND ( 'NONE', #21154, .T. ) ;
#25642=DIRECTION ( 'NONE',  ( 1.000000000000000000, 0.000000000000000000, 0.000000000000000000 ) ) ;
#25646=DIRECTION ( 'NONE',  ( 0.000000000000000000, 0.000000000000000000, -1.000000000000000000 ) ) ;
#25650=VECTOR ( 'NONE', #1701, 1000.000000000000000 ) ;
#25652=CARTESIAN_POINT ( 'NONE',  ( 85.00000000000152056, 17.00000000000000000, 35.00000000000000000 ) ) ;
#25670=DIRECTION ( 'NONE',  ( 0.000000000000000000, 0.000000000000000000, 1.000000000000000000 ) ) ;
#25677=ORIENTED_EDGE ( 'NONE', *, *, #20285, .T. ) ;
#25686=DIRECTION ( 'NONE',  ( 0.000000000000000000, 0.000000000000000000, 1.000000000000000000 ) ) ;
#25687=EDGE_LOOP ( 'NONE', ( #23809, #36383, #17663, #41971 ) ) ;
#25700=ORIENTED_EDGE ( 'NONE', *, *, #43066, .F. ) ;
#25702=CARTESIAN_POINT ( 'NONE',  ( 85.00000000000213163, 17.00000000000000000, 115.0000000000000142 ) ) ;
#25712=ORIENTED_EDGE ( 'NONE', *, *, #30270, .T. ) ;
#25716=CARTESIAN_POINT ( 'NONE',  ( 85.00000000000123634, 17.00000000000000000, 5.000000000000004441 ) ) ;
#25725=VECTOR ( 'NONE', #3306, 1000.000000000000000 ) ;
#25738=LINE ( 'NONE', #37803, #17082 ) ;
#25741=ORIENTED_EDGE ( 'NONE', *, *, #27562, .T. ) ;
#25744=CARTESIAN_POINT ( 'NONE',  ( -119.9999999999994174, 17.00000000000000000, -54.99999999999999289 ) ) ;
#25760=VERTEX_POINT ( 'NONE', #1935 ) ;
#25769=DIRECTION ( 'NONE',  ( 0.000000000000000000, -0.000000000000000000, -1.000000000000000000 ) ) ;
#25770=VECTOR ( 'NONE', #14221, 1000.000000000000000 ) ;
#25794=AXIS2_PLACEMENT_3D ( 'NONE', #35583, #15808, #30969 ) ;
#25812=EDGE_CURVE ( 'NONE', #2324, #27056, #21937, .T. ) ;
#25821=DIRECTION ( 'NONE',  ( 0.000000000000000000, 0.000000000000000000, -1.000000000000000000 ) ) ;
#25830=ORIENTED_EDGE ( 'NONE', *, *, #49351, .T. ) ;
#25834=EDGE_LOOP ( 'NONE', ( #33926, #32596, #42145, #33739 ) ) ;
#25836=LINE ( 'NONE', #45552, #29533 ) ;
#25839=EDGE_CURVE ( 'NONE', #30626, #40517, #33496, .T. ) ;
#25840=CARTESIAN_POINT ( 'NONE',  ( -15.00000000000001421, 17.00000000000000000, -90.00000000000000000 ) ) ;
#25846=AXIS2_PLACEMENT_3D ( 'NONE', #24821, #5310, #35879 ) ;
#25856=ORIENTED_EDGE ( 'NONE', *, *, #3888, .T. ) ;
#25874=EDGE_CURVE ( 'NONE', #7258, #6011, #26295, .T. ) ;
#25877=EDGE_LOOP ( 'NONE', ( #15334, #32870, #18486, #17119 ) ) ;
#25885=VECTOR ( 'NONE', #40672, 1000.000000000000000 ) ;
#25890=VECTOR ( 'NONE', #1384, 1000.000000000000000 ) ;
#25896=PLANE ( 'NONE',  #26696 ) ;
#25900=FACE_OUTER_BOUND ( 'NONE', #40481, .T. ) ;
#25908=VECTOR ( 'NONE', #8406, 1000.000000000000000 ) ;
#25911=FACE_BOUND ( 'NONE', #10296, .T. ) ;
#25915=VERTEX_POINT ( 'NONE', #8321 ) ;
#25923=VECTOR ( 'NONE', #5432, 1000.000000000000000 ) ;
#25937=VERTEX_POINT ( 'NONE', #26799 ) ;
#25941=VERTEX_POINT ( 'NONE', #23960 ) ;
#25942=LINE ( 'NONE', #41577, #36931 ) ;
#25944=ORIENTED_EDGE ( 'NONE', *, *, #14632, .T. ) ;
#25952=DIRECTION ( 'NONE',  ( 0.000000000000000000, 0.000000000000000000, 1.000000000000000000 ) ) ;
#25956=EDGE_CURVE ( 'NONE', #11106, #34772, #47270, .T. ) ;
#25965=ORIENTED_EDGE ( 'NONE', *, *, #726, .F. ) ;
#25966=FACE_OUTER_BOUND ( 'NONE', #22283, .T. ) ;
#25968=ORIENTED_EDGE ( 'NONE', *, *, #15366, .F. ) ;
#25975=ORIENTED_EDGE ( 'NONE', *, *, #18580, .F. ) ;
#25991=DIRECTION ( 'NONE',  ( 1.000000000000000000, 0.000000000000000000, 0.000000000000000000 ) ) ;
#25995=VECTOR ( 'NONE', #45561, 1000.000000000000000 ) ;
#26017=ORIENTED_EDGE ( 'NONE', *, *, #35057, .F. ) ;
#26019=PLANE ( 'NONE',  #30025 ) ;
#26027=VECTOR ( 'NONE', #34503, 1000.000000000000000 ) ;
#26028=ORIENTED_EDGE ( 'NONE', *, *, #50290, .F. ) ;
#26042=VERTEX_POINT ( 'NONE', #48519 ) ;
#26055=ORIENTED_EDGE ( 'NONE', *, *, #14954, .T. ) ;
#26068=ORIENTED_EDGE ( 'NONE', *, *, #29760, .F. ) ;
#26069=EDGE_LOOP ( 'NONE', ( #30103, #21198, #13173, #35185 ) ) ;
#26072=CARTESIAN_POINT ( 'NONE',  ( -14.99999999999906919, 17.00000000000000000, -24.99999999999999289 ) ) ;
#26081=PLANE ( 'NONE',  #26728 ) ;
#26082=CARTESIAN_POINT ( 'NONE',  ( 85.00000000000152056, 17.00000000000000000, 35.00000000000000000 ) ) ;
#26088=AXIS2_PLACEMENT_3D ( 'NONE', #8827, #28321, #28570 ) ;
#26092=LINE ( 'NONE', #22250, #44508 ) ;
#26101=CARTESIAN_POINT ( 'NONE',  ( 135.0000000000021600, 17.00000000000000000, 95.00000000000000000 ) ) ;
#26107=PLANE ( 'NONE',  #31575 ) ;
#26114=VECTOR ( 'NONE', #26485, 1000.000000000000000 ) ;
#26137=ORIENTED_EDGE ( 'NONE', *, *, #21582, .T. ) ;
#26153=ADVANCED_FACE ( 'NONE', ( #25473 ), #41119, .F. ) ;
#26194=LINE ( 'NONE', #41840, #45511 ) ;
#26197=ORIENTED_EDGE ( 'NONE', *, *, #46280, .T. ) ;
#26201=ADVANCED_FACE ( 'NONE', ( #29326 ), #21617, .F. ) ;
#26213=LINE ( 'NONE', #46168, #47193 ) ;
#26220=ORIENTED_EDGE ( 'NONE', *, *, #6466, .T. ) ;
#26229=EDGE_CURVE ( 'NONE', #14126, #33150, #23390, .T. ) ;
#26234=VERTEX_POINT ( 'NONE', #42371 ) ;
#26239=VECTOR ( 'NONE', #43540, 1000.000000000000000 ) ;
#26240=EDGE_CURVE ( 'NONE', #40932, #25760, #19274, .T. ) ;
#26241=VECTOR ( 'NONE', #48798, 1000.000000000000000 ) ;
#26242=ADVANCED_FACE ( 'NONE', ( #3884 ), #34445, .F. ) ;
#26248=CARTESIAN_POINT ( 'NONE',  ( 34.99999999999997868, 17.00000000000000000, -114.9999999999999858 ) ) ;
#26249=ORIENTED_EDGE ( 'NONE', *, *, #9359, .F. ) ;
#26258=CARTESIAN_POINT ( 'NONE',  ( -120.0000000000000426, 16.00000000000000000, -114.9999999999999858 ) ) ;
#26260=LINE ( 'NONE', #2636, #30380 ) ;
#26266=CARTESIAN_POINT ( 'NONE',  ( -64.99999999999846523, 17.00000000000000000, 35.00000000000000000 ) ) ;
#26267=ORIENTED_EDGE ( 'NONE', *, *, #50290, .T. ) ;
#26269=DIRECTION ( 'NONE',  ( 1.000000000000000000, 0.000000000000000000, -0.000000000000000000 ) ) ;
#26274=ORIENTED_EDGE ( 'NONE', *, *, #49483, .T. ) ;
#26285=ORIENTED_EDGE ( 'NONE', *, *, #30744, .T. ) ;
#26291=DIRECTION ( 'NONE',  ( 0.000000000000000000, 0.000000000000000000, -1.000000000000000000 ) ) ;
#26294=ADVANCED_FACE ( 'NONE', ( #18764 ), #46444, .F. ) ;
#26295=LINE ( 'NONE', #18574, #24171 ) ;
#26308=EDGE_CURVE ( 'NONE', #21982, #45538, #15437, .T. ) ;
#26314=LINE ( 'NONE', #26562, #18792 ) ;
#26329=ORIENTED_EDGE ( 'NONE', *, *, #4381, .F. ) ;
#26335=ORIENTED_EDGE ( 'NONE', *, *, #32652, .T. ) ;
#26342=CARTESIAN_POINT ( 'NONE',  ( -64.99999999999940314, 17.00000000000000000, -54.99999999999999289 ) ) ;
#26343=AXIS2_PLACEMENT_3D ( 'NONE', #14012, #36907, #1728 ) ;
#26351=DIRECTION ( 'NONE',  ( 1.000000000000000000, 0.000000000000000000, 0.000000000000000000 ) ) ;
#26359=DIRECTION ( 'NONE',  ( 1.000000000000000000, 0.000000000000000000, 0.000000000000000000 ) ) ;
#26362=EDGE_CURVE ( 'NONE', #9086, #42678, #23128, .T. ) ;
#26370=CARTESIAN_POINT ( 'NONE',  ( 135.0000000000021600, 16.00000000000000000, 95.00000000000000000 ) ) ;
#26372=DIRECTION ( 'NONE',  ( 0.000000000000000000, 0.000000000000000000, 1.000000000000000000 ) ) ;
#26376=ORIENTED_EDGE ( 'NONE', *, *, #43825, .T. ) ;
#26382=DIRECTION ( 'NONE',  ( 1.000000000000000000, 0.000000000000000000, 0.000000000000000000 ) ) ;
#26383=CARTESIAN_POINT ( 'NONE',  ( -14.99999999999812594, 17.00000000000000000, 90.00000000000000000 ) ) ;
#26385=LINE ( 'NONE', #21780, #47728 ) ;
#26388=LINE ( 'NONE', #6133, #13572 ) ;
#26390=PLANE ( 'NONE',  #13010 ) ;
#26411=ORIENTED_EDGE ( 'NONE', *, *, #43707, .T. ) ;
#26413=EDGE_CURVE ( 'NONE', #11508, #50635, #37439, .T. ) ;
#26415=LINE ( 'NONE', #6924, #50660 ) ;
#26446=VECTOR ( 'NONE', #46646, 1000.000000000000000 ) ;
#26460=FACE_OUTER_BOUND ( 'NONE', #5048, .T. ) ;
#26474=CARTESIAN_POINT ( 'NONE',  ( -114.9999999999984652, 17.00000000000000000, 35.00000000000000000 ) ) ;
#26475=ADVANCED_FACE ( 'NONE', ( #10711 ), #37684, .F. ) ;
#26481=ORIENTED_EDGE ( 'NONE', *, *, #16868, .F. ) ;
#26483=ADVANCED_FACE ( 'NONE', ( #45081 ), #26107, .F. ) ;
#26485=DIRECTION ( 'NONE',  ( -0.000000000000000000, -1.000000000000000000, -0.000000000000000000 ) ) ;
#26487=AXIS2_PLACEMENT_3D ( 'NONE', #29211, #24855, #9700 ) ;
#26494=DIRECTION ( 'NONE',  ( 0.000000000000000000, -1.000000000000000000, 0.000000000000000000 ) ) ;
#26495=DIRECTION ( 'NONE',  ( 0.000000000000000000, 0.000000000000000000, 1.000000000000000000 ) ) ;
#26497=EDGE_LOOP ( 'NONE', ( #39111, #46085, #5822, #1929 ) ) ;
#26510=ORIENTED_EDGE ( 'NONE', *, *, #27169, .F. ) ;
#26512=PLANE ( 'NONE',  #11015 ) ;
#26513=CARTESIAN_POINT ( 'NONE',  ( 85.00000000000123634, 16.00000000000000000, 5.000000000000004441 ) ) ;
#26515=CARTESIAN_POINT ( 'NONE',  ( -64.99999999999877787, 17.00000000000000000, 5.000000000000004441 ) ) ;
#26536=VERTEX_POINT ( 'NONE', #19430 ) ;
#26555=VECTOR ( 'NONE', #45703, 1000.000000000000000 ) ;
#26560=EDGE_LOOP ( 'NONE', ( #41367, #29624, #44746, #30260 ) ) ;
#26562=CARTESIAN_POINT ( 'NONE',  ( -165.0000000000000284, 16.00000000000000000, 115.0000000000000142 ) ) ;
#26579=EDGE_CURVE ( 'NONE', #41804, #36, #3009, .T. ) ;
#26582=DIRECTION ( 'NONE',  ( -0.000000000000000000, -0.000000000000000000, -1.000000000000000000 ) ) ;
#26583=EDGE_CURVE ( 'NONE', #35690, #15972, #22769, .T. ) ;
#26595=PLANE ( 'NONE',  #3730 ) ;
#26596=ORIENTED_EDGE ( 'NONE', *, *, #92, .F. ) ;
#26606=PLANE ( 'NONE',  #28135 ) ;
#26621=ORIENTED_EDGE ( 'NONE', *, *, #47852, .F. ) ;
#26626=ORIENTED_EDGE ( 'NONE', *, *, #6195, .T. ) ;
#26628=ORIENTED_EDGE ( 'NONE', *, *, #23108, .T. ) ;
#26633=EDGE_CURVE ( 'NONE', #35523, #32541, #44273, .T. ) ;
#26641=CARTESIAN_POINT ( 'NONE',  ( 35.00000000000152767, 17.00000000000000000, 60.00000000000000000 ) ) ;
#26646=DIRECTION ( 'NONE',  ( -1.000000000000000000, -0.000000000000000000, -0.000000000000000000 ) ) ;
#26648=VERTEX_POINT ( 'NONE', #23794 ) ;
#26654=ORIENTED_EDGE ( 'NONE', *, *, #35975, .F. ) ;
#26658=ORIENTED_EDGE ( 'NONE', *, *, #28450, .F. ) ;
#26660=FACE_BOUND ( 'NONE', #38301, .T. ) ;
#26661=CARTESIAN_POINT ( 'NONE',  ( -114.9999999999978542, 17.00000000000000000, 95.00000000000000000 ) ) ;
#26668=LINE ( 'NONE', #22303, #41194 ) ;
#26670=VECTOR ( 'NONE', #28055, 1000.000000000000000 ) ;
#26671=ORIENTED_EDGE ( 'NONE', *, *, #12404, .F. ) ;
#26679=CARTESIAN_POINT ( 'NONE',  ( -114.9999999999987779, 17.00000000000000000, 5.000000000000004441 ) ) ;
#26683=ORIENTED_EDGE ( 'NONE', *, *, #20669, .T. ) ;
#26688=VECTOR ( 'NONE', #31721, 1000.000000000000000 ) ;
#26689=EDGE_LOOP ( 'NONE', ( #38694, #40858, #25700, #24248 ) ) ;
#26691=LINE ( 'NONE', #49228, #15088 ) ;
#26692=VECTOR ( 'NONE', #5963, 1000.000000000000000 ) ;
#26693=EDGE_LOOP ( 'NONE', ( #17031, #18806, #47748, #28217 ) ) ;
#26696=AXIS2_PLACEMENT_3D ( 'NONE', #41276, #45609, #34106 ) ;
#26699=DIRECTION ( 'NONE',  ( -0.000000000000000000, -0.000000000000000000, -1.000000000000000000 ) ) ;
#26701=VERTEX_POINT ( 'NONE', #36635 ) ;
#26703=DIRECTION ( 'NONE',  ( 0.000000000000000000, 0.000000000000000000, 1.000000000000000000 ) ) ;
#26720=CARTESIAN_POINT ( 'NONE',  ( 130.0000000000002842, 17.00000000000000000, -84.99999999999998579 ) ) ;
#26724=VECTOR ( 'NONE', #19379, 1000.000000000000000 ) ;
#26725=VECTOR ( 'NONE', #11311, 1000.000000000000000 ) ;
#26728=AXIS2_PLACEMENT_3D ( 'NONE', #26342, #21979, #32347 ) ;
#26739=CARTESIAN_POINT ( 'NONE',  ( 35.00000000000186162, 17.00000000000000000, 65.00000000000000000 ) ) ;
#26742=ORIENTED_EDGE ( 'NONE', *, *, #37262, .T. ) ;
#26747=ORIENTED_EDGE ( 'NONE', *, *, #10598, .F. ) ;
#26749=ORIENTED_EDGE ( 'NONE', *, *, #7485, .F. ) ;
#26763=VERTEX_POINT ( 'NONE', #40199 ) ;
#26767=ORIENTED_EDGE ( 'NONE', *, *, #8825, .T. ) ;
#26772=CARTESIAN_POINT ( 'NONE',  ( -164.9999999999994031, 17.00000000000000000, -54.99999999999999289 ) ) ;
#26787=FACE_OUTER_BOUND ( 'NONE', #11252, .T. ) ;
#26796=PLANE ( 'NONE',  #46486 ) ;
#26799=CARTESIAN_POINT ( 'NONE',  ( -15.00000000000001421, 16.00000000000000000, -114.9999999999999858 ) ) ;
#26806=EDGE_CURVE ( 'NONE', #34694, #17244, #48098, .T. ) ;
#26815=PLANE ( 'NONE',  #3339 ) ;
#26822=EDGE_CURVE ( 'NONE', #39178, #16051, #17599, .T. ) ;
#26830=LINE ( 'NONE', #30165, #21638 ) ;
#26841=ORIENTED_EDGE ( 'NONE', *, *, #46269, .F. ) ;
#26851=CARTESIAN_POINT ( 'NONE',  ( -165.0000000000000284, 16.00000000000000000, -90.00000000000000000 ) ) ;
#26852=ADVANCED_FACE ( 'NONE', ( #45018 ), #41455, .F. ) ;
#26857=DIRECTION ( 'NONE',  ( -0.000000000000000000, -0.000000000000000000, -1.000000000000000000 ) ) ;
#26858=LINE ( 'NONE', #7366, #32076 ) ;
#26869=EDGE_LOOP ( 'NONE', ( #49613, #39924, #26017, #11641 ) ) ;
#26893=VECTOR ( 'NONE', #43003, 1000.000000000000000 ) ;
#26899=CARTESIAN_POINT ( 'NONE',  ( -114.9999999999994031, 16.00000000000000000, -54.99999999999999289 ) ) ;
#26907=CARTESIAN_POINT ( 'NONE',  ( 130.0000000000002842, 17.00000000000000000, -60.00000000000000000 ) ) ;
#26908=LINE ( 'NONE', #11520, #27959 ) ;
#26926=CARTESIAN_POINT ( 'NONE',  ( -65.00000000000002842, 17.00000000000000000, -90.00000000000000000 ) ) ;
#26927=LINE ( 'NONE', #15127, #49996 ) ;
#26929=EDGE_CURVE ( 'NONE', #40517, #2086, #15280, .T. ) ;
#26942=VECTOR ( 'NONE', #14143, 1000.000000000000000 ) ;
#26944=ORIENTED_EDGE ( 'NONE', *, *, #27740, .F. ) ;
#26946=VERTEX_POINT ( 'NONE', #11418 ) ;
#26955=LINE ( 'NONE', #50001, #26725 ) ;
#26966=PLANE ( 'NONE',  #23836 ) ;
#26980=FACE_OUTER_BOUND ( 'NONE', #42156, .T. ) ;
#26981=DIRECTION ( 'NONE',  ( 1.000000000000000000, 0.000000000000000000, 0.000000000000000000 ) ) ;
#26992=LINE ( 'NONE', #7507, #791 ) ;
#26994=EDGE_CURVE ( 'NONE', #32522, #16517, #19102, .T. ) ;
#27003=CARTESIAN_POINT ( 'NONE',  ( 130.0000000000018474, 16.00000000000000000, 65.00000000000000000 ) ) ;
#27021=LINE ( 'NONE', #15472, #12061 ) ;
#27023=CARTESIAN_POINT ( 'NONE',  ( -175.0000000000000000, 0.000000000000000000, 122.5000000000000142 ) ) ;
#27030=DIRECTION ( 'NONE',  ( -1.000000000000000000, 0.000000000000000000, -0.000000000000000000 ) ) ;
#27038=ORIENTED_EDGE ( 'NONE', *, *, #14286, .T. ) ;
#27044=VECTOR ( 'NONE', #33453, 1000.000000000000000 ) ;
#27048=FACE_OUTER_BOUND ( 'NONE', #45373, .T. ) ;
#27056=VERTEX_POINT ( 'NONE', #27066 ) ;
#27062=EDGE_CURVE ( 'NONE', #10058, #22540, #7069, .T. ) ;
#27066=CARTESIAN_POINT ( 'NONE',  ( 164.9999999999999716, 17.00000000000000000, -60.00000000000001421 ) ) ;
#27078=VERTEX_POINT ( 'NONE', #24495 ) ;
#27084=VERTEX_POINT ( 'NONE', #8340 ) ;
#27088=EDGE_CURVE ( 'NONE', #4851, #15322, #32194, .T. ) ;
#27093=EDGE_CURVE ( 'NONE', #2811, #27098, #16286, .T. ) ;
#27098=VERTEX_POINT ( 'NONE', #27837 ) ;
#27101=DIRECTION ( 'NONE',  ( -0.000000000000000000, -1.000000000000000000, -0.000000000000000000 ) ) ;
#27102=EDGE_CURVE ( 'NONE', #23633, #46654, #24753, .T. ) ;
#27115=ORIENTED_EDGE ( 'NONE', *, *, #16460, .F. ) ;
#27126=ADVANCED_FACE ( 'NONE', ( #137 ), #31703, .F. ) ;
#27135=CARTESIAN_POINT ( 'NONE',  ( -14.99999999999970868, 17.00000000000000000, -84.99999999999998579 ) ) ;
#27144=ORIENTED_EDGE ( 'NONE', *, *, #12225, .T. ) ;
#27154=EDGE_CURVE ( 'NONE', #36736, #2086, #40652, .T. ) ;
#27155=ORIENTED_EDGE ( 'NONE', *, *, #10879, .T. ) ;
#27169=EDGE_CURVE ( 'NONE', #42432, #45549, #25243, .T. ) ;
#27173=DIRECTION ( 'NONE',  ( -0.000000000000000000, -1.000000000000000000, -0.000000000000000000 ) ) ;
#27176=DIRECTION ( 'NONE',  ( 0.000000000000000000, 0.000000000000000000, 1.000000000000000000 ) ) ;
#27177=CARTESIAN_POINT ( 'NONE',  ( 85.00000000000029843, 17.00000000000000000, -84.99999999999998579 ) ) ;
#27188=VECTOR ( 'NONE', #36267, 1000.000000000000000 ) ;
#27196=VECTOR ( 'NONE', #42183, 1000.000000000000000 ) ;
#27198=ORIENTED_EDGE ( 'NONE', *, *, #2203, .F. ) ;
#27213=DIRECTION ( 'NONE',  ( -1.000000000000000000, 0.000000000000000000, -0.000000000000000000 ) ) ;
#27221=ORIENTED_EDGE ( 'NONE', *, *, #49745, .F. ) ;
#27224=VECTOR ( 'NONE', #18691, 1000.000000000000000 ) ;
#27231=CARTESIAN_POINT ( 'NONE',  ( 135.0000000000012790, 16.00000000000000000, 5.000000000000004441 ) ) ;
#27259=VERTEX_POINT ( 'NONE', #30360 ) ;
#27264=ORIENTED_EDGE ( 'NONE', *, *, #24742, .T. ) ;
#27265=VECTOR ( 'NONE', #11546, 1000.000000000000000 ) ;
#27279=ORIENTED_EDGE ( 'NONE', *, *, #2428, .F. ) ;
#27281=FACE_OUTER_BOUND ( 'NONE', #9339, .T. ) ;
#27285=ORIENTED_EDGE ( 'NONE', *, *, #25956, .T. ) ;
#27288=EDGE_CURVE ( 'NONE', #7259, #26234, #2877, .T. ) ;
#27297=AXIS2_PLACEMENT_3D ( 'NONE', #24096, #7941, #47381 ) ;
#27300=FACE_OUTER_BOUND ( 'NONE', #50455, .T. ) ;
#27318=ORIENTED_EDGE ( 'NONE', *, *, #32983, .T. ) ;
#27327=VECTOR ( 'NONE', #12848, 1000.000000000000000 ) ;
#27332=EDGE_LOOP ( 'NONE', ( #21765, #25975, #22487, #18606 ) ) ;
#27345=VECTOR ( 'NONE', #11964, 1000.000000000000000 ) ;
#27355=ORIENTED_EDGE ( 'NONE', *, *, #24275, .T. ) ;
#27356=EDGE_LOOP ( 'NONE', ( #3465, #11301, #28430, #12126 ) ) ;
#27361=CARTESIAN_POINT ( 'NONE',  ( 130.0000000000015064, 16.00000000000000000, 60.00000000000000000 ) ) ;
#27379=EDGE_CURVE ( 'NONE', #30568, #16843, #38832, .T. ) ;
#27386=VERTEX_POINT ( 'NONE', #6747 ) ;
#27400=AXIS2_PLACEMENT_3D ( 'NONE', #15449, #6737, #22384 ) ;
#27414=LINE ( 'NONE', #7663, #42635 ) ;
#27416=DIRECTION ( 'NONE',  ( 0.000000000000000000, 0.000000000000000000, -1.000000000000000000 ) ) ;
#27419=CARTESIAN_POINT ( 'NONE',  ( 35.00000000000122213, 17.00000000000000000, 5.000000000000004441 ) ) ;
#27420=CARTESIAN_POINT ( 'NONE',  ( -70.00000000000002842, 17.00000000000000000, -114.9999999999999858 ) ) ;
#27421=DIRECTION ( 'NONE',  ( 1.000000000000000000, 0.000000000000000000, -0.000000000000000000 ) ) ;
#27426=VECTOR ( 'NONE', #18579, 1000.000000000000000 ) ;
#27428=CARTESIAN_POINT ( 'NONE',  ( 164.9999999999999716, 17.00000000000000000, -90.00000000000002842 ) ) ;
#27430=ORIENTED_EDGE ( 'NONE', *, *, #27623, .F. ) ;
#27433=DIRECTION ( 'NONE',  ( -1.000000000000000000, 0.000000000000000000, -0.000000000000000000 ) ) ;
#27440=ADVANCED_FACE ( 'NONE', ( #39588 ), #27533, .F. ) ;
#27444=ORIENTED_EDGE ( 'NONE', *, *, #43825, .F. ) ;
#27452=DIRECTION ( 'NONE',  ( -0.000000000000000000, -0.000000000000000000, -1.000000000000000000 ) ) ;
#27469=EDGE_CURVE ( 'NONE', #6749, #41585, #16485, .T. ) ;
#27472=ORIENTED_EDGE ( 'NONE', *, *, #46934, .F. ) ;
#27474=PLANE ( 'NONE',  #8717 ) ;
#27475=VECTOR ( 'NONE', #25485, 1000.000000000000000 ) ;
#27498=DIRECTION ( 'NONE',  ( 0.000000000000000000, -1.000000000000000000, 0.000000000000000000 ) ) ;
#27504=DIRECTION ( 'NONE',  ( -1.000000000000000000, 0.000000000000000000, 0.000000000000000000 ) ) ;
#27508=EDGE_CURVE ( 'NONE', #42902, #39284, #25184, .T. ) ;
#27512=ORIENTED_EDGE ( 'NONE', *, *, #33461, .T. ) ;
#27516=CARTESIAN_POINT ( 'NONE',  ( -19.99999999999815969, 17.00000000000000000, 90.00000000000000000 ) ) ;
#27523=VECTOR ( 'NONE', #49850, 1000.000000000000000 ) ;
#27527=DIRECTION ( 'NONE',  ( 0.000000000000000000, -1.000000000000000000, 0.000000000000000000 ) ) ;
#27533=PLANE ( 'NONE',  #11929 ) ;
#27536=ORIENTED_EDGE ( 'NONE', *, *, #41596, .F. ) ;
#27543=LINE ( 'NONE', #43179, #3487 ) ;
#27549=DIRECTION ( 'NONE',  ( 0.000000000000000000, -0.000000000000000000, -1.000000000000000000 ) ) ;
#27559=ORIENTED_EDGE ( 'NONE', *, *, #20505, .T. ) ;
#27562=EDGE_CURVE ( 'NONE', #16052, #40932, #40829, .T. ) ;
#27574=DIRECTION ( 'NONE',  ( 0.000000000000000000, -1.000000000000000000, 0.000000000000000000 ) ) ;
#27581=VECTOR ( 'NONE', #29484, 1000.000000000000000 ) ;
#27584=CARTESIAN_POINT ( 'NONE',  ( -164.9999999999990905, 17.00000000000000000, -24.99999999999999289 ) ) ;
#27587=EDGE_CURVE ( 'NONE', #23962, #27903, #1341, .T. ) ;
#27596=VERTEX_POINT ( 'NONE', #10037 ) ;
#27600=ORIENTED_EDGE ( 'NONE', *, *, #9797, .T. ) ;
#27615=ORIENTED_EDGE ( 'NONE', *, *, #38680, .F. ) ;
#27623=EDGE_CURVE ( 'NONE', #13738, #41411, #41086, .T. ) ;
#27626=ORIENTED_EDGE ( 'NONE', *, *, #12797, .F. ) ;
#27628=DIRECTION ( 'NONE',  ( -0.000000000000000000, -1.000000000000000000, -0.000000000000000000 ) ) ;
#27632=VERTEX_POINT ( 'NONE', #17740 ) ;
#27643=CARTESIAN_POINT ( 'NONE',  ( -119.9999999999981668, 17.00000000000000000, 65.00000000000000000 ) ) ;
#27657=DIRECTION ( 'NONE',  ( 1.000000000000000000, 0.000000000000000000, 0.000000000000000000 ) ) ;
#27658=ORIENTED_EDGE ( 'NONE', *, *, #34452, .T. ) ;
#27664=VERTEX_POINT ( 'NONE', #14390 ) ;
#27666=VERTEX_POINT ( 'NONE', #42583 ) ;
#27680=LINE ( 'NONE', #27428, #49542 ) ;
#27684=CARTESIAN_POINT ( 'NONE',  ( 85.00000000000213163, 17.00000000000000000, 115.0000000000000142 ) ) ;
#27689=ORIENTED_EDGE ( 'NONE', *, *, #17091, .F. ) ;
#27699=CARTESIAN_POINT ( 'NONE',  ( -69.99999999999783995, 17.00000000000000000, 95.00000000000000000 ) ) ;
#27705=CARTESIAN_POINT ( 'NONE',  ( -69.99999999999879208, 17.00000000000000000, 30.00000000000000000 ) ) ;
#27714=FACE_OUTER_BOUND ( 'NONE', #24336, .T. ) ;
#27715=DIRECTION ( 'NONE',  ( -0.000000000000000000, -0.000000000000000000, -1.000000000000000000 ) ) ;
#27728=EDGE_CURVE ( 'NONE', #17801, #7259, #11046, .T. ) ;
#27730=EDGE_CURVE ( 'NONE', #42669, #34694, #7464, .T. ) ;
#27732=DIRECTION ( 'NONE',  ( -0.000000000000000000, -1.000000000000000000, -0.000000000000000000 ) ) ;
#27734=EDGE_CURVE ( 'NONE', #41244, #24564, #14897, .T. ) ;
#27735=EDGE_CURVE ( 'NONE', #40073, #34466, #26194, .T. ) ;
#27739=DIRECTION ( 'NONE',  ( -0.000000000000000000, -1.000000000000000000, -0.000000000000000000 ) ) ;
#27740=EDGE_CURVE ( 'NONE', #343, #25937, #29792, .T. ) ;
#27743=ORIENTED_EDGE ( 'NONE', *, *, #21843, .T. ) ;
#27750=CARTESIAN_POINT ( 'NONE',  ( -119.9999999999987921, 17.00000000000000000, 30.00000000000000000 ) ) ;
#27753=VECTOR ( 'NONE', #6218, 1000.000000000000000 ) ;
#27769=DIRECTION ( 'NONE',  ( 0.000000000000000000, 0.000000000000000000, -1.000000000000000000 ) ) ;
#27771=ORIENTED_EDGE ( 'NONE', *, *, #33730, .F. ) ;
#27772=CARTESIAN_POINT ( 'NONE',  ( 80.00000000000092371, 16.00000000000000000, 0.000000000000000000 ) ) ;
#27773=DIRECTION ( 'NONE',  ( -0.000000000000000000, -1.000000000000000000, -0.000000000000000000 ) ) ;
#27780=AXIS2_PLACEMENT_3D ( 'NONE', #3229, #18877, #34558 ) ;
#27794=EDGE_CURVE ( 'NONE', #43115, #43496, #20008, .T. ) ;
#27796=VERTEX_POINT ( 'NONE', #8221 ) ;
#27810=EDGE_CURVE ( 'NONE', #26042, #16866, #8475, .T. ) ;
#27812=FACE_OUTER_BOUND ( 'NONE', #10779, .T. ) ;
#27820=PLANE ( 'NONE',  #35965 ) ;
#27830=VECTOR ( 'NONE', #16143, 1000.000000000000000 ) ;
#27837=CARTESIAN_POINT ( 'NONE',  ( 35.00000000000028422, 16.00000000000000000, -84.99999999999998579 ) ) ;
#27854=ORIENTED_EDGE ( 'NONE', *, *, #47110, .F. ) ;
#27856=VECTOR ( 'NONE', #1834, 1000.000000000000000 ) ;
#27866=VECTOR ( 'NONE', #32343, 1000.000000000000000 ) ;
#27877=CARTESIAN_POINT ( 'NONE',  ( -64.99999999999971578, 17.00000000000000000, -84.99999999999998579 ) ) ;
#27892=VECTOR ( 'NONE', #28636, 1000.000000000000000 ) ;
#27894=LINE ( 'NONE', #8885, #19074 ) ;
#27898=PLANE ( 'NONE',  #34389 ) ;
#27903=VERTEX_POINT ( 'NONE', #31324 ) ;
#27912=CARTESIAN_POINT ( 'NONE',  ( 175.0000000000000000, 15.00000000000000000, 122.5000000000000142 ) ) ;
#27925=DIRECTION ( 'NONE',  ( 1.000000000000000000, 0.000000000000000000, 0.000000000000000000 ) ) ;
#27928=LINE ( 'NONE', #39737, #25440 ) ;
#27930=CARTESIAN_POINT ( 'NONE',  ( 30.00000000000217781, 17.00000000000000000, 95.00000000000000000 ) ) ;
#27940=LINE ( 'NONE', #47893, #21612 ) ;
#27943=ORIENTED_EDGE ( 'NONE', *, *, #10378, .T. ) ;
#27945=PLANE ( 'NONE',  #23677 ) ;
#27946=CARTESIAN_POINT ( 'NONE',  ( 80.00000000000122213, 17.00000000000000000, 5.000000000000004441 ) ) ;
#27952=DIRECTION ( 'NONE',  ( -1.000000000000000000, 0.000000000000000000, -0.000000000000000000 ) ) ;
#27959=VECTOR ( 'NONE', #34124, 1000.000000000000000 ) ;
#27965=VECTOR ( 'NONE', #8137, 1000.000000000000000 ) ;
#27966=CARTESIAN_POINT ( 'NONE',  ( 85.00000000000213163, 16.00000000000000000, 95.00000000000000000 ) ) ;
#27970=DIRECTION ( 'NONE',  ( 1.000000000000000000, 0.000000000000000000, 0.000000000000000000 ) ) ;
#27972=FACE_OUTER_BOUND ( 'NONE', #18546, .T. ) ;
#27975=FACE_OUTER_BOUND ( 'NONE', #46581, .T. ) ;
#27983=DIRECTION ( 'NONE',  ( 0.000000000000000000, -1.000000000000000000, 0.000000000000000000 ) ) ;
#27989=ORIENTED_EDGE ( 'NONE', *, *, #22195, .T. ) ;
#27992=DIRECTION ( 'NONE',  ( 0.000000000000000000, 0.000000000000000000, 1.000000000000000000 ) ) ;
#27996=CARTESIAN_POINT ( 'NONE',  ( -120.0000000000000426, 17.00000000000000000, -114.9999999999999858 ) ) ;
#27999=CARTESIAN_POINT ( 'NONE',  ( 164.9999999999999716, 16.00000000000000000, 115.0000000000000142 ) ) ;
#28009=EDGE_LOOP ( 'NONE', ( #3426, #34363, #47854, #38429 ) ) ;
#28010=DIRECTION ( 'NONE',  ( -1.000000000000000000, -0.000000000000000000, -0.000000000000000000 ) ) ;
#28014=CARTESIAN_POINT ( 'NONE',  ( -19.99999999999971223, 17.00000000000000000, -84.99999999999998579 ) ) ;
#28015=EDGE_CURVE ( 'NONE', #2747, #14851, #44346, .T. ) ;
#28016=ORIENTED_EDGE ( 'NONE', *, *, #35351, .T. ) ;
#28027=EDGE_CURVE ( 'NONE', #33254, #41585, #16661, .T. ) ;
#28036=ORIENTED_EDGE ( 'NONE', *, *, #28439, .T. ) ;
#28044=ORIENTED_EDGE ( 'NONE', *, *, #44608, .T. ) ;
#28045=ORIENTED_EDGE ( 'NONE', *, *, #32712, .T. ) ;
#28049=CARTESIAN_POINT ( 'NONE',  ( 135.0000000000006253, 16.00000000000000000, -30.00000000000000000 ) ) ;
#28055=DIRECTION ( 'NONE',  ( -1.000000000000000000, -0.000000000000000000, 2.312964634635864737E-16 ) ) ;
#28062=DIRECTION ( 'NONE',  ( 0.000000000000000000, 0.000000000000000000, 1.000000000000000000 ) ) ;
#28074=ORIENTED_EDGE ( 'NONE', *, *, #30838, .T. ) ;
#28080=ADVANCED_FACE ( 'NONE', ( #15780 ), #10917, .F. ) ;
#28088=EDGE_CURVE ( 'NONE', #17655, #4851, #38644, .T. ) ;
#28098=CARTESIAN_POINT ( 'NONE',  ( -164.9999999999981526, 17.00000000000000000, 90.00000000000000000 ) ) ;
#28106=ORIENTED_EDGE ( 'NONE', *, *, #11507, .F. ) ;
#28110=EDGE_LOOP ( 'NONE', ( #46233, #15938, #20911, #26285 ) ) ;
#28116=ORIENTED_EDGE ( 'NONE', *, *, #33245, .T. ) ;
#28127=FACE_OUTER_BOUND ( 'NONE', #6479, .T. ) ;
#28130=DIRECTION ( 'NONE',  ( -1.000000000000000000, 0.000000000000000000, -3.469446951953611724E-16 ) ) ;
#28135=AXIS2_PLACEMENT_3D ( 'NONE', #34307, #7109, #29952 ) ;
#28139=EDGE_LOOP ( 'NONE', ( #23233, #1578, #43050, #19332 ) ) ;
#28144=CARTESIAN_POINT ( 'NONE',  ( 85.00000000000056843, 17.00000000000000000, -54.99999999999999289 ) ) ;
#28153=VERTEX_POINT ( 'NONE', #24504 ) ;
#28157=CARTESIAN_POINT ( 'NONE',  ( 129.9999999999999432, 16.00000000000000000, -114.9999999999999858 ) ) ;
#28179=AXIS2_PLACEMENT_3D ( 'NONE', #503, #16637, #27433 ) ;
#28189=LINE ( 'NONE', #46622, #20014 ) ;
#28198=CARTESIAN_POINT ( 'NONE',  ( -119.9999999999994174, 16.00000000000000000, -54.99999999999999289 ) ) ;
#28202=VERTEX_POINT ( 'NONE', #20386 ) ;
#28211=AXIS2_PLACEMENT_3D ( 'NONE', #21836, #13853, #9272 ) ;
#28215=CARTESIAN_POINT ( 'NONE',  ( 85.00000000000123634, 16.00000000000000000, 5.000000000000004441 ) ) ;
#28217=ORIENTED_EDGE ( 'NONE', *, *, #23613, .T. ) ;
#28218=VECTOR ( 'NONE', #48439, 1000.000000000000000 ) ;
#28230=LINE ( 'NONE', #3599, #47650 ) ;
#28233=DIRECTION ( 'NONE',  ( -1.000000000000000000, 0.000000000000000000, -0.000000000000000000 ) ) ;
#28237=LINE ( 'NONE', #24394, #20444 ) ;
#28243=DIRECTION ( 'NONE',  ( -1.000000000000000000, 0.000000000000000000, -0.000000000000000000 ) ) ;
#28249=CARTESIAN_POINT ( 'NONE',  ( 0.000000000000000000, 17.00000000000000000, 0.000000000000000000 ) ) ;
#28261=LINE ( 'NONE', #39564, #32960 ) ;
#28274=LINE ( 'NONE', #36493, #15692 ) ;
#28282=ADVANCED_FACE ( 'NONE', ( #37833 ), #26019, .F. ) ;
#28287=VECTOR ( 'NONE', #50719, 1000.000000000000000 ) ;
#28290=LINE ( 'NONE', #35765, #44756 ) ;
#28292=ORIENTED_EDGE ( 'NONE', *, *, #50341, .T. ) ;
#28296=VECTOR ( 'NONE', #23732, 1000.000000000000000 ) ;
#28300=VECTOR ( 'NONE', #39948, 1000.000000000000000 ) ;
#28302=CARTESIAN_POINT ( 'NONE',  ( -14.99999999999782041, 17.00000000000000000, 95.00000000000000000 ) ) ;
#28305=ORIENTED_EDGE ( 'NONE', *, *, #21121, .T. ) ;
#28307=ORIENTED_EDGE ( 'NONE', *, *, #38137, .F. ) ;
#28308=CARTESIAN_POINT ( 'NONE',  ( 135.0000000000015632, 17.00000000000000000, 35.00000000000000000 ) ) ;
#28311=AXIS2_PLACEMENT_3D ( 'NONE', #6978, #26981, #31356 ) ;
#28314=CARTESIAN_POINT ( 'NONE',  ( 79.99999999999997158, 17.00000000000000000, -90.00000000000000000 ) ) ;
#28321=DIRECTION ( 'NONE',  ( -1.000000000000000000, 0.000000000000000000, 0.000000000000000000 ) ) ;
#28326=DIRECTION ( 'NONE',  ( 0.000000000000000000, 0.000000000000000000, -1.000000000000000000 ) ) ;
#28328=DIRECTION ( 'NONE',  ( -1.000000000000000000, -0.000000000000000000, 4.625929269271687073E-16 ) ) ;
#28332=EDGE_CURVE ( 'NONE', #375, #19127, #2404, .T. ) ;
#28346=AXIS2_PLACEMENT_3D ( 'NONE', #33347, #30491, #21782 ) ;
#28354=AXIS2_PLACEMENT_3D ( 'NONE', #32929, #21099, #33430 ) ;
#28359=VECTOR ( 'NONE', #17850, 1000.000000000000000 ) ;
#28384=CARTESIAN_POINT ( 'NONE',  ( 0.000000000000000000, 0.000000000000000000, 0.000000000000000000 ) ) ;
#28387=PLANE ( 'NONE',  #30188 ) ;
#28394=CARTESIAN_POINT ( 'NONE',  ( -69.99999999999879208, 17.00000000000000000, 5.000000000000004441 ) ) ;
#28397=DIRECTION ( 'NONE',  ( 1.000000000000000000, 0.000000000000000000, -4.625929269271584521E-16 ) ) ;
#28402=DIRECTION ( 'NONE',  ( 0.000000000000000000, 0.000000000000000000, 1.000000000000000000 ) ) ;
#28411=ORIENTED_EDGE ( 'NONE', *, *, #38074, .F. ) ;
#28412=DIRECTION ( 'NONE',  ( -1.000000000000000000, -0.000000000000000000, -0.000000000000000000 ) ) ;
#28414=AXIS2_PLACEMENT_3D ( 'NONE', #37092, #17813, #10379 ) ;
#28422=DIRECTION ( 'NONE',  ( -0.000000000000000000, -0.000000000000000000, -1.000000000000000000 ) ) ;
#28430=ORIENTED_EDGE ( 'NONE', *, *, #20226, .F. ) ;
#28431=CARTESIAN_POINT ( 'NONE',  ( -69.99999999999879208, 17.00000000000000000, 30.00000000000000000 ) ) ;
#28433=DIRECTION ( 'NONE',  ( 1.000000000000000000, 0.000000000000000000, 0.000000000000000000 ) ) ;
#28439=EDGE_CURVE ( 'NONE', #24182, #38545, #30115, .T. ) ;
#28442=ADVANCED_FACE ( 'NONE', ( #27281 ), #49804, .F. ) ;
#28450=EDGE_CURVE ( 'NONE', #39659, #2507, #18548, .T. ) ;
#28451=DIRECTION ( 'NONE',  ( -1.000000000000000000, -0.000000000000000000, 2.312964634635864737E-16 ) ) ;
#28453=DIRECTION ( 'NONE',  ( -0.000000000000000000, -1.000000000000000000, -0.000000000000000000 ) ) ;
#28458=LINE ( 'NONE', #40251, #11080 ) ;
#28459=CARTESIAN_POINT ( 'NONE',  ( 135.0000000000009663, 17.00000000000000000, -24.99999999999999289 ) ) ;
#28472=ORIENTED_EDGE ( 'NONE', *, *, #29293, .F. ) ;
#28487=DIRECTION ( 'NONE',  ( 1.000000000000000000, 0.000000000000000000, 0.000000000000000000 ) ) ;
#28489=ORIENTED_EDGE ( 'NONE', *, *, #740, .F. ) ;
#28492=PLANE ( 'NONE',  #49120 ) ;
#28506=PLANE ( 'NONE',  #5650 ) ;
#28509=CARTESIAN_POINT ( 'NONE',  ( 0.000000000000000000, 17.00000000000000000, 0.000000000000000000 ) ) ;
#28515=DIRECTION ( 'NONE',  ( -2.312964634635843537E-16, 0.000000000000000000, -1.000000000000000000 ) ) ;
#28518=LINE ( 'NONE', #23905, #245 ) ;
#28522=ORIENTED_EDGE ( 'NONE', *, *, #40565, .F. ) ;
#28524=DIRECTION ( 'NONE',  ( -0.000000000000000000, -1.000000000000000000, -0.000000000000000000 ) ) ;
#28529=ORIENTED_EDGE ( 'NONE', *, *, #10486, .T. ) ;
#28531=PLANE ( 'NONE',  #32282 ) ;
#28534=ORIENTED_EDGE ( 'NONE', *, *, #46925, .F. ) ;
#28537=EDGE_CURVE ( 'NONE', #19596, #34874, #28290, .T. ) ;
#28538=EDGE_LOOP ( 'NONE', ( #37043, #23518, #6048, #50062 ) ) ;
#28554=CARTESIAN_POINT ( 'NONE',  ( 35.00000000000152767, 17.00000000000000000, 35.00000000000000000 ) ) ;
#28567=EDGE_CURVE ( 'NONE', #35690, #11870, #16492, .T. ) ;
#28570=DIRECTION ( 'NONE',  ( 0.000000000000000000, 0.000000000000000000, 1.000000000000000000 ) ) ;
#28580=ORIENTED_EDGE ( 'NONE', *, *, #5268, .F. ) ;
#28588=CARTESIAN_POINT ( 'NONE',  ( -164.9999999999994031, 17.00000000000000000, -54.99999999999999289 ) ) ;
#28591=ORIENTED_EDGE ( 'NONE', *, *, #4921, .T. ) ;
#28594=CARTESIAN_POINT ( 'NONE',  ( 85.00000000000123634, 17.00000000000000000, 5.000000000000004441 ) ) ;
#28614=LINE ( 'NONE', #24525, #15463 ) ;
#28628=EDGE_CURVE ( 'NONE', #33142, #15045, #40100, .T. ) ;
#28634=VERTEX_POINT ( 'NONE', #16732 ) ;
#28636=DIRECTION ( 'NONE',  ( -0.000000000000000000, -1.000000000000000000, -0.000000000000000000 ) ) ;
#28645=VERTEX_POINT ( 'NONE', #47242 ) ;
#28653=ORIENTED_EDGE ( 'NONE', *, *, #49759, .T. ) ;
#28658=ORIENTED_EDGE ( 'NONE', *, *, #26929, .F. ) ;
#28660=EDGE_CURVE ( 'NONE', #6936, #24694, #47495, .T. ) ;
#28667=CARTESIAN_POINT ( 'NONE',  ( 0.000000000000000000, 17.00000000000000000, 0.000000000000000000 ) ) ;
#28674=EDGE_CURVE ( 'NONE', #37527, #46181, #45157, .T. ) ;
#28689=VECTOR ( 'NONE', #49292, 1000.000000000000000 ) ;
#28692=VECTOR ( 'NONE', #10898, 1000.000000000000000 ) ;
#28718=ADVANCED_FACE ( 'NONE', ( #41597 ), #1349, .F. ) ;
#28722=ORIENTED_EDGE ( 'NONE', *, *, #338, .F. ) ;
#28752=PLANE ( 'NONE',  #18260 ) ;
#28760=DIRECTION ( 'NONE',  ( 1.000000000000000000, 0.000000000000000000, 0.000000000000000000 ) ) ;
#28787=EDGE_CURVE ( 'NONE', #16006, #41417, #30821, .T. ) ;
#28790=EDGE_CURVE ( 'NONE', #46654, #50635, #26955, .T. ) ;
#28796=ORIENTED_EDGE ( 'NONE', *, *, #12158, .F. ) ;
#28798=VECTOR ( 'NONE', #7539, 1000.000000000000000 ) ;
#28802=CARTESIAN_POINT ( 'NONE',  ( 35.00000000000152767, 17.00000000000000000, 60.00000000000000000 ) ) ;
#28803=VECTOR ( 'NONE', #1494, 1000.000000000000000 ) ;
#28814=CARTESIAN_POINT ( 'NONE',  ( 30.00000000000153833, 16.00000000000000000, 35.00000000000000000 ) ) ;
#28819=FACE_OUTER_BOUND ( 'NONE', #35178, .T. ) ;
#28821=LINE ( 'NONE', #40867, #38735 ) ;
#28822=ORIENTED_EDGE ( 'NONE', *, *, #8634, .T. ) ;
#28842=EDGE_LOOP ( 'NONE', ( #11326, #40909, #5682, #16495 ) ) ;
#28847=EDGE_CURVE ( 'NONE', #13654, #25400, #2833, .T. ) ;
#28860=DIRECTION ( 'NONE',  ( 0.000000000000000000, -1.000000000000000000, 0.000000000000000000 ) ) ;
#28870=EDGE_LOOP ( 'NONE', ( #45984, #37066, #12808, #23446 ) ) ;
#28886=FACE_OUTER_BOUND ( 'NONE', #20772, .T. ) ;
#28897=CARTESIAN_POINT ( 'NONE',  ( -115.0000000000000284, 16.00000000000000000, -114.9999999999999858 ) ) ;
#28907=VERTEX_POINT ( 'NONE', #45916 ) ;
#28908=VECTOR ( 'NONE', #37956, 1000.000000000000000 ) ;
#28917=ORIENTED_EDGE ( 'NONE', *, *, #15005, .F. ) ;
#28919=AXIS2_PLACEMENT_3D ( 'NONE', #27877, #34827, #35339 ) ;
#28923=EDGE_LOOP ( 'NONE', ( #25255, #40786, #5263, #9867 ) ) ;
#28946=PLANE ( 'NONE',  #12249 ) ;
#28969=ADVANCED_FACE ( 'NONE', ( #27972 ), #27474, .F. ) ;
#28983=DIRECTION ( 'NONE',  ( -0.000000000000000000, -1.000000000000000000, -0.000000000000000000 ) ) ;
#28984=DIRECTION ( 'NONE',  ( -0.000000000000000000, -1.000000000000000000, -0.000000000000000000 ) ) ;
#28988=CARTESIAN_POINT ( 'NONE',  ( -69.99999999999909051, 17.00000000000000000, -24.99999999999999289 ) ) ;
#29005=VECTOR ( 'NONE', #3017, 1000.000000000000000 ) ;
#29015=CARTESIAN_POINT ( 'NONE',  ( -165.0000000000000284, 17.00000000000000000, -114.9999999999999858 ) ) ;
#29032=CARTESIAN_POINT ( 'NONE',  ( -114.9999999999987779, 17.00000000000000000, 30.00000000000000000 ) ) ;
#29040=ORIENTED_EDGE ( 'NONE', *, *, #12422, .F. ) ;
#29056=ORIENTED_EDGE ( 'NONE', *, *, #27093, .F. ) ;
#29057=ADVANCED_FACE ( 'NONE', ( #48929 ), #8981, .F. ) ;
#29061=DIRECTION ( 'NONE',  ( -0.000000000000000000, -1.000000000000000000, -0.000000000000000000 ) ) ;
#29066=LINE ( 'NONE', #12900, #7302 ) ;
#29071=EDGE_CURVE ( 'NONE', #1528, #28645, #37463, .T. ) ;
#29075=LINE ( 'NONE', #44695, #46887 ) ;
#29076=ORIENTED_EDGE ( 'NONE', *, *, #27734, .F. ) ;
#29096=LINE ( 'NONE', #25488, #3327 ) ;
#29105=ORIENTED_EDGE ( 'NONE', *, *, #42907, .F. ) ;
#29114=EDGE_CURVE ( 'NONE', #3719, #37462, #17431, .T. ) ;
#29121=DIRECTION ( 'NONE',  ( 0.000000000000000000, 0.000000000000000000, -1.000000000000000000 ) ) ;
#29123=ORIENTED_EDGE ( 'NONE', *, *, #38548, .F. ) ;
#29132=DIRECTION ( 'NONE',  ( -0.000000000000000000, -1.000000000000000000, -0.000000000000000000 ) ) ;
#29139=EDGE_CURVE ( 'NONE', #24319, #41244, #9983, .T. ) ;
#29144=CARTESIAN_POINT ( 'NONE',  ( -64.99999999999909051, 16.00000000000000000, -24.99999999999999289 ) ) ;
#29155=CARTESIAN_POINT ( 'NONE',  ( 29.99999999999998579, 17.00000000000000000, -114.9999999999999858 ) ) ;
#29175=ADVANCED_FACE ( 'NONE', ( #7410 ), #22790, .F. ) ;
#29192=DIRECTION ( 'NONE',  ( -0.000000000000000000, -0.000000000000000000, -1.000000000000000000 ) ) ;
#29196=VECTOR ( 'NONE', #17449, 1000.000000000000000 ) ;
#29199=DIRECTION ( 'NONE',  ( 0.000000000000000000, -1.000000000000000000, 0.000000000000000000 ) ) ;
#29201=DIRECTION ( 'NONE',  ( 0.000000000000000000, -1.000000000000000000, 0.000000000000000000 ) ) ;
#29207=CARTESIAN_POINT ( 'NONE',  ( 0.000000000000000000, 17.00000000000000000, 0.000000000000000000 ) ) ;
#29209=DIRECTION ( 'NONE',  ( -1.000000000000000000, -0.000000000000000000, 4.625929269271635797E-16 ) ) ;
#29211=CARTESIAN_POINT ( 'NONE',  ( 0.000000000000000000, 17.00000000000000000, 0.000000000000000000 ) ) ;
#29213=PLANE ( 'NONE',  #45816 ) ;
#29220=EDGE_LOOP ( 'NONE', ( #42041, #26137, #10425, #7030 ) ) ;
#29227=ORIENTED_EDGE ( 'NONE', *, *, #37194, .T. ) ;
#29231=CARTESIAN_POINT ( 'NONE',  ( 0.000000000000000000, 17.00000000000000000, 0.000000000000000000 ) ) ;
#29243=ORIENTED_EDGE ( 'NONE', *, *, #36979, .T. ) ;
#29244=CARTESIAN_POINT ( 'NONE',  ( 0.000000000000000000, 17.00000000000000000, 0.000000000000000000 ) ) ;
#29283=CARTESIAN_POINT ( 'NONE',  ( -14.99999999999812594, 17.00000000000000000, 65.00000000000000000 ) ) ;
#29293=EDGE_CURVE ( 'NONE', #41952, #17244, #30243, .T. ) ;
#29297=LINE ( 'NONE', #49244, #36312 ) ;
#29318=CARTESIAN_POINT ( 'NONE',  ( 164.9999999999999716, 17.00000000000000000, 115.0000000000000142 ) ) ;
#29326=FACE_OUTER_BOUND ( 'NONE', #22916, .T. ) ;
#29331=CARTESIAN_POINT ( 'NONE',  ( 175.0000000000000000, 15.00000000000000000, -122.5000000000000000 ) ) ;
#29349=ORIENTED_EDGE ( 'NONE', *, *, #37194, .F. ) ;
#29353=EDGE_CURVE ( 'NONE', #41804, #7870, #19706, .T. ) ;
#29354=ADVANCED_FACE ( 'NONE', ( #38967 ), #19948, .F. ) ;
#29356=ORIENTED_EDGE ( 'NONE', *, *, #25559, .T. ) ;
#29358=CARTESIAN_POINT ( 'NONE',  ( -114.9999999999987779, 16.00000000000000000, 30.00000000000000000 ) ) ;
#29360=ORIENTED_EDGE ( 'NONE', *, *, #16153, .F. ) ;
#29367=VERTEX_POINT ( 'NONE', #21461 ) ;
#29369=LINE ( 'NONE', #17814, #33908 ) ;
#29370=ORIENTED_EDGE ( 'NONE', *, *, #4593, .T. ) ;
#29392=ORIENTED_EDGE ( 'NONE', *, *, #30646, .T. ) ;
#29404=CARTESIAN_POINT ( 'NONE',  ( -114.9999999999991047, 17.00000000000000000, -24.99999999999999289 ) ) ;
#29419=VERTEX_POINT ( 'NONE', #9668 ) ;
#29422=LINE ( 'NONE', #5820, #37029 ) ;
#29436=DIRECTION ( 'NONE',  ( 1.000000000000000000, 0.000000000000000000, 0.000000000000000000 ) ) ;
#29447=DIRECTION ( 'NONE',  ( -0.000000000000000000, -0.000000000000000000, 1.000000000000000000 ) ) ;
#29450=CARTESIAN_POINT ( 'NONE',  ( 35.00000000000091660, 17.00000000000000000, -24.99999999999999289 ) ) ;
#29455=LINE ( 'NONE', #32821, #30557 ) ;
#29478=DIRECTION ( 'NONE',  ( 1.000000000000000000, 0.000000000000000000, -0.000000000000000000 ) ) ;
#29482=CARTESIAN_POINT ( 'NONE',  ( 0.000000000000000000, 17.00000000000000000, 0.000000000000000000 ) ) ;
#29484=DIRECTION ( 'NONE',  ( -0.000000000000000000, -1.000000000000000000, -0.000000000000000000 ) ) ;
#29490=ADVANCED_FACE ( 'NONE', ( #40477 ), #48118, .F. ) ;
#29491=CARTESIAN_POINT ( 'NONE',  ( -114.9999999999991047, 17.00000000000000000, 0.000000000000000000 ) ) ;
#29495=CARTESIAN_POINT ( 'NONE',  ( -70.00000000000002842, 16.00000000000000000, -114.9999999999999858 ) ) ;
#29501=CARTESIAN_POINT ( 'NONE',  ( 135.0000000000012790, 17.00000000000000000, 30.00000000000000000 ) ) ;
#29514=CARTESIAN_POINT ( 'NONE',  ( -14.99999999999937472, 17.00000000000000000, -54.99999999999999289 ) ) ;
#29516=CARTESIAN_POINT ( 'NONE',  ( 85.00000000000090949, 17.00000000000000000, 0.000000000000000000 ) ) ;
#29524=LINE ( 'NONE', #24677, #384 ) ;
#29525=CARTESIAN_POINT ( 'NONE',  ( 85.00000000000090949, 17.00000000000000000, -24.99999999999999289 ) ) ;
#29527=VECTOR ( 'NONE', #7702, 1000.000000000000000 ) ;
#29533=VECTOR ( 'NONE', #22483, 1000.000000000000000 ) ;
#29543=PLANE ( 'NONE',  #40970 ) ;
#29548=FACE_OUTER_BOUND ( 'NONE', #9575, .T. ) ;
#29552=VERTEX_POINT ( 'NONE', #37403 ) ;
#29557=CARTESIAN_POINT ( 'NONE',  ( 130.0000000000018474, 17.00000000000000000, 90.00000000000000000 ) ) ;
#29560=DIRECTION ( 'NONE',  ( -0.000000000000000000, -1.000000000000000000, -0.000000000000000000 ) ) ;
#29562=ORIENTED_EDGE ( 'NONE', *, *, #9663, .T. ) ;
#29570=CARTESIAN_POINT ( 'NONE',  ( -164.9999999999990905, 17.00000000000000000, 0.000000000000000000 ) ) ;
#29588=DIRECTION ( 'NONE',  ( 0.000000000000000000, 0.000000000000000000, 1.000000000000000000 ) ) ;
#29590=FACE_OUTER_BOUND ( 'NONE', #264, .T. ) ;
#29604=DIRECTION ( 'NONE',  ( 1.000000000000000000, 0.000000000000000000, 0.000000000000000000 ) ) ;
#29606=CARTESIAN_POINT ( 'NONE',  ( -69.99999999999940314, 16.00000000000000000, -54.99999999999999289 ) ) ;
#29624=ORIENTED_EDGE ( 'NONE', *, *, #28439, .F. ) ;
#29626=CARTESIAN_POINT ( 'NONE',  ( -119.9999999999997158, 17.00000000000000000, -84.99999999999998579 ) ) ;
#29627=DIRECTION ( 'NONE',  ( 0.000000000000000000, 0.000000000000000000, -1.000000000000000000 ) ) ;
#29641=EDGE_CURVE ( 'NONE', #4392, #50192, #5190, .T. ) ;
#29642=CARTESIAN_POINT ( 'NONE',  ( 164.9999999999999716, 17.00000000000000000, 59.99999999999999289 ) ) ;
#29645=VECTOR ( 'NONE', #46341, 1000.000000000000000 ) ;
#29650=CARTESIAN_POINT ( 'NONE',  ( 85.00000000000152056, 16.00000000000000000, 35.00000000000000000 ) ) ;
#29661=ORIENTED_EDGE ( 'NONE', *, *, #5113, .F. ) ;
#29663=VECTOR ( 'NONE', #30319, 1000.000000000000000 ) ;
#29666=VECTOR ( 'NONE', #5469, 1000.000000000000000 ) ;
#29670=ORIENTED_EDGE ( 'NONE', *, *, #6692, .T. ) ;
#29675=VERTEX_POINT ( 'NONE', #42717 ) ;
#29681=ORIENTED_EDGE ( 'NONE', *, *, #10300, .T. ) ;
#29683=DIRECTION ( 'NONE',  ( 0.000000000000000000, 0.000000000000000000, -1.000000000000000000 ) ) ;
#29686=EDGE_CURVE ( 'NONE', #18457, #39326, #32651, .T. ) ;
#29689=LINE ( 'NONE', #7108, #34078 ) ;
#29694=EDGE_CURVE ( 'NONE', #20602, #41952, #3739, .T. ) ;
#29701=VECTOR ( 'NONE', #33925, 1000.000000000000000 ) ;
#29703=CARTESIAN_POINT ( 'NONE',  ( 35.00000000000186162, 17.00000000000000000, 65.00000000000000000 ) ) ;
#29706=ADVANCED_FACE ( 'NONE', ( #29548 ), #17251, .F. ) ;
#29724=CARTESIAN_POINT ( 'NONE',  ( 85.00000000000056843, 17.00000000000000000, -30.00000000000000000 ) ) ;
#29734=CARTESIAN_POINT ( 'NONE',  ( 85.00000000000213163, 17.00000000000000000, 95.00000000000000000 ) ) ;
#29735=EDGE_LOOP ( 'NONE', ( #29056, #45985, #7282, #2691 ) ) ;
#29738=VERTEX_POINT ( 'NONE', #2108 ) ;
#29741=LINE ( 'NONE', #45357, #25438 ) ;
#29744=ORIENTED_EDGE ( 'NONE', *, *, #26413, .T. ) ;
#29749=FACE_BOUND ( 'NONE', #1034, .T. ) ;
#29760=EDGE_CURVE ( 'NONE', #21529, #25320, #10052, .T. ) ;
#29792=LINE ( 'NONE', #50241, #33291 ) ;
#29810=PLANE ( 'NONE',  #39505 ) ;
#29817=CARTESIAN_POINT ( 'NONE',  ( -119.9999999999978400, 16.00000000000000000, 115.0000000000000142 ) ) ;
#29840=EDGE_CURVE ( 'NONE', #27056, #35523, #48408, .T. ) ;
#29854=EDGE_LOOP ( 'NONE', ( #11275, #18987, #24899, #24765 ) ) ;
#29855=LINE ( 'NONE', #46219, #10373 ) ;
#29857=CARTESIAN_POINT ( 'NONE',  ( 35.00000000000061107, 17.00000000000000000, -54.99999999999999289 ) ) ;
#29858=VERTEX_POINT ( 'NONE', #4612 ) ;
#29864=CARTESIAN_POINT ( 'NONE',  ( 85.00000000000213163, 16.00000000000000000, 115.0000000000000142 ) ) ;
#29865=ORIENTED_EDGE ( 'NONE', *, *, #26994, .F. ) ;
#29873=CARTESIAN_POINT ( 'NONE',  ( 30.00000000000123279, 17.00000000000000000, 5.000000000000004441 ) ) ;
#29879=FACE_OUTER_BOUND ( 'NONE', #7581, .T. ) ;
#29880=DIRECTION ( 'NONE',  ( 0.000000000000000000, 1.000000000000000000, 0.000000000000000000 ) ) ;
#29897=LINE ( 'NONE', #42194, #28692 ) ;
#29907=LINE ( 'NONE', #37628, #16658 ) ;
#29923=ADVANCED_FACE ( 'NONE', ( #13048 ), #12296, .F. ) ;
#29925=DIRECTION ( 'NONE',  ( -0.000000000000000000, -1.000000000000000000, -0.000000000000000000 ) ) ;
#29930=EDGE_CURVE ( 'NONE', #22771, #42166, #5091, .T. ) ;
#29932=DIRECTION ( 'NONE',  ( 1.000000000000000000, 0.000000000000000000, 0.000000000000000000 ) ) ;
#29941=ORIENTED_EDGE ( 'NONE', *, *, #24742, .F. ) ;
#29951=CARTESIAN_POINT ( 'NONE',  ( 35.00000000000091660, 17.00000000000000000, -24.99999999999999289 ) ) ;
#29952=DIRECTION ( 'NONE',  ( -1.000000000000000000, 0.000000000000000000, -0.000000000000000000 ) ) ;
#29962=VERTEX_POINT ( 'NONE', #3043 ) ;
#29963=FACE_OUTER_BOUND ( 'NONE', #10996, .T. ) ;
#29983=LINE ( 'NONE', #45091, #39365 ) ;
#29994=DIRECTION ( 'NONE',  ( 0.000000000000000000, -1.000000000000000000, 0.000000000000000000 ) ) ;
#30005=CARTESIAN_POINT ( 'NONE',  ( 80.00000000000028422, 17.00000000000000000, -84.99999999999998579 ) ) ;
#30010=ADVANCED_FACE ( 'NONE', ( #49953 ), #42048, .F. ) ;
#30013=FACE_BOUND ( 'NONE', #37907, .T. ) ;
#30014=CARTESIAN_POINT ( 'NONE',  ( -164.9999999999984936, 17.00000000000000000, 35.00000000000000000 ) ) ;
#30025=AXIS2_PLACEMENT_3D ( 'NONE', #41148, #33722, #41659 ) ;
#30038=ORIENTED_EDGE ( 'NONE', *, *, #2276, .T. ) ;
#30040=ORIENTED_EDGE ( 'NONE', *, *, #42017, .F. ) ;
#30043=DIRECTION ( 'NONE',  ( -0.000000000000000000, -1.000000000000000000, -0.000000000000000000 ) ) ;
#30050=ORIENTED_EDGE ( 'NONE', *, *, #48527, .T. ) ;
#30051=DIRECTION ( 'NONE',  ( -1.000000000000000000, -0.000000000000000000, -0.000000000000000000 ) ) ;
#30068=CARTESIAN_POINT ( 'NONE',  ( 80.00000000000216005, 16.00000000000000000, 95.00000000000000000 ) ) ;
#30070=DIRECTION ( 'NONE',  ( -1.000000000000000000, 0.000000000000000000, 0.000000000000000000 ) ) ;
#30077=ORIENTED_EDGE ( 'NONE', *, *, #27562, .F. ) ;
#30083=ORIENTED_EDGE ( 'NONE', *, *, #94, .F. ) ;
#30093=LINE ( 'NONE', #14432, #3142 ) ;
#30097=VERTEX_POINT ( 'NONE', #26661 ) ;
#30103=ORIENTED_EDGE ( 'NONE', *, *, #45622, .T. ) ;
#30110=DIRECTION ( 'NONE',  ( 1.000000000000000000, 0.000000000000000000, -0.000000000000000000 ) ) ;
#30115=LINE ( 'NONE', #42400, #45544 ) ;
#30118=PLANE ( 'NONE',  #15327 ) ;
#30128=DIRECTION ( 'NONE',  ( -0.000000000000000000, -1.000000000000000000, -0.000000000000000000 ) ) ;
#30142=CARTESIAN_POINT ( 'NONE',  ( 135.0000000000015632, 16.00000000000000000, 35.00000000000000000 ) ) ;
#30148=CARTESIAN_POINT ( 'NONE',  ( 135.0000000000009663, 17.00000000000000000, -24.99999999999999289 ) ) ;
#30154=VECTOR ( 'NONE', #36675, 1000.000000000000000 ) ;
#30155=CARTESIAN_POINT ( 'NONE',  ( 85.00000000000184741, 17.00000000000000000, 65.00000000000000000 ) ) ;
#30165=CARTESIAN_POINT ( 'NONE',  ( 85.00000000000090949, 16.00000000000000000, -24.99999999999999289 ) ) ;
#30167=ORIENTED_EDGE ( 'NONE', *, *, #4527, .F. ) ;
#30177=VERTEX_POINT ( 'NONE', #26907 ) ;
#30183=ORIENTED_EDGE ( 'NONE', *, *, #32402, .F. ) ;
#30188=AXIS2_PLACEMENT_3D ( 'NONE', #25045, #28130, #4523 ) ;
#30189=DIRECTION ( 'NONE',  ( 0.000000000000000000, 0.000000000000000000, -1.000000000000000000 ) ) ;
#30193=CARTESIAN_POINT ( 'NONE',  ( -69.99999999999972999, 17.00000000000000000, -84.99999999999998579 ) ) ;
#30198=ADVANCED_FACE ( 'NONE', ( #46873 ), #43056, .F. ) ;
#30201=EDGE_LOOP ( 'NONE', ( #49903, #43810, #37389, #4037 ) ) ;
#30211=ORIENTED_EDGE ( 'NONE', *, *, #35568, .F. ) ;
#30223=AXIS2_PLACEMENT_3D ( 'NONE', #2919, #18572, #34248 ) ;
#30224=VECTOR ( 'NONE', #5078, 1000.000000000000000 ) ;
#30235=ORIENTED_EDGE ( 'NONE', *, *, #10458, .F. ) ;
#30238=DIRECTION ( 'NONE',  ( -1.096345236817341200E-13, 0.000000000000000000, 1.000000000000000000 ) ) ;
#30241=ORIENTED_EDGE ( 'NONE', *, *, #46124, .T. ) ;
#30242=ADVANCED_FACE ( 'NONE', ( #1247 ), #5574, .F. ) ;
#30243=LINE ( 'NONE', #34355, #25152 ) ;
#30244=CARTESIAN_POINT ( 'NONE',  ( -69.99999999999783995, 17.00000000000000000, 95.00000000000000000 ) ) ;
#30253=ORIENTED_EDGE ( 'NONE', *, *, #45604, .F. ) ;
#30260=ORIENTED_EDGE ( 'NONE', *, *, #11716, .T. ) ;
#30270=EDGE_CURVE ( 'NONE', #23377, #418, #4580, .T. ) ;
#30280=CARTESIAN_POINT ( 'NONE',  ( -114.9999999999997158, 17.00000000000000000, -84.99999999999998579 ) ) ;
#30294=VERTEX_POINT ( 'NONE', #45055 ) ;
#30295=CARTESIAN_POINT ( 'NONE',  ( 164.9999999999999716, 17.00000000000000000, -85.00000000000001421 ) ) ;
#30298=CARTESIAN_POINT ( 'NONE',  ( 135.0000000000000000, 17.00000000000000000, -114.9999999999999858 ) ) ;
#30315=DIRECTION ( 'NONE',  ( 0.000000000000000000, 0.000000000000000000, 1.000000000000000000 ) ) ;
#30319=DIRECTION ( 'NONE',  ( -1.000000000000000000, -0.000000000000000000, -0.000000000000000000 ) ) ;
#30324=CARTESIAN_POINT ( 'NONE',  ( 85.00000000000184741, 17.00000000000000000, 90.00000000000000000 ) ) ;
#30329=CARTESIAN_POINT ( 'NONE',  ( -69.99999999999816680, 17.00000000000000000, 65.00000000000000000 ) ) ;
#30340=VECTOR ( 'NONE', #49226, 1000.000000000000000 ) ;
#30353=ORIENTED_EDGE ( 'NONE', *, *, #23968, .T. ) ;
#30355=EDGE_CURVE ( 'NONE', #23599, #14979, #14279, .T. ) ;
#30360=CARTESIAN_POINT ( 'NONE',  ( -120.0000000000000426, 17.00000000000000000, -114.9999999999999858 ) ) ;
#30365=LINE ( 'NONE', #26266, #7492 ) ;
#30380=VECTOR ( 'NONE', #10356, 1000.000000000000000 ) ;
#30383=EDGE_LOOP ( 'NONE', ( #22399, #47713, #14222, #7031 ) ) ;
#30385=VECTOR ( 'NONE', #38027, 1000.000000000000000 ) ;
#30393=ORIENTED_EDGE ( 'NONE', *, *, #7309, .F. ) ;
#30394=CARTESIAN_POINT ( 'NONE',  ( -114.9999999999978542, 17.00000000000000000, 95.00000000000000000 ) ) ;
#30398=PLANE ( 'NONE',  #50094 ) ;
#30408=EDGE_CURVE ( 'NONE', #20578, #21162, #48633, .T. ) ;
#30410=EDGE_LOOP ( 'NONE', ( #47611, #21260, #14409, #46083 ) ) ;
#30423=ORIENTED_EDGE ( 'NONE', *, *, #41643, .F. ) ;
#30439=LINE ( 'NONE', #39169, #33648 ) ;
#30465=CARTESIAN_POINT ( 'NONE',  ( -114.9999999999994031, 17.00000000000000000, -54.99999999999999289 ) ) ;
#30466=CARTESIAN_POINT ( 'NONE',  ( 85.00000000000029843, 16.00000000000000000, -84.99999999999998579 ) ) ;
#30467=ORIENTED_EDGE ( 'NONE', *, *, #17628, .T. ) ;
#30471=PLANE ( 'NONE',  #15013 ) ;
#30481=PLANE ( 'NONE',  #13077 ) ;
#30485=FACE_OUTER_BOUND ( 'NONE', #12952, .T. ) ;
#30486=ORIENTED_EDGE ( 'NONE', *, *, #29139, .F. ) ;
#30491=DIRECTION ( 'NONE',  ( 1.000000000000000000, 0.000000000000000000, 0.000000000000000000 ) ) ;
#30498=LINE ( 'NONE', #30005, #40167 ) ;
#30499=VECTOR ( 'NONE', #4183, 1000.000000000000000 ) ;
#30515=ORIENTED_EDGE ( 'NONE', *, *, #27734, .T. ) ;
#30530=ADVANCED_FACE ( 'NONE', ( #15811 ), #46814, .F. ) ;
#30533=EDGE_CURVE ( 'NONE', #34291, #9471, #30712, .T. ) ;
#30535=VERTEX_POINT ( 'NONE', #3481 ) ;
#30546=LINE ( 'NONE', #6941, #40959 ) ;
#30549=ORIENTED_EDGE ( 'NONE', *, *, #9629, .F. ) ;
#30552=AXIS2_PLACEMENT_3D ( 'NONE', #35660, #19973, #20474 ) ;
#30557=VECTOR ( 'NONE', #40760, 1000.000000000000000 ) ;
#30558=LINE ( 'NONE', #15919, #19003 ) ;
#30568=VERTEX_POINT ( 'NONE', #22986 ) ;
#30589=VERTEX_POINT ( 'NONE', #39181 ) ;
#30594=EDGE_CURVE ( 'NONE', #302, #30568, #174, .T. ) ;
#30601=ORIENTED_EDGE ( 'NONE', *, *, #11386, .F. ) ;
#30606=VECTOR ( 'NONE', #18562, 1000.000000000000000 ) ;
#30608=CARTESIAN_POINT ( 'NONE',  ( -114.9999999999991047, 16.00000000000000000, -24.99999999999999289 ) ) ;
#30614=EDGE_CURVE ( 'NONE', #20642, #49743, #12954, .T. ) ;
#30623=VECTOR ( 'NONE', #26699, 1000.000000000000000 ) ;
#30626=VERTEX_POINT ( 'NONE', #32491 ) ;
#30639=CARTESIAN_POINT ( 'NONE',  ( -64.99999999999815259, 17.00000000000000000, 90.00000000000000000 ) ) ;
#30641=EDGE_CURVE ( 'NONE', #25157, #5959, #19905, .T. ) ;
#30646=EDGE_CURVE ( 'NONE', #17811, #18412, #5270, .T. ) ;
#30656=ORIENTED_EDGE ( 'NONE', *, *, #5208, .T. ) ;
#30687=ORIENTED_EDGE ( 'NONE', *, *, #36525, .F. ) ;
#30702=DIRECTION ( 'NONE',  ( -3.469446951953611231E-16, -0.000000000000000000, -1.000000000000000000 ) ) ;
#30708=AXIS2_PLACEMENT_3D ( 'NONE', #15305, #22976, #7596 ) ;
#30709=EDGE_CURVE ( 'NONE', #7258, #21648, #45501, .T. ) ;
#30712=LINE ( 'NONE', #23520, #47297 ) ;
#30719=LINE ( 'NONE', #38421, #36356 ) ;
#30725=VERTEX_POINT ( 'NONE', #37856 ) ;
#30733=EDGE_LOOP ( 'NONE', ( #11438, #1293, #39023, #16820 ) ) ;
#30737=EDGE_CURVE ( 'NONE', #41895, #38277, #2675, .T. ) ;
#30741=ORIENTED_EDGE ( 'NONE', *, *, #30641, .F. ) ;
#30744=EDGE_CURVE ( 'NONE', #35238, #11684, #25038, .T. ) ;
#30748=DIRECTION ( 'NONE',  ( 1.000000000000000000, 0.000000000000000000, 0.000000000000000000 ) ) ;
#30752=LINE ( 'NONE', #39977, #11912 ) ;
#30759=ORIENTED_EDGE ( 'NONE', *, *, #26229, .F. ) ;
#30760=VECTOR ( 'NONE', #20243, 1000.000000000000000 ) ;
#30763=DIRECTION ( 'NONE',  ( -1.000000000000000000, -0.000000000000000000, -0.000000000000000000 ) ) ;
#30779=CARTESIAN_POINT ( 'NONE',  ( 35.00000000000091660, 16.00000000000000000, 0.000000000000000000 ) ) ;
#30783=CARTESIAN_POINT ( 'NONE',  ( 135.0000000000009663, 17.00000000000000000, 0.000000000000000000 ) ) ;
#30795=CARTESIAN_POINT ( 'NONE',  ( -119.9999999999997158, 16.00000000000000000, -84.99999999999998579 ) ) ;
#30799=ORIENTED_EDGE ( 'NONE', *, *, #33841, .F. ) ;
#30801=CARTESIAN_POINT ( 'NONE',  ( -19.99999999999783995, 17.00000000000000000, 95.00000000000000000 ) ) ;
#30806=EDGE_CURVE ( 'NONE', #25400, #27666, #6527, .T. ) ;
#30807=VECTOR ( 'NONE', #30238, 1000.000000000000000 ) ;
#30810=ORIENTED_EDGE ( 'NONE', *, *, #32807, .F. ) ;
#30821=LINE ( 'NONE', #22095, #4644 ) ;
#30830=DIRECTION ( 'NONE',  ( -0.000000000000000000, -0.000000000000000000, -1.000000000000000000 ) ) ;
#30838=EDGE_CURVE ( 'NONE', #27903, #48546, #1932, .T. ) ;
#30849=FACE_OUTER_BOUND ( 'NONE', #36786, .T. ) ;
#30854=ADVANCED_FACE ( 'NONE', ( #49330 ), #2186, .F. ) ;
#30856=DIRECTION ( 'NONE',  ( -0.000000000000000000, -1.000000000000000000, -0.000000000000000000 ) ) ;
#30859=EDGE_CURVE ( 'NONE', #16290, #39670, #19593, .T. ) ;
#30866=LINE ( 'NONE', #14686, #3619 ) ;
#30871=ADVANCED_FACE ( 'NONE', ( #10884 ), #26796, .F. ) ;
#30876=ORIENTED_EDGE ( 'NONE', *, *, #24387, .F. ) ;
#30884=ORIENTED_EDGE ( 'NONE', *, *, #2044, .T. ) ;
#30892=CARTESIAN_POINT ( 'NONE',  ( 30.00000000000218492, 17.00000000000000000, 115.0000000000000142 ) ) ;
#30897=CARTESIAN_POINT ( 'NONE',  ( -69.99999999999847944, 16.00000000000000000, 35.00000000000000000 ) ) ;
#30903=ORIENTED_EDGE ( 'NONE', *, *, #9883, .F. ) ;
#30909=DIRECTION ( 'NONE',  ( 1.000000000000000000, 0.000000000000000000, 0.000000000000000000 ) ) ;
#30920=ORIENTED_EDGE ( 'NONE', *, *, #49745, .T. ) ;
#30926=ADVANCED_FACE ( 'NONE', ( #27812 ), #39374, .F. ) ;
#30933=DIRECTION ( 'NONE',  ( 1.000000000000000000, 0.000000000000000000, -0.000000000000000000 ) ) ;
#30939=EDGE_CURVE ( 'NONE', #46399, #38860, #31924, .T. ) ;
#30947=VECTOR ( 'NONE', #32231, 1000.000000000000000 ) ;
#30949=ORIENTED_EDGE ( 'NONE', *, *, #27379, .F. ) ;
#30953=ORIENTED_EDGE ( 'NONE', *, *, #42907, .T. ) ;
#30959=EDGE_CURVE ( 'NONE', #22969, #27078, #871, .T. ) ;
#30968=VERTEX_POINT ( 'NONE', #32168 ) ;
#30969=DIRECTION ( 'NONE',  ( 1.000000000000000000, 0.000000000000000000, -0.000000000000000000 ) ) ;
#30975=VERTEX_POINT ( 'NONE', #35525 ) ;
#30976=EDGE_CURVE ( 'NONE', #31422, #31585, #47763, .T. ) ;
#30979=FACE_OUTER_BOUND ( 'NONE', #17623, .T. ) ;
#30982=VECTOR ( 'NONE', #42002, 1000.000000000000000 ) ;
#30990=EDGE_CURVE ( 'NONE', #34175, #5984, #32422, .T. ) ;
#30995=CARTESIAN_POINT ( 'NONE',  ( -19.99999999999971223, 17.00000000000000000, -84.99999999999998579 ) ) ;
#31010=CARTESIAN_POINT ( 'NONE',  ( 35.00000000000152767, 17.00000000000000000, 35.00000000000000000 ) ) ;
#31019=ORIENTED_EDGE ( 'NONE', *, *, #39589, .F. ) ;
#31020=VERTEX_POINT ( 'NONE', #22122 ) ;
#31022=FACE_OUTER_BOUND ( 'NONE', #25877, .T. ) ;
#31032=CARTESIAN_POINT ( 'NONE',  ( -114.9999999999984652, 17.00000000000000000, 60.00000000000000000 ) ) ;
#31035=ORIENTED_EDGE ( 'NONE', *, *, #15969, .T. ) ;
#31048=CARTESIAN_POINT ( 'NONE',  ( 80.00000000000092371, 17.00000000000000000, 0.000000000000000000 ) ) ;
#31057=ADVANCED_FACE ( 'NONE', ( #37792 ), #2607, .F. ) ;
#31088=EDGE_CURVE ( 'NONE', #47244, #3216, #41116, .T. ) ;
#31099=DIRECTION ( 'NONE',  ( 0.000000000000000000, -0.000000000000000000, -1.000000000000000000 ) ) ;
#31107=CARTESIAN_POINT ( 'NONE',  ( -119.9999999999990905, 17.00000000000000000, -24.99999999999999289 ) ) ;
#31108=CARTESIAN_POINT ( 'NONE',  ( 79.99999999999995737, 16.00000000000000000, -114.9999999999999858 ) ) ;
#31117=CARTESIAN_POINT ( 'NONE',  ( 80.00000000000092371, 16.00000000000000000, -24.99999999999999289 ) ) ;
#31135=DIRECTION ( 'NONE',  ( -0.000000000000000000, -1.000000000000000000, -0.000000000000000000 ) ) ;
#31146=ORIENTED_EDGE ( 'NONE', *, *, #2256, .T. ) ;
#31149=DIRECTION ( 'NONE',  ( -0.000000000000000000, -0.000000000000000000, -1.000000000000000000 ) ) ;
#31157=VECTOR ( 'NONE', #41135, 1000.000000000000000 ) ;
#31177=EDGE_CURVE ( 'NONE', #31585, #46422, #18253, .T. ) ;
#31180=ORIENTED_EDGE ( 'NONE', *, *, #1775, .F. ) ;
#31208=CARTESIAN_POINT ( 'NONE',  ( -164.9999999999981526, 17.00000000000000000, 90.00000000000000000 ) ) ;
#31225=LINE ( 'NONE', #175, #44951 ) ;
#31234=VECTOR ( 'NONE', #33717, 1000.000000000000000 ) ;
#31239=VECTOR ( 'NONE', #22203, 1000.000000000000000 ) ;
#31254=VERTEX_POINT ( 'NONE', #38553 ) ;
#31262=LINE ( 'NONE', #46853, #12855 ) ;
#31273=ORIENTED_EDGE ( 'NONE', *, *, #35548, .F. ) ;
#31274=VERTEX_POINT ( 'NONE', #9183 ) ;
#31295=EDGE_CURVE ( 'NONE', #48700, #15604, #35905, .T. ) ;
#31297=DIRECTION ( 'NONE',  ( 0.000000000000000000, 0.000000000000000000, 1.000000000000000000 ) ) ;
#31299=DIRECTION ( 'NONE',  ( 1.000000000000000000, 0.000000000000000000, -0.000000000000000000 ) ) ;
#31308=ORIENTED_EDGE ( 'NONE', *, *, #40671, .F. ) ;
#31315=LINE ( 'NONE', #11802, #6804 ) ;
#31317=CARTESIAN_POINT ( 'NONE',  ( -19.99999999999940670, 16.00000000000000000, -54.99999999999999289 ) ) ;
#31324=CARTESIAN_POINT ( 'NONE',  ( -64.99999999999971578, 17.00000000000000000, -84.99999999999998579 ) ) ;
#31328=ADVANCED_FACE ( 'NONE', ( #13275 ), #20476, .F. ) ;
#31336=AXIS2_PLACEMENT_3D ( 'NONE', #33866, #7161, #3041 ) ;
#31339=LINE ( 'NONE', #47682, #44758 ) ;
#31353=EDGE_CURVE ( 'NONE', #8610, #24878, #12783, .T. ) ;
#31355=DIRECTION ( 'NONE',  ( 0.000000000000000000, 0.000000000000000000, -1.000000000000000000 ) ) ;
#31356=DIRECTION ( 'NONE',  ( 0.000000000000000000, 0.000000000000000000, -1.000000000000000000 ) ) ;
#31399=DIRECTION ( 'NONE',  ( 0.000000000000000000, -1.000000000000000000, 0.000000000000000000 ) ) ;
#31400=PLANE ( 'NONE',  #23474 ) ;
#31401=CARTESIAN_POINT ( 'NONE',  ( -14.99999999999782041, 17.00000000000000000, 115.0000000000000142 ) ) ;
#31408=VECTOR ( 'NONE', #8444, 1000.000000000000000 ) ;
#31413=LINE ( 'NONE', #28814, #5346 ) ;
#31422=VERTEX_POINT ( 'NONE', #34308 ) ;
#31426=CARTESIAN_POINT ( 'NONE',  ( -164.9999999999987779, 17.00000000000000000, 5.000000000000004441 ) ) ;
#31432=DIRECTION ( 'NONE',  ( -1.000000000000000000, -0.000000000000000000, -0.000000000000000000 ) ) ;
#31443=FACE_OUTER_BOUND ( 'NONE', #25531, .T. ) ;
#31448=FACE_OUTER_BOUND ( 'NONE', #48192, .T. ) ;
#31455=EDGE_LOOP ( 'NONE', ( #19872, #49894, #41712, #25481 ) ) ;
#31472=DIRECTION ( 'NONE',  ( 0.000000000000000000, -0.000000000000000000, -1.000000000000000000 ) ) ;
#31477=LINE ( 'NONE', #35848, #6059 ) ;
#31480=AXIS2_PLACEMENT_3D ( 'NONE', #15628, #19980, #31299 ) ;
#31487=ADVANCED_FACE ( 'NONE', ( #6347 ), #21483, .F. ) ;
#31498=DIRECTION ( 'NONE',  ( 1.000000000000000000, 0.000000000000000000, 0.000000000000000000 ) ) ;
#31505=ORIENTED_EDGE ( 'NONE', *, *, #8771, .T. ) ;
#31512=LINE ( 'NONE', #47099, #31998 ) ;
#31520=AXIS2_PLACEMENT_3D ( 'NONE', #24709, #40355, #40844 ) ;
#31524=ORIENTED_EDGE ( 'NONE', *, *, #11922, .T. ) ;
#31533=ORIENTED_EDGE ( 'NONE', *, *, #43874, .F. ) ;
#31536=FACE_OUTER_BOUND ( 'NONE', #15465, .T. ) ;
#31544=DIRECTION ( 'NONE',  ( -1.000000000000000000, -0.000000000000000000, -0.000000000000000000 ) ) ;
#31550=EDGE_CURVE ( 'NONE', #15399, #4762, #15326, .T. ) ;
#31551=CARTESIAN_POINT ( 'NONE',  ( -14.99999999999906919, 17.00000000000000000, 0.000000000000000000 ) ) ;
#31561=CARTESIAN_POINT ( 'NONE',  ( 0.000000000000000000, 17.00000000000000000, 0.000000000000000000 ) ) ;
#31562=EDGE_CURVE ( 'NONE', #42175, #17726, #15817, .T. ) ;
#31567=ADVANCED_FACE ( 'NONE', ( #30979 ), #35596, .F. ) ;
#31568=EDGE_LOOP ( 'NONE', ( #22747, #44928, #12184, #25856 ) ) ;
#31575=AXIS2_PLACEMENT_3D ( 'NONE', #33077, #33328, #25619 ) ;
#31581=VERTEX_POINT ( 'NONE', #39188 ) ;
#31585=VERTEX_POINT ( 'NONE', #23251 ) ;
#31590=EDGE_LOOP ( 'NONE', ( #1970, #18468, #12767, #4843 ) ) ;
#31594=VECTOR ( 'NONE', #28433, 1000.000000000000000 ) ;
#31595=ORIENTED_EDGE ( 'NONE', *, *, #12489, .F. ) ;
#31603=LINE ( 'NONE', #46932, #9383 ) ;
#31611=EDGE_LOOP ( 'NONE', ( #31878, #14438, #3720, #36394 ) ) ;
#31615=PLANE ( 'NONE',  #15193 ) ;
#31620=LINE ( 'NONE', #47208, #42735 ) ;
#31629=VECTOR ( 'NONE', #12894, 1000.000000000000000 ) ;
#31639=CARTESIAN_POINT ( 'NONE',  ( -175.0000000000000000, 15.00000000000000000, 122.5000000000000142 ) ) ;
#31647=ADVANCED_FACE ( 'NONE', ( #50148 ), #28387, .F. ) ;
#31649=ORIENTED_EDGE ( 'NONE', *, *, #6691, .F. ) ;
#31650=CARTESIAN_POINT ( 'NONE',  ( 130.0000000000012221, 17.00000000000000000, 5.000000000000004441 ) ) ;
#31654=ORIENTED_EDGE ( 'NONE', *, *, #20040, .T. ) ;
#31666=ORIENTED_EDGE ( 'NONE', *, *, #10300, .F. ) ;
#31669=VERTEX_POINT ( 'NONE', #20932 ) ;
#31674=PLANE ( 'NONE',  #40381 ) ;
#31676=AXIS2_PLACEMENT_3D ( 'NONE', #4114, #11820, #27213 ) ;
#31678=VERTEX_POINT ( 'NONE', #1195 ) ;
#31684=ORIENTED_EDGE ( 'NONE', *, *, #32789, .F. ) ;
#31686=PLANE ( 'NONE',  #12179 ) ;
#31687=CARTESIAN_POINT ( 'NONE',  ( 30.00000000000092726, 16.00000000000000000, -24.99999999999999289 ) ) ;
#31691=VECTOR ( 'NONE', #43618, 1000.000000000000000 ) ;
#31694=ORIENTED_EDGE ( 'NONE', *, *, #2118, .F. ) ;
#31703=PLANE ( 'NONE',  #50361 ) ;
#31706=ORIENTED_EDGE ( 'NONE', *, *, #24934, .F. ) ;
#31714=CARTESIAN_POINT ( 'NONE',  ( -64.99999999999909051, 17.00000000000000000, -24.99999999999999289 ) ) ;
#31717=ORIENTED_EDGE ( 'NONE', *, *, #27062, .F. ) ;
#31721=DIRECTION ( 'NONE',  ( 0.000000000000000000, 0.000000000000000000, 1.000000000000000000 ) ) ;
#31724=AXIS2_PLACEMENT_3D ( 'NONE', #3529, #45611, #50183 ) ;
#31725=DIRECTION ( 'NONE',  ( 1.000000000000000000, 0.000000000000000000, 0.000000000000000000 ) ) ;
#31744=DIRECTION ( 'NONE',  ( -1.000000000000000000, 0.000000000000000000, 0.000000000000000000 ) ) ;
#31751=CARTESIAN_POINT ( 'NONE',  ( 30.00000000000123279, 16.00000000000000000, 5.000000000000004441 ) ) ;
#31755=PLANE ( 'NONE',  #867 ) ;
#31779=VERTEX_POINT ( 'NONE', #17080 ) ;
#31782=PLANE ( 'NONE',  #36114 ) ;
#31783=EDGE_CURVE ( 'NONE', #37447, #4392, #20168, .T. ) ;
#31785=DIRECTION ( 'NONE',  ( -1.000000000000000000, 0.000000000000000000, 0.000000000000000000 ) ) ;
#31790=FACE_OUTER_BOUND ( 'NONE', #15218, .T. ) ;
#31794=CARTESIAN_POINT ( 'NONE',  ( -164.9999999999990905, 17.00000000000000000, 0.000000000000000000 ) ) ;
#31795=LINE ( 'NONE', #47378, #2792 ) ;
#31802=ADVANCED_FACE ( 'NONE', ( #49588, #41177 ), #22197, .F. ) ;
#31813=CARTESIAN_POINT ( 'NONE',  ( 30.00000000000029132, 17.00000000000000000, -84.99999999999998579 ) ) ;
#31824=ORIENTED_EDGE ( 'NONE', *, *, #48842, .T. ) ;
#31828=ORIENTED_EDGE ( 'NONE', *, *, #47784, .F. ) ;
#31831=ORIENTED_EDGE ( 'NONE', *, *, #9797, .F. ) ;
#31832=PLANE ( 'NONE',  #24606 ) ;
#31838=DIRECTION ( 'NONE',  ( 0.000000000000000000, -1.000000000000000000, 0.000000000000000000 ) ) ;
#31839=ORIENTED_EDGE ( 'NONE', *, *, #33450, .T. ) ;
#31853=LINE ( 'NONE', #1305, #48216 ) ;
#31858=ORIENTED_EDGE ( 'NONE', *, *, #50432, .T. ) ;
#31878=ORIENTED_EDGE ( 'NONE', *, *, #35781, .T. ) ;
#31882=LINE ( 'NONE', #41514, #9940 ) ;
#31885=ADVANCED_FACE ( 'NONE', ( #42688 ), #7561, .F. ) ;
#31888=DIRECTION ( 'NONE',  ( -1.000000000000000000, 0.000000000000000000, 4.625929269271584521E-16 ) ) ;
#31895=CARTESIAN_POINT ( 'NONE',  ( -119.9999999999978400, 17.00000000000000000, 95.00000000000000000 ) ) ;
#31896=AXIS2_PLACEMENT_3D ( 'NONE', #4270, #39680, #39935 ) ;
#31901=EDGE_LOOP ( 'NONE', ( #19753, #6822, #30040, #34706 ) ) ;
#31904=AXIS2_PLACEMENT_3D ( 'NONE', #16424, #39537, #30 ) ;
#31906=ADVANCED_FACE ( 'NONE', ( #3955 ), #18829, .F. ) ;
#31923=CARTESIAN_POINT ( 'NONE',  ( 0.000000000000000000, 0.000000000000000000, 0.000000000000000000 ) ) ;
#31924=LINE ( 'NONE', #39618, #32593 ) ;
#31926=EDGE_CURVE ( 'NONE', #14555, #47244, #50351, .T. ) ;
#31927=ADVANCED_FACE ( 'NONE', ( #39132 ), #11919, .F. ) ;
#31935=PLANE ( 'NONE',  #26088 ) ;
#31937=EDGE_CURVE ( 'NONE', #12984, #17110, #7822, .T. ) ;
#31946=VERTEX_POINT ( 'NONE', #50089 ) ;
#31947=VECTOR ( 'NONE', #389, 1000.000000000000000 ) ;
#31951=VERTEX_POINT ( 'NONE', #42943 ) ;
#31955=ORIENTED_EDGE ( 'NONE', *, *, #34223, .F. ) ;
#31978=DIRECTION ( 'NONE',  ( 1.000000000000000000, 0.000000000000000000, 0.000000000000000000 ) ) ;
#31989=CARTESIAN_POINT ( 'NONE',  ( 85.00000000000184741, 17.00000000000000000, 65.00000000000000000 ) ) ;
#31998=VECTOR ( 'NONE', #16102, 1000.000000000000000 ) ;
#32000=AXIS2_PLACEMENT_3D ( 'NONE', #49790, #42643, #23150 ) ;
#32013=ORIENTED_EDGE ( 'NONE', *, *, #24672, .T. ) ;
#32019=VERTEX_POINT ( 'NONE', #43956 ) ;
#32020=FACE_OUTER_BOUND ( 'NONE', #14110, .T. ) ;
#32025=DIRECTION ( 'NONE',  ( -1.000000000000000000, -0.000000000000000000, -0.000000000000000000 ) ) ;
#32032=ORIENTED_EDGE ( 'NONE', *, *, #49021, .F. ) ;
#32040=DIRECTION ( 'NONE',  ( 0.000000000000000000, -1.000000000000000000, 0.000000000000000000 ) ) ;
#32041=VECTOR ( 'NONE', #12675, 1000.000000000000000 ) ;
#32046=CARTESIAN_POINT ( 'NONE',  ( 85.00000000000213163, 17.00000000000000000, 95.00000000000000000 ) ) ;
#32047=CARTESIAN_POINT ( 'NONE',  ( -64.99999999999909051, 17.00000000000000000, -24.99999999999999289 ) ) ;
#32051=LINE ( 'NONE', #997, #35593 ) ;
#32056=DIRECTION ( 'NONE',  ( 1.000000000000000000, 0.000000000000000000, 0.000000000000000000 ) ) ;
#32067=ORIENTED_EDGE ( 'NONE', *, *, #3297, .T. ) ;
#32071=CARTESIAN_POINT ( 'NONE',  ( -14.99999999999812594, 17.00000000000000000, 90.00000000000000000 ) ) ;
#32073=EDGE_LOOP ( 'NONE', ( #47583, #16653, #22939, #13112 ) ) ;
#32076=VECTOR ( 'NONE', #26359, 1000.000000000000000 ) ;
#32077=LINE ( 'NONE', #27966, #346 ) ;
#32084=LINE ( 'NONE', #3863, #39260 ) ;
#32085=ORIENTED_EDGE ( 'NONE', *, *, #33841, .T. ) ;
#32099=ORIENTED_EDGE ( 'NONE', *, *, #12346, .T. ) ;
#32100=PRODUCT_CONTEXT ( 'NONE', #23656, 'mechanical' ) ;
#32104=AXIS2_PLACEMENT_3D ( 'NONE', #23195, #43955, #24227 ) ;
#32111=VECTOR ( 'NONE', #46076, 1000.000000000000000 ) ;
#32113=EDGE_CURVE ( 'NONE', #45606, #11106, #12168, .T. ) ;
#32115=ADVANCED_FACE ( 'NONE', ( #8326 ), #31935, .F. ) ;
#32116=ORIENTED_EDGE ( 'NONE', *, *, #36979, .F. ) ;
#32118=ORIENTED_EDGE ( 'NONE', *, *, #36048, .T. ) ;
#32126=CARTESIAN_POINT ( 'NONE',  ( -164.9999999999997442, 16.00000000000000000, -60.00000000000000000 ) ) ;
#32134=ADVANCED_FACE ( 'NONE', ( #4962 ), #27820, .F. ) ;
#32137=ADVANCED_FACE ( 'NONE', ( #628 ), #12909, .F. ) ;
#32139=ADVANCED_FACE ( 'NONE', ( #43459 ), #31686, .F. ) ;
#32147=LINE ( 'NONE', #40103, #22099 ) ;
#32150=DIRECTION ( 'NONE',  ( 0.000000000000000000, 0.000000000000000000, 1.000000000000000000 ) ) ;
#32154=ORIENTED_EDGE ( 'NONE', *, *, #11449, .F. ) ;
#32168=CARTESIAN_POINT ( 'NONE',  ( 85.00000000000152056, 16.00000000000000000, 35.00000000000000000 ) ) ;
#32171=ADVANCED_FACE ( 'NONE', ( #16023 ), #49277, .F. ) ;
#32172=CARTESIAN_POINT ( 'NONE',  ( 29.99999999999998579, 17.00000000000000000, -114.9999999999999858 ) ) ;
#32184=VERTEX_POINT ( 'NONE', #29331 ) ;
#32189=VERTEX_POINT ( 'NONE', #14161 ) ;
#32192=EDGE_CURVE ( 'NONE', #23358, #40073, #30093, .T. ) ;
#32194=LINE ( 'NONE', #8839, #41403 ) ;
#32213=EDGE_CURVE ( 'NONE', #49071, #8841, #25738, .T. ) ;
#32217=AXIS2_PLACEMENT_3D ( 'NONE', #43075, #21181, #5530 ) ;
#32225=ORIENTED_EDGE ( 'NONE', *, *, #8457, .F. ) ;
#32231=DIRECTION ( 'NONE',  ( -0.000000000000000000, -1.000000000000000000, -0.000000000000000000 ) ) ;
#32235=ORIENTED_EDGE ( 'NONE', *, *, #33450, .F. ) ;
#32251=ORIENTED_EDGE ( 'NONE', *, *, #2005, .F. ) ;
#32266=DIRECTION ( 'NONE',  ( -1.000000000000000000, -0.000000000000000000, -0.000000000000000000 ) ) ;
#32270=ADVANCED_FACE ( 'NONE', ( #6237 ), #48525, .F. ) ;
#32278=LINE ( 'NONE', #12760, #43934 ) ;
#32279=ORIENTED_EDGE ( 'NONE', *, *, #6126, .T. ) ;
#32282=AXIS2_PLACEMENT_3D ( 'NONE', #12362, #4173, #46975 ) ;
#32286=DIRECTION ( 'NONE',  ( -0.000000000000000000, -1.000000000000000000, -0.000000000000000000 ) ) ;
#32288=VECTOR ( 'NONE', #11016, 1000.000000000000000 ) ;
#32289=EDGE_CURVE ( 'NONE', #43380, #20901, #57, .T. ) ;
#32291=VERTEX_POINT ( 'NONE', #34972 ) ;
#32299=PLANE ( 'NONE',  #13540 ) ;
#32305=CARTESIAN_POINT ( 'NONE',  ( -114.9999999999987779, 16.00000000000000000, 5.000000000000004441 ) ) ;
#32311=LINE ( 'NONE', #40507, #1710 ) ;
#32314=DIRECTION ( 'NONE',  ( 0.000000000000000000, 0.000000000000000000, 1.000000000000000000 ) ) ;
#32318=DIRECTION ( 'NONE',  ( -0.000000000000000000, -1.000000000000000000, -0.000000000000000000 ) ) ;
#32321=ORIENTED_EDGE ( 'NONE', *, *, #32740, .T. ) ;
#32325=AXIS2_PLACEMENT_3D ( 'NONE', #29244, #16948, #32602 ) ;
#32342=ORIENTED_EDGE ( 'NONE', *, *, #36928, .T. ) ;
#32343=DIRECTION ( 'NONE',  ( 1.000000000000000000, 0.000000000000000000, 0.000000000000000000 ) ) ;
#32344=EDGE_CURVE ( 'NONE', #574, #36127, #41879, .T. ) ;
#32345=CARTESIAN_POINT ( 'NONE',  ( -175.0000000000000000, 0.000000000000000000, 122.5000000000000142 ) ) ;
#32347=DIRECTION ( 'NONE',  ( 0.000000000000000000, 0.000000000000000000, -1.000000000000000000 ) ) ;
#32351=FACE_OUTER_BOUND ( 'NONE', #15963, .T. ) ;
#32361=CARTESIAN_POINT ( 'NONE',  ( 35.00000000000186162, 17.00000000000000000, 90.00000000000000000 ) ) ;
#32368=ORIENTED_EDGE ( 'NONE', *, *, #11414, .T. ) ;
#32369=VECTOR ( 'NONE', #34583, 1000.000000000000000 ) ;
#32372=LINE ( 'NONE', #4668, #24520 ) ;
#32375=CARTESIAN_POINT ( 'NONE',  ( -165.0000000000000284, 16.00000000000000000, 115.0000000000000142 ) ) ;
#32386=( GEOMETRIC_REPRESENTATION_CONTEXT ( 3 ) GLOBAL_UNCERTAINTY_ASSIGNED_CONTEXT ( ( #7519 ) ) GLOBAL_UNIT_ASSIGNED_CONTEXT ( ( #4712, #13158, #17010 ) ) REPRESENTATION_CONTEXT ( 'NONE', 'WORKASPACE' ) );
#32391=DIRECTION ( 'NONE',  ( 1.000000000000000000, 0.000000000000000000, 0.000000000000000000 ) ) ;
#32392=DIRECTION ( 'NONE',  ( -0.000000000000000000, -1.000000000000000000, -0.000000000000000000 ) ) ;
#32394=VERTEX_POINT ( 'NONE', #10827 ) ;
#32397=CARTESIAN_POINT ( 'NONE',  ( 85.00000000000056843, 17.00000000000000000, -30.00000000000000000 ) ) ;
#32398=EDGE_CURVE ( 'NONE', #40766, #25202, #15194, .T. ) ;
#32402=EDGE_CURVE ( 'NONE', #42338, #37393, #22375, .T. ) ;
#32413=VECTOR ( 'NONE', #13161, 1000.000000000000000 ) ;
#32421=AXIS2_PLACEMENT_3D ( 'NONE', #8821, #16520, #20355 ) ;
#32422=LINE ( 'NONE', #5708, #33440 ) ;
#32431=CARTESIAN_POINT ( 'NONE',  ( -15.00000000000001421, 17.00000000000000000, -114.9999999999999858 ) ) ;
#32435=AXIS2_PLACEMENT_3D ( 'NONE', #9128, #36095, #48582 ) ;
#32442=DIRECTION ( 'NONE',  ( 0.000000000000000000, 0.000000000000000000, 1.000000000000000000 ) ) ;
#32446=ORIENTED_EDGE ( 'NONE', *, *, #28628, .T. ) ;
#32449=PLANE ( 'NONE',  #42552 ) ;
#32454=ORIENTED_EDGE ( 'NONE', *, *, #21513, .T. ) ;
#32459=VECTOR ( 'NONE', #46096, 1000.000000000000000 ) ;
#32460=ADVANCED_FACE ( 'NONE', ( #47209 ), #4402, .F. ) ;
#32463=EDGE_LOOP ( 'NONE', ( #34093, #39013, #18805, #43731 ) ) ;
#32470=ORIENTED_EDGE ( 'NONE', *, *, #37870, .T. ) ;
#32472=ORIENTED_EDGE ( 'NONE', *, *, #43094, .F. ) ;
#32478=ORIENTED_EDGE ( 'NONE', *, *, #33461, .F. ) ;
#32491=CARTESIAN_POINT ( 'NONE',  ( 85.00000000000090949, 16.00000000000000000, 0.000000000000000000 ) ) ;
#32498=PLANE ( 'NONE',  #47940 ) ;
#32501=DIRECTION ( 'NONE',  ( 0.000000000000000000, 0.000000000000000000, 1.000000000000000000 ) ) ;
#32502=DIRECTION ( 'NONE',  ( 1.000000000000000000, 0.000000000000000000, 0.000000000000000000 ) ) ;
#32512=VECTOR ( 'NONE', #12369, 1000.000000000000000 ) ;
#32519=FACE_OUTER_BOUND ( 'NONE', #17494, .T. ) ;
#32522=VERTEX_POINT ( 'NONE', #29514 ) ;
#32529=CARTESIAN_POINT ( 'NONE',  ( 135.0000000000015632, 17.00000000000000000, 60.00000000000000000 ) ) ;
#32540=ORIENTED_EDGE ( 'NONE', *, *, #35680, .F. ) ;
#32541=VERTEX_POINT ( 'NONE', #22062 ) ;
#32553=PLANE ( 'NONE',  #3703 ) ;
#32556=LINE ( 'NONE', #4591, #19962 ) ;
#32585=ORIENTED_EDGE ( 'NONE', *, *, #48382, .T. ) ;
#32586=DIRECTION ( 'NONE',  ( -1.000000000000000000, 0.000000000000000000, 0.000000000000000000 ) ) ;
#32590=ORIENTED_EDGE ( 'NONE', *, *, #48842, .F. ) ;
#32593=VECTOR ( 'NONE', #44193, 1000.000000000000000 ) ;
#32596=ORIENTED_EDGE ( 'NONE', *, *, #48462, .F. ) ;
#32602=DIRECTION ( 'NONE',  ( 0.000000000000000000, -0.000000000000000000, -1.000000000000000000 ) ) ;
#32605=ORIENTED_EDGE ( 'NONE', *, *, #26806, .F. ) ;
#32607=CARTESIAN_POINT ( 'NONE',  ( -14.99999999999876366, 17.00000000000000000, 5.000000000000004441 ) ) ;
#32608=DIRECTION ( 'NONE',  ( -1.000000000000000000, -0.000000000000000000, -0.000000000000000000 ) ) ;
#32618=DIRECTION ( 'NONE',  ( -1.000000000000000000, -0.000000000000000000, -0.000000000000000000 ) ) ;
#32623=LINE ( 'NONE', #6418, #10878 ) ;
#32627=VERTEX_POINT ( 'NONE', #7689 ) ;
#32632=CARTESIAN_POINT ( 'NONE',  ( 135.0000000000021600, 17.00000000000000000, 95.00000000000000000 ) ) ;
#32651=LINE ( 'NONE', #44422, #39126 ) ;
#32652=EDGE_CURVE ( 'NONE', #38860, #46422, #41814, .T. ) ;
#32657=AXIS2_PLACEMENT_3D ( 'NONE', #38619, #3175, #35282 ) ;
#32661=PLANE ( 'NONE',  #28354 ) ;
#32666=ORIENTED_EDGE ( 'NONE', *, *, #7997, .T. ) ;
#32670=DIRECTION ( 'NONE',  ( 0.000000000000000000, 0.000000000000000000, 1.000000000000000000 ) ) ;
#32687=VECTOR ( 'NONE', #7239, 1000.000000000000000 ) ;
#32692=VECTOR ( 'NONE', #24885, 1000.000000000000000 ) ;
#32694=ADVANCED_FACE ( 'NONE', ( #19472 ), #14366, .F. ) ;
#32695=ORIENTED_EDGE ( 'NONE', *, *, #39751, .T. ) ;
#32698=DIRECTION ( 'NONE',  ( 1.000000000000000000, 0.000000000000000000, 0.000000000000000000 ) ) ;
#32712=EDGE_CURVE ( 'NONE', #18412, #22853, #26415, .T. ) ;
#32717=ORIENTED_EDGE ( 'NONE', *, *, #19692, .F. ) ;
#32726=FACE_OUTER_BOUND ( 'NONE', #12368, .T. ) ;
#32740=EDGE_CURVE ( 'NONE', #45593, #2472, #16388, .T. ) ;
#32741=EDGE_CURVE ( 'NONE', #15045, #43660, #43079, .T. ) ;
#32749=ORIENTED_EDGE ( 'NONE', *, *, #35320, .T. ) ;
#32753=LINE ( 'NONE', #21439, #41231 ) ;
#32778=VECTOR ( 'NONE', #39273, 1000.000000000000000 ) ;
#32779=ADVANCED_FACE ( 'NONE', ( #16145 ), #27945, .F. ) ;
#32781=EDGE_CURVE ( 'NONE', #574, #4352, #4091, .T. ) ;
#32785=ORIENTED_EDGE ( 'NONE', *, *, #25555, .F. ) ;
#32789=EDGE_CURVE ( 'NONE', #405, #33858, #20489, .T. ) ;
#32799=CARTESIAN_POINT ( 'NONE',  ( 0.000000000000000000, 17.00000000000000000, 0.000000000000000000 ) ) ;
#32806=VECTOR ( 'NONE', #5915, 1000.000000000000000 ) ;
#32807=EDGE_CURVE ( 'NONE', #37393, #40932, #46892, .T. ) ;
#32816=CARTESIAN_POINT ( 'NONE',  ( -165.0000000000000284, 16.00000000000000000, -90.00000000000000000 ) ) ;
#32819=AXIS2_PLACEMENT_3D ( 'NONE', #33090, #45341, #10229 ) ;
#32820=ORIENTED_EDGE ( 'NONE', *, *, #43493, .T. ) ;
#32821=CARTESIAN_POINT ( 'NONE',  ( -164.9999999999994031, 17.00000000000000000, -54.99999999999999289 ) ) ;
#32824=ORIENTED_EDGE ( 'NONE', *, *, #46529, .F. ) ;
#32838=ORIENTED_EDGE ( 'NONE', *, *, #3052, .F. ) ;
#32839=FACE_OUTER_BOUND ( 'NONE', #23904, .T. ) ;
#32847=AXIS2_PLACEMENT_3D ( 'NONE', #38754, #3576, #23856 ) ;
#32856=EDGE_CURVE ( 'NONE', #7083, #26946, #34009, .T. ) ;
#32857=LINE ( 'NONE', #48437, #20946 ) ;
#32866=CARTESIAN_POINT ( 'NONE',  ( 80.00000000000122213, 17.00000000000000000, 30.00000000000000000 ) ) ;
#32870=ORIENTED_EDGE ( 'NONE', *, *, #37397, .F. ) ;
#32888=PLANE ( 'NONE',  #18847 ) ;
#32903=ORIENTED_EDGE ( 'NONE', *, *, #28660, .T. ) ;
#32920=EDGE_CURVE ( 'NONE', #7457, #48700, #36420, .T. ) ;
#32925=ORIENTED_EDGE ( 'NONE', *, *, #23807, .F. ) ;
#32929=CARTESIAN_POINT ( 'NONE',  ( -119.9999999999987921, 17.00000000000000000, 5.000000000000004441 ) ) ;
#32930=DIRECTION ( 'NONE',  ( 0.000000000000000000, 0.000000000000000000, 1.000000000000000000 ) ) ;
#32931=CARTESIAN_POINT ( 'NONE',  ( 80.00000000000186162, 17.00000000000000000, 90.00000000000000000 ) ) ;
#32939=CARTESIAN_POINT ( 'NONE',  ( -114.9999999999984652, 16.00000000000000000, 35.00000000000000000 ) ) ;
#32945=CARTESIAN_POINT ( 'NONE',  ( -19.99999999999783995, 16.00000000000000000, 95.00000000000000000 ) ) ;
#32950=EDGE_LOOP ( 'NONE', ( #36326, #13459, #30876, #28472 ) ) ;
#32952=ORIENTED_EDGE ( 'NONE', *, *, #4484, .T. ) ;
#32953=CARTESIAN_POINT ( 'NONE',  ( 135.0000000000012790, 16.00000000000000000, 5.000000000000004441 ) ) ;
#32960=VECTOR ( 'NONE', #28760, 1000.000000000000000 ) ;
#32966=ORIENTED_EDGE ( 'NONE', *, *, #23470, .F. ) ;
#32969=VERTEX_POINT ( 'NONE', #32816 ) ;
#32976=VERTEX_POINT ( 'NONE', #41694 ) ;
#32983=EDGE_CURVE ( 'NONE', #1474, #40766, #6546, .T. ) ;
#32985=VECTOR ( 'NONE', #22423, 1000.000000000000000 ) ;
#32995=CARTESIAN_POINT ( 'NONE',  ( 164.9999999999999716, 17.00000000000000000, 34.99999999999999289 ) ) ;
#32996=DIRECTION ( 'NONE',  ( 0.000000000000000000, 0.000000000000000000, -1.000000000000000000 ) ) ;
#33005=CARTESIAN_POINT ( 'NONE',  ( -164.9999999999981526, 17.00000000000000000, 90.00000000000000000 ) ) ;
#33026=LINE ( 'NONE', #13501, #43759 ) ;
#33042=EDGE_CURVE ( 'NONE', #15322, #27386, #16027, .T. ) ;
#33045=EDGE_CURVE ( 'NONE', #50559, #35762, #38623, .T. ) ;
#33051=CARTESIAN_POINT ( 'NONE',  ( -64.99999999999940314, 17.00000000000000000, -54.99999999999999289 ) ) ;
#33053=EDGE_CURVE ( 'NONE', #14054, #24991, #3442, .T. ) ;
#33058=VECTOR ( 'NONE', #19981, 1000.000000000000000 ) ;
#33071=ADVANCED_FACE ( 'NONE', ( #42691 ), #46515, .F. ) ;
#33077=CARTESIAN_POINT ( 'NONE',  ( -69.99999999999783995, 17.00000000000000000, 95.00000000000000000 ) ) ;
#33090=CARTESIAN_POINT ( 'NONE',  ( -64.99999999999909051, 17.00000000000000000, 0.000000000000000000 ) ) ;
#33102=VERTEX_POINT ( 'NONE', #43710 ) ;
#33142=VERTEX_POINT ( 'NONE', #36301 ) ;
#33148=ADVANCED_FACE ( 'NONE', ( #9082 ), #35806, .F. ) ;
#33150=VERTEX_POINT ( 'NONE', #9333 ) ;
#33154=EDGE_LOOP ( 'NONE', ( #3940, #6194, #37824, #8039 ) ) ;
#33155=DIRECTION ( 'NONE',  ( -0.000000000000000000, -0.000000000000000000, -1.000000000000000000 ) ) ;
#33163=EDGE_LOOP ( 'NONE', ( #23747, #12251, #5670, #31035 ) ) ;
#33170=DIRECTION ( 'NONE',  ( 0.000000000000000000, 0.000000000000000000, -1.000000000000000000 ) ) ;
#33175=PLANE ( 'NONE',  #31520 ) ;
#33177=ORIENTED_EDGE ( 'NONE', *, *, #45262, .F. ) ;
#33187=CARTESIAN_POINT ( 'NONE',  ( -19.99999999999783995, 17.00000000000000000, 95.00000000000000000 ) ) ;
#33193=AXIS2_PLACEMENT_3D ( 'NONE', #47460, #16206, #31099 ) ;
#33205=ORIENTED_EDGE ( 'NONE', *, *, #34690, .T. ) ;
#33206=LINE ( 'NONE', #36558, #27044 ) ;
#33207=LINE ( 'NONE', #17286, #24187 ) ;
#33210=ADVANCED_BREP_SHAPE_REPRESENTATION ( '', ( #39479, #45486 ), #32386 ) ;
#33213=ORIENTED_EDGE ( 'NONE', *, *, #37053, .T. ) ;
#33215=CARTESIAN_POINT ( 'NONE',  ( -64.99999999999846523, 17.00000000000000000, 60.00000000000000000 ) ) ;
#33219=ORIENTED_EDGE ( 'NONE', *, *, #6466, .F. ) ;
#33223=AXIS2_PLACEMENT_3D ( 'NONE', #6314, #40708, #2210 ) ;
#33244=ORIENTED_EDGE ( 'NONE', *, *, #43065, .T. ) ;
#33245=EDGE_CURVE ( 'NONE', #26648, #25407, #33945, .T. ) ;
#33251=CARTESIAN_POINT ( 'NONE',  ( 85.00000000000056843, 17.00000000000000000, -54.99999999999999289 ) ) ;
#33254=VERTEX_POINT ( 'NONE', #13678 ) ;
#33255=FACE_OUTER_BOUND ( 'NONE', #7687, .T. ) ;
#33258=CARTESIAN_POINT ( 'NONE',  ( -14.99999999999937472, 17.00000000000000000, -54.99999999999999289 ) ) ;
#33264=DIRECTION ( 'NONE',  ( -0.000000000000000000, -0.000000000000000000, -1.000000000000000000 ) ) ;
#33269=VECTOR ( 'NONE', #26646, 1000.000000000000000 ) ;
#33274=DIRECTION ( 'NONE',  ( -1.000000000000000000, -0.000000000000000000, -0.000000000000000000 ) ) ;
#33283=EDGE_LOOP ( 'NONE', ( #49815, #27689, #11346, #9562 ) ) ;
#33285=LINE ( 'NONE', #32529, #38880 ) ;
#33287=EDGE_LOOP ( 'NONE', ( #14332, #5453, #41923, #47723 ) ) ;
#33288=CARTESIAN_POINT ( 'NONE',  ( 80.00000000000061107, 16.00000000000000000, -54.99999999999999289 ) ) ;
#33291=VECTOR ( 'NONE', #22086, 1000.000000000000000 ) ;
#33297=ORIENTED_EDGE ( 'NONE', *, *, #30939, .T. ) ;
#33298=ORIENTED_EDGE ( 'NONE', *, *, #19260, .F. ) ;
#33305=LINE ( 'NONE', #48381, #196 ) ;
#33306=CARTESIAN_POINT ( 'NONE',  ( -114.9999999999981526, 17.00000000000000000, 90.00000000000000000 ) ) ;
#33307=DIRECTION ( 'NONE',  ( 0.000000000000000000, 0.000000000000000000, 1.000000000000000000 ) ) ;
#33323=ORIENTED_EDGE ( 'NONE', *, *, #27740, .T. ) ;
#33328=DIRECTION ( 'NONE',  ( -1.000000000000000000, 0.000000000000000000, 0.000000000000000000 ) ) ;
#33333=DIRECTION ( 'NONE',  ( -1.000000000000000000, -0.000000000000000000, -0.000000000000000000 ) ) ;
#33347=CARTESIAN_POINT ( 'NONE',  ( -14.99999999999845812, 17.00000000000000000, 35.00000000000000000 ) ) ;
#33348=ORIENTED_EDGE ( 'NONE', *, *, #48711, .T. ) ;
#33364=AXIS2_PLACEMENT_3D ( 'NONE', #28667, #36906, #44292 ) ;
#33377=ORIENTED_EDGE ( 'NONE', *, *, #25956, .F. ) ;
#33388=ORIENTED_EDGE ( 'NONE', *, *, #5325, .F. ) ;
#33394=EDGE_CURVE ( 'NONE', #31274, #22541, #26992, .T. ) ;
#33395=LINE ( 'NONE', #32375, #47829 ) ;
#33397=CARTESIAN_POINT ( 'NONE',  ( 130.0000000000015064, 17.00000000000000000, 35.00000000000000000 ) ) ;
#33398=ORIENTED_EDGE ( 'NONE', *, *, #33668, .F. ) ;
#33410=FACE_OUTER_BOUND ( 'NONE', #45775, .T. ) ;
#33412=CARTESIAN_POINT ( 'NONE',  ( 135.0000000000019043, 16.00000000000000000, 65.00000000000000000 ) ) ;
#33413=DIRECTION ( 'NONE',  ( 0.000000000000000000, 0.000000000000000000, -1.000000000000000000 ) ) ;
#33430=DIRECTION ( 'NONE',  ( 0.000000000000000000, 0.000000000000000000, 1.000000000000000000 ) ) ;
#33433=CARTESIAN_POINT ( 'NONE',  ( 129.9999999999999432, 16.00000000000000000, -114.9999999999999858 ) ) ;
#33438=DIRECTION ( 'NONE',  ( 0.000000000000000000, 0.000000000000000000, 1.000000000000000000 ) ) ;
#33440=VECTOR ( 'NONE', #21880, 1000.000000000000000 ) ;
#33448=CARTESIAN_POINT ( 'NONE',  ( 130.0000000000002842, 16.00000000000000000, -84.99999999999998579 ) ) ;
#33450=EDGE_CURVE ( 'NONE', #32627, #31779, #45009, .T. ) ;
#33453=DIRECTION ( 'NONE',  ( -0.000000000000000000, -0.000000000000000000, -1.000000000000000000 ) ) ;
#33456=LINE ( 'NONE', #13684, #31157 ) ;
#33459=FACE_OUTER_BOUND ( 'NONE', #15029, .T. ) ;
#33460=DIRECTION ( 'NONE',  ( -0.000000000000000000, -0.000000000000000000, -1.000000000000000000 ) ) ;
#33461=EDGE_CURVE ( 'NONE', #39326, #35676, #49097, .T. ) ;
#33464=PLANE ( 'NONE',  #34935 ) ;
#33483=DIRECTION ( 'NONE',  ( -0.000000000000000000, -0.000000000000000000, 1.000000000000000000 ) ) ;
#33494=DIRECTION ( 'NONE',  ( -0.000000000000000000, -0.000000000000000000, -1.000000000000000000 ) ) ;
#33496=LINE ( 'NONE', #49085, #40531 ) ;
#33505=DIRECTION ( 'NONE',  ( -1.000000000000000000, -0.000000000000000000, -0.000000000000000000 ) ) ;
#33510=CARTESIAN_POINT ( 'NONE',  ( -64.99999999999783995, 17.00000000000000000, 95.00000000000000000 ) ) ;
#33511=CARTESIAN_POINT ( 'NONE',  ( 164.9999999999999716, 16.00000000000000000, 30.00000000000000000 ) ) ;
#33523=ORIENTED_EDGE ( 'NONE', *, *, #11111, .T. ) ;
#33528=AXIS2_PLACEMENT_3D ( 'NONE', #19151, #23534, #50152 ) ;
#33530=EDGE_LOOP ( 'NONE', ( #3131, #29040, #38899, #44238 ) ) ;
#33532=VECTOR ( 'NONE', #19281, 1000.000000000000000 ) ;
#33535=FACE_OUTER_BOUND ( 'NONE', #8100, .T. ) ;
#33538=VERTEX_POINT ( 'NONE', #34787 ) ;
#33542=VECTOR ( 'NONE', #29447, 1000.000000000000000 ) ;
#33563=LINE ( 'NONE', #40754, #33542 ) ;
#33574=FACE_OUTER_BOUND ( 'NONE', #41304, .T. ) ;
#33577=EDGE_LOOP ( 'NONE', ( #13239, #5494, #22642, #50310 ) ) ;
#33578=CARTESIAN_POINT ( 'NONE',  ( -14.99999999999782041, 17.00000000000000000, 95.00000000000000000 ) ) ;
#33595=PLANE ( 'NONE',  #28346 ) ;
#33604=ORIENTED_EDGE ( 'NONE', *, *, #15004, .T. ) ;
#33609=FACE_BOUND ( 'NONE', #24882, .T. ) ;
#33620=ORIENTED_EDGE ( 'NONE', *, *, #48365, .T. ) ;
#33622=AXIS2_PLACEMENT_3D ( 'NONE', #45205, #41397, #6257 ) ;
#33623=CARTESIAN_POINT ( 'NONE',  ( -19.99999999999971223, 17.00000000000000000, -60.00000000000000000 ) ) ;
#33625=CARTESIAN_POINT ( 'NONE',  ( -14.99999999999812594, 17.00000000000000000, 65.00000000000000000 ) ) ;
#33627=VERTEX_POINT ( 'NONE', #46264 ) ;
#33632=DIRECTION ( 'NONE',  ( -0.000000000000000000, -1.000000000000000000, -0.000000000000000000 ) ) ;
#33635=ORIENTED_EDGE ( 'NONE', *, *, #37933, .F. ) ;
#33638=CARTESIAN_POINT ( 'NONE',  ( 164.9999999999999716, 17.00000000000000000, 4.999999999999990230 ) ) ;
#33639=DIRECTION ( 'NONE',  ( 3.469446951953611231E-16, -0.000000000000000000, -1.000000000000000000 ) ) ;
#33644=CARTESIAN_POINT ( 'NONE',  ( 135.0000000000006253, 17.00000000000000000, -54.99999999999999289 ) ) ;
#33648=VECTOR ( 'NONE', #35328, 1000.000000000000000 ) ;
#33650=EDGE_LOOP ( 'NONE', ( #23695, #2345, #36189, #7698 ) ) ;
#33657=ORIENTED_EDGE ( 'NONE', *, *, #42173, .T. ) ;
#33658=DIRECTION ( 'NONE',  ( 1.000000000000000000, 0.000000000000000000, -0.000000000000000000 ) ) ;
#33660=ORIENTED_EDGE ( 'NONE', *, *, #26362, .T. ) ;
#33668=EDGE_CURVE ( 'NONE', #6629, #38277, #29897, .T. ) ;
#33675=DIRECTION ( 'NONE',  ( -0.000000000000000000, -1.000000000000000000, -0.000000000000000000 ) ) ;
#33680=ORIENTED_EDGE ( 'NONE', *, *, #45087, .T. ) ;
#33682=ADVANCED_FACE ( 'NONE', ( #14233 ), #3183, .F. ) ;
#33700=EDGE_CURVE ( 'NONE', #8841, #24012, #34518, .T. ) ;
#33707=LINE ( 'NONE', #17793, #28689 ) ;
#33712=CARTESIAN_POINT ( 'NONE',  ( 130.0000000000008811, 17.00000000000000000, -24.99999999999999289 ) ) ;
#33713=EDGE_CURVE ( 'NONE', #3086, #10429, #8331, .T. ) ;
#33715=EDGE_LOOP ( 'NONE', ( #10880, #14961, #49609, #2868 ) ) ;
#33717=DIRECTION ( 'NONE',  ( 0.000000000000000000, 0.000000000000000000, 1.000000000000000000 ) ) ;
#33718=AXIS2_PLACEMENT_3D ( 'NONE', #28588, #1409, #47296 ) ;
#33719=ORIENTED_EDGE ( 'NONE', *, *, #40312, .T. ) ;
#33722=DIRECTION ( 'NONE',  ( 0.000000000000000000, 0.000000000000000000, 1.000000000000000000 ) ) ;
#33725=DIRECTION ( 'NONE',  ( 0.000000000000000000, 0.000000000000000000, 1.000000000000000000 ) ) ;
#33730=EDGE_CURVE ( 'NONE', #46304, #50236, #43217, .T. ) ;
#33731=DIRECTION ( 'NONE',  ( 0.000000000000000000, -0.000000000000000000, -1.000000000000000000 ) ) ;
#33739=ORIENTED_EDGE ( 'NONE', *, *, #35426, .T. ) ;
#33746=DIRECTION ( 'NONE',  ( 1.000000000000000000, 0.000000000000000000, 0.000000000000000000 ) ) ;
#33753=LINE ( 'NONE', #6790, #21566 ) ;
#33766=EDGE_CURVE ( 'NONE', #33142, #614, #3709, .T. ) ;
#33771=ADVANCED_FACE ( 'NONE', ( #7830 ), #19610, .F. ) ;
#33774=DIRECTION ( 'NONE',  ( -1.000000000000000000, 0.000000000000000000, -0.000000000000000000 ) ) ;
#33778=ORIENTED_EDGE ( 'NONE', *, *, #33045, .F. ) ;
#33812=CARTESIAN_POINT ( 'NONE',  ( 164.9999999999999716, 17.00000000000000000, -114.9999999999999858 ) ) ;
#33816=EDGE_LOOP ( 'NONE', ( #17170, #7276, #34607, #6689 ) ) ;
#33818=VECTOR ( 'NONE', #38549, 1000.000000000000000 ) ;
#33826=AXIS2_PLACEMENT_3D ( 'NONE', #22630, #11081, #38803 ) ;
#33827=LINE ( 'NONE', #45583, #40133 ) ;
#33829=CARTESIAN_POINT ( 'NONE',  ( -65.00000000000002842, 17.00000000000000000, -90.00000000000000000 ) ) ;
#33830=PLANE ( 'NONE',  #25471 ) ;
#33837=ORIENTED_EDGE ( 'NONE', *, *, #39751, .F. ) ;
#33841=EDGE_CURVE ( 'NONE', #29675, #9554, #33206, .T. ) ;
#33851=LINE ( 'NONE', #11253, #14302 ) ;
#33858=VERTEX_POINT ( 'NONE', #5227 ) ;
#33866=CARTESIAN_POINT ( 'NONE',  ( 0.000000000000000000, 16.00000000000000000, 0.000000000000000000 ) ) ;
#33869=ORIENTED_EDGE ( 'NONE', *, *, #32712, .F. ) ;
#33876=DIRECTION ( 'NONE',  ( -0.000000000000000000, -0.000000000000000000, -1.000000000000000000 ) ) ;
#33879=ORIENTED_EDGE ( 'NONE', *, *, #32983, .F. ) ;
#33880=DIRECTION ( 'NONE',  ( -0.000000000000000000, -1.000000000000000000, -0.000000000000000000 ) ) ;
#33889=ORIENTED_EDGE ( 'NONE', *, *, #46791, .T. ) ;
#33899=CARTESIAN_POINT ( 'NONE',  ( 85.00000000000090949, 17.00000000000000000, 0.000000000000000000 ) ) ;
#33908=VECTOR ( 'NONE', #33483, 1000.000000000000000 ) ;
#33909=ORIENTED_EDGE ( 'NONE', *, *, #20192, .T. ) ;
#33915=LINE ( 'NONE', #50005, #7921 ) ;
#33925=DIRECTION ( 'NONE',  ( -0.000000000000000000, -0.000000000000000000, -1.000000000000000000 ) ) ;
#33926=ORIENTED_EDGE ( 'NONE', *, *, #25839, .T. ) ;
#33933=CARTESIAN_POINT ( 'NONE',  ( 85.00000000000056843, 16.00000000000000000, -54.99999999999999289 ) ) ;
#33945=LINE ( 'NONE', #26248, #9777 ) ;
#33951=LINE ( 'NONE', #6742, #35269 ) ;
#33955=CARTESIAN_POINT ( 'NONE',  ( -114.9999999999997158, 16.00000000000000000, -60.00000000000000000 ) ) ;
#33956=EDGE_CURVE ( 'NONE', #31581, #40535, #48793, .T. ) ;
#33957=VECTOR ( 'NONE', #42128, 1000.000000000000000 ) ;
#33966=LINE ( 'NONE', #13938, #37280 ) ;
#33968=DIRECTION ( 'NONE',  ( -0.000000000000000000, -0.000000000000000000, -1.000000000000000000 ) ) ;
#33974=EDGE_CURVE ( 'NONE', #46680, #34035, #16779, .T. ) ;
#33975=LINE ( 'NONE', #50320, #16073 ) ;
#33995=CARTESIAN_POINT ( 'NONE',  ( 130.0000000000002842, 17.00000000000000000, -84.99999999999998579 ) ) ;
#33997=EDGE_CURVE ( 'NONE', #10490, #22721, #18271, .T. ) ;
#34009=LINE ( 'NONE', #30148, #37678 ) ;
#34010=DIRECTION ( 'NONE',  ( 1.000000000000000000, 0.000000000000000000, -4.625929269271635797E-16 ) ) ;
#34014=FACE_OUTER_BOUND ( 'NONE', #39103, .T. ) ;
#34027=ADVANCED_FACE ( 'NONE', ( #13915 ), #21896, .F. ) ;
#34032=CARTESIAN_POINT ( 'NONE',  ( 35.00000000000122213, 17.00000000000000000, 5.000000000000004441 ) ) ;
#34034=VECTOR ( 'NONE', #50200, 1000.000000000000000 ) ;
#34035=VERTEX_POINT ( 'NONE', #10580 ) ;
#34047=ORIENTED_EDGE ( 'NONE', *, *, #40185, .T. ) ;
#34050=PLANE ( 'NONE',  #11481 ) ;
#34066=EDGE_CURVE ( 'NONE', #37688, #18558, #49784, .T. ) ;
#34077=CARTESIAN_POINT ( 'NONE',  ( -64.99999999999815259, 17.00000000000000000, 65.00000000000000000 ) ) ;
#34078=VECTOR ( 'NONE', #10194, 1000.000000000000000 ) ;
#34093=ORIENTED_EDGE ( 'NONE', *, *, #3616, .T. ) ;
#34106=DIRECTION ( 'NONE',  ( -1.000000000000000000, 0.000000000000000000, -0.000000000000000000 ) ) ;
#34109=LINE ( 'NONE', #30244, #35167 ) ;
#34119=CARTESIAN_POINT ( 'NONE',  ( -64.99999999999846523, 17.00000000000000000, 60.00000000000000000 ) ) ;
#34124=DIRECTION ( 'NONE',  ( 1.000000000000000000, 0.000000000000000000, 0.000000000000000000 ) ) ;
#34131=ORIENTED_EDGE ( 'NONE', *, *, #23753, .F. ) ;
#34132=EDGE_CURVE ( 'NONE', #21529, #5410, #8524, .T. ) ;
#34138=VECTOR ( 'NONE', #20832, 1000.000000000000000 ) ;
#34146=EDGE_CURVE ( 'NONE', #45351, #28634, #34982, .T. ) ;
#34151=VECTOR ( 'NONE', #8235, 1000.000000000000000 ) ;
#34156=VECTOR ( 'NONE', #5635, 1000.000000000000000 ) ;
#34164=VERTEX_POINT ( 'NONE', #38818 ) ;
#34167=LINE ( 'NONE', #30298, #35241 ) ;
#34173=VERTEX_POINT ( 'NONE', #19293 ) ;
#34174=DIRECTION ( 'NONE',  ( 1.000000000000000000, 0.000000000000000000, 0.000000000000000000 ) ) ;
#34175=VERTEX_POINT ( 'NONE', #15205 ) ;
#34180=DIRECTION ( 'NONE',  ( -1.000000000000000000, -0.000000000000000000, -0.000000000000000000 ) ) ;
#34191=VERTEX_POINT ( 'NONE', #42886 ) ;
#34195=DIRECTION ( 'NONE',  ( 0.000000000000000000, 0.000000000000000000, 1.000000000000000000 ) ) ;
#34214=ORIENTED_EDGE ( 'NONE', *, *, #48365, .F. ) ;
#34223=EDGE_CURVE ( 'NONE', #42678, #50118, #36235, .T. ) ;
#34226=DIRECTION ( 'NONE',  ( -0.000000000000000000, -1.000000000000000000, -0.000000000000000000 ) ) ;
#34233=DIRECTION ( 'NONE',  ( -0.000000000000000000, -1.000000000000000000, -0.000000000000000000 ) ) ;
#34236=ORIENTED_EDGE ( 'NONE', *, *, #39743, .T. ) ;
#34248=DIRECTION ( 'NONE',  ( 1.000000000000000000, 0.000000000000000000, -0.000000000000000000 ) ) ;
#34249=DIRECTION ( 'NONE',  ( 1.000000000000000000, 0.000000000000000000, 0.000000000000000000 ) ) ;
#34250=ORIENTED_EDGE ( 'NONE', *, *, #41596, .T. ) ;
#34254=DIRECTION ( 'NONE',  ( -1.000000000000000000, -0.000000000000000000, -0.000000000000000000 ) ) ;
#34268=DIRECTION ( 'NONE',  ( 0.000000000000000000, 0.000000000000000000, 1.000000000000000000 ) ) ;
#34280=ORIENTED_EDGE ( 'NONE', *, *, #7349, .F. ) ;
#34284=DIRECTION ( 'NONE',  ( -1.000000000000000000, 0.000000000000000000, 0.000000000000000000 ) ) ;
#34288=FACE_OUTER_BOUND ( 'NONE', #24529, .T. ) ;
#34289=CARTESIAN_POINT ( 'NONE',  ( -14.99999999999845812, 17.00000000000000000, 35.00000000000000000 ) ) ;
#34291=VERTEX_POINT ( 'NONE', #24929 ) ;
#34307=CARTESIAN_POINT ( 'NONE',  ( 85.00000000000123634, 17.00000000000000000, 30.00000000000000000 ) ) ;
#34308=CARTESIAN_POINT ( 'NONE',  ( -69.99999999999879208, 16.00000000000000000, 30.00000000000000000 ) ) ;
#34322=CARTESIAN_POINT ( 'NONE',  ( -114.9999999999978542, 16.00000000000000000, 115.0000000000000142 ) ) ;
#34325=DIRECTION ( 'NONE',  ( 0.000000000000000000, 0.000000000000000000, -1.000000000000000000 ) ) ;
#34326=ORIENTED_EDGE ( 'NONE', *, *, #14646, .F. ) ;
#34335=ADVANCED_FACE ( 'NONE', ( #12864 ), #32888, .F. ) ;
#34338=DIRECTION ( 'NONE',  ( 0.000000000000000000, 0.000000000000000000, 1.000000000000000000 ) ) ;
#34340=CARTESIAN_POINT ( 'NONE',  ( 135.0000000000000000, 17.00000000000000000, -90.00000000000000000 ) ) ;
#34344=LINE ( 'NONE', #3982, #37921 ) ;
#34354=ORIENTED_EDGE ( 'NONE', *, *, #24265, .T. ) ;
#34355=CARTESIAN_POINT ( 'NONE',  ( -64.99999999999940314, 16.00000000000000000, -54.99999999999999289 ) ) ;
#34362=PRODUCT_DEFINITION_SHAPE ( 'NONE', 'NONE',  #17451 ) ;
#34363=ORIENTED_EDGE ( 'NONE', *, *, #18779, .F. ) ;
#34368=CARTESIAN_POINT ( 'NONE',  ( 85.00000000000213163, 17.00000000000000000, 95.00000000000000000 ) ) ;
#34372=LINE ( 'NONE', #11011, #277 ) ;
#34377=VECTOR ( 'NONE', #12173, 1000.000000000000000 ) ;
#34384=VECTOR ( 'NONE', #14295, 1000.000000000000000 ) ;
#34387=DIRECTION ( 'NONE',  ( 1.000000000000000000, 0.000000000000000000, -0.000000000000000000 ) ) ;
#34388=CARTESIAN_POINT ( 'NONE',  ( 130.0000000000021032, 17.00000000000000000, 95.00000000000000000 ) ) ;
#34389=AXIS2_PLACEMENT_3D ( 'NONE', #39453, #39705, #19427 ) ;
#34392=EDGE_LOOP ( 'NONE', ( #3984, #321, #24312, #654 ) ) ;
#34396=FACE_OUTER_BOUND ( 'NONE', #3607, .T. ) ;
#34401=EDGE_CURVE ( 'NONE', #2527, #14054, #41326, .T. ) ;
#34402=ADVANCED_FACE ( 'NONE', ( #34396 ), #22323, .F. ) ;
#34404=DIRECTION ( 'NONE',  ( 0.000000000000000000, 0.000000000000000000, 1.000000000000000000 ) ) ;
#34414=CARTESIAN_POINT ( 'NONE',  ( 164.9999999999999716, 16.00000000000000000, 95.00000000000000000 ) ) ;
#34426=EDGE_CURVE ( 'NONE', #6173, #50118, #6178, .T. ) ;
#34428=ORIENTED_EDGE ( 'NONE', *, *, #23054, .F. ) ;
#34431=CARTESIAN_POINT ( 'NONE',  ( 30.00000000000062172, 16.00000000000000000, -30.00000000000000000 ) ) ;
#34440=EDGE_LOOP ( 'NONE', ( #47692, #23367, #5056, #30353 ) ) ;
#34445=PLANE ( 'NONE',  #23307 ) ;
#34452=EDGE_CURVE ( 'NONE', #36, #31581, #38262, .T. ) ;
#34454=ORIENTED_EDGE ( 'NONE', *, *, #34066, .T. ) ;
#34457=VECTOR ( 'NONE', #4064, 1000.000000000000000 ) ;
#34464=EDGE_CURVE ( 'NONE', #16051, #27596, #25942, .T. ) ;
#34466=VERTEX_POINT ( 'NONE', #10522 ) ;
#34474=DIRECTION ( 'NONE',  ( -0.000000000000000000, -1.000000000000000000, -0.000000000000000000 ) ) ;
#34476=EDGE_CURVE ( 'NONE', #34694, #39319, #23595, .T. ) ;
#34499=FACE_OUTER_BOUND ( 'NONE', #1936, .T. ) ;
#34503=DIRECTION ( 'NONE',  ( 1.000000000000000000, 0.000000000000000000, 0.000000000000000000 ) ) ;
#34518=LINE ( 'NONE', #18330, #18823 ) ;
#34524=CARTESIAN_POINT ( 'NONE',  ( 35.00000000000028422, 17.00000000000000000, -84.99999999999998579 ) ) ;
#34525=VECTOR ( 'NONE', #37423, 1000.000000000000000 ) ;
#34534=DIRECTION ( 'NONE',  ( -0.000000000000000000, -1.000000000000000000, -0.000000000000000000 ) ) ;
#34537=ORIENTED_EDGE ( 'NONE', *, *, #25525, .T. ) ;
#34540=CARTESIAN_POINT ( 'NONE',  ( 85.00000000000184741, 17.00000000000000000, 90.00000000000000000 ) ) ;
#34546=CARTESIAN_POINT ( 'NONE',  ( 35.00000000000186162, 16.00000000000000000, 90.00000000000000000 ) ) ;
#34547=ORIENTED_EDGE ( 'NONE', *, *, #36560, .T. ) ;
#34549=LINE ( 'NONE', #15041, #11525 ) ;
#34558=DIRECTION ( 'NONE',  ( -1.000000000000000000, 0.000000000000000000, -0.000000000000000000 ) ) ;
#34563=LINE ( 'NONE', #19412, #11954 ) ;
#34580=CARTESIAN_POINT ( 'NONE',  ( 135.0000000000021600, 17.00000000000000000, 95.00000000000000000 ) ) ;
#34583=DIRECTION ( 'NONE',  ( 1.000000000000000000, 0.000000000000000000, 0.000000000000000000 ) ) ;
#34584=ORIENTED_EDGE ( 'NONE', *, *, #46513, .F. ) ;
#34595=DIRECTION ( 'NONE',  ( 1.000000000000000000, 0.000000000000000000, 0.000000000000000000 ) ) ;
#34602=ORIENTED_EDGE ( 'NONE', *, *, #6119, .T. ) ;
#34605=ORIENTED_EDGE ( 'NONE', *, *, #46234, .T. ) ;
#34607=ORIENTED_EDGE ( 'NONE', *, *, #11772, .F. ) ;
#34608=LINE ( 'NONE', #26899, #36934 ) ;
#34616=ADVANCED_FACE ( 'NONE', ( #4101 ), #8210, .F. ) ;
#34617=FACE_BOUND ( 'NONE', #47841, .T. ) ;
#34633=ADVANCED_FACE ( 'NONE', ( #35920 ), #20252, .F. ) ;
#34634=VECTOR ( 'NONE', #36829, 1000.000000000000000 ) ;
#34638=EDGE_CURVE ( 'NONE', #5571, #17054, #36428, .T. ) ;
#34641=EDGE_CURVE ( 'NONE', #25320, #42631, #44567, .T. ) ;
#34655=ORIENTED_EDGE ( 'NONE', *, *, #24754, .F. ) ;
#34656=EDGE_CURVE ( 'NONE', #50236, #50559, #47653, .T. ) ;
#34671=DIRECTION ( 'NONE',  ( 0.000000000000000000, 0.000000000000000000, -1.000000000000000000 ) ) ;
#34684=EDGE_CURVE ( 'NONE', #10553, #37470, #6613, .T. ) ;
#34689=VERTEX_POINT ( 'NONE', #18653 ) ;
#34690=EDGE_CURVE ( 'NONE', #41862, #30294, #41515, .T. ) ;
#34694=VERTEX_POINT ( 'NONE', #22005 ) ;
#34704=DIRECTION ( 'NONE',  ( 0.000000000000000000, -0.000000000000000000, -1.000000000000000000 ) ) ;
#34706=ORIENTED_EDGE ( 'NONE', *, *, #16121, .T. ) ;
#34714=ADVANCED_FACE ( 'NONE', ( #37940 ), #18406, .F. ) ;
#34741=CARTESIAN_POINT ( 'NONE',  ( 30.00000000000029132, 17.00000000000000000, -60.00000000000000000 ) ) ;
#34745=VERTEX_POINT ( 'NONE', #13791 ) ;
#34747=VECTOR ( 'NONE', #251, 1000.000000000000000 ) ;
#34760=ORIENTED_EDGE ( 'NONE', *, *, #27735, .F. ) ;
#34768=ADVANCED_FACE ( 'NONE', ( #41013 ), #5857, .F. ) ;
#34772=VERTEX_POINT ( 'NONE', #37681 ) ;
#34774=LINE ( 'NONE', #121, #27196 ) ;
#34776=ADVANCED_FACE ( 'NONE', ( #18152 ), #33830, .F. ) ;
#34777=DIRECTION ( 'NONE',  ( 1.000000000000000000, 0.000000000000000000, -0.000000000000000000 ) ) ;
#34787=CARTESIAN_POINT ( 'NONE',  ( 85.00000000000056843, 17.00000000000000000, -54.99999999999999289 ) ) ;
#34813=DIRECTION ( 'NONE',  ( -1.000000000000000000, -0.000000000000000000, -0.000000000000000000 ) ) ;
#34827=DIRECTION ( 'NONE',  ( 0.000000000000000000, 0.000000000000000000, 1.000000000000000000 ) ) ;
#34828=DIRECTION ( 'NONE',  ( 0.000000000000000000, -1.000000000000000000, 0.000000000000000000 ) ) ;
#34830=CARTESIAN_POINT ( 'NONE',  ( -69.99999999999972999, 16.00000000000000000, -84.99999999999998579 ) ) ;
#34831=ORIENTED_EDGE ( 'NONE', *, *, #34932, .T. ) ;
#34835=DIRECTION ( 'NONE',  ( 0.000000000000000000, 0.000000000000000000, 1.000000000000000000 ) ) ;
#34849=DIRECTION ( 'NONE',  ( 1.000000000000000000, 0.000000000000000000, 0.000000000000000000 ) ) ;
#34857=AXIS2_PLACEMENT_3D ( 'NONE', #35024, #50595, #22931 ) ;
#34874=VERTEX_POINT ( 'NONE', #49910 ) ;
#34875=EDGE_LOOP ( 'NONE', ( #12045, #20251, #19612, #32454 ) ) ;
#34876=LINE ( 'NONE', #46865, #22968 ) ;
#34893=VECTOR ( 'NONE', #5456, 1000.000000000000000 ) ;
#34898=CARTESIAN_POINT ( 'NONE',  ( 79.99999999999997158, 17.00000000000000000, -90.00000000000000000 ) ) ;
#34904=LINE ( 'NONE', #15634, #45476 ) ;
#34906=ORIENTED_EDGE ( 'NONE', *, *, #22992, .F. ) ;
#34908=ORIENTED_EDGE ( 'NONE', *, *, #35568, .T. ) ;
#34919=EDGE_CURVE ( 'NONE', #907, #20271, #4731, .T. ) ;
#34932=EDGE_CURVE ( 'NONE', #18558, #21591, #29096, .T. ) ;
#34935=AXIS2_PLACEMENT_3D ( 'NONE', #10851, #7007, #30110 ) ;
#34936=CARTESIAN_POINT ( 'NONE',  ( 130.0000000000008811, 17.00000000000000000, -24.99999999999999289 ) ) ;
#34943=FACE_OUTER_BOUND ( 'NONE', #20888, .T. ) ;
#34947=PLANE ( 'NONE',  #43797 ) ;
#34951=VECTOR ( 'NONE', #4691, 1000.000000000000000 ) ;
#34962=DIRECTION ( 'NONE',  ( 0.000000000000000000, -0.000000000000000000, -1.000000000000000000 ) ) ;
#34964=EDGE_CURVE ( 'NONE', #32976, #28202, #17542, .T. ) ;
#34967=AXIS2_PLACEMENT_3D ( 'NONE', #50144, #22496, #3233 ) ;
#34972=CARTESIAN_POINT ( 'NONE',  ( -114.9999999999994031, 17.00000000000000000, -54.99999999999999289 ) ) ;
#34974=EDGE_CURVE ( 'NONE', #4263, #30568, #48799, .T. ) ;
#34982=LINE ( 'NONE', #42636, #8226 ) ;
#34986=PLANE ( 'NONE',  #8138 ) ;
#34987=AXIS2_PLACEMENT_3D ( 'NONE', #24334, #43039, #24073 ) ;
#34997=ADVANCED_FACE ( 'NONE', ( #9835 ), #20883, .F. ) ;
#35000=ADVANCED_FACE ( 'NONE', ( #29590 ), #32449, .F. ) ;
#35006=ORIENTED_EDGE ( 'NONE', *, *, #25509, .F. ) ;
#35012=VECTOR ( 'NONE', #7402, 1000.000000000000000 ) ;
#35015=ORIENTED_EDGE ( 'NONE', *, *, #26413, .F. ) ;
#35016=ORIENTED_EDGE ( 'NONE', *, *, #33394, .T. ) ;
#35020=LINE ( 'NONE', #15487, #37186 ) ;
#35024=CARTESIAN_POINT ( 'NONE',  ( 35.00000000000028422, 17.00000000000000000, -60.00000000000000000 ) ) ;
#35026=DIRECTION ( 'NONE',  ( 1.000000000000000000, 0.000000000000000000, 0.000000000000000000 ) ) ;
#35033=ORIENTED_EDGE ( 'NONE', *, *, #6400, .F. ) ;
#35034=ORIENTED_EDGE ( 'NONE', *, *, #49025, .F. ) ;
#35045=DIRECTION ( 'NONE',  ( 0.000000000000000000, -1.000000000000000000, 0.000000000000000000 ) ) ;
#35057=EDGE_CURVE ( 'NONE', #16051, #36968, #26260, .T. ) ;
#35070=DIRECTION ( 'NONE',  ( 0.000000000000000000, 0.000000000000000000, 1.000000000000000000 ) ) ;
#35073=ORIENTED_EDGE ( 'NONE', *, *, #2670, .F. ) ;
#35102=DIRECTION ( 'NONE',  ( -1.000000000000000000, -0.000000000000000000, -0.000000000000000000 ) ) ;
#35105=DIRECTION ( 'NONE',  ( 1.000000000000000000, 0.000000000000000000, -0.000000000000000000 ) ) ;
#35117=ADVANCED_FACE ( 'NONE', ( #4680 ), #47731, .F. ) ;
#35119=ORIENTED_EDGE ( 'NONE', *, *, #1775, .T. ) ;
#35167=VECTOR ( 'NONE', #49443, 1000.000000000000000 ) ;
#35171=DIRECTION ( 'NONE',  ( 1.000000000000000000, 0.000000000000000000, 0.000000000000000000 ) ) ;
#35173=ORIENTED_EDGE ( 'NONE', *, *, #22506, .F. ) ;
#35175=ORIENTED_EDGE ( 'NONE', *, *, #48664, .T. ) ;
#35178=EDGE_LOOP ( 'NONE', ( #32118, #42784, #25052, #39573 ) ) ;
#35185=ORIENTED_EDGE ( 'NONE', *, *, #12452, .T. ) ;
#35187=CARTESIAN_POINT ( 'NONE',  ( 85.00000000000090949, 17.00000000000000000, 0.000000000000000000 ) ) ;
#35192=CARTESIAN_POINT ( 'NONE',  ( -69.99999999999783995, 17.00000000000000000, 115.0000000000000142 ) ) ;
#35196=PLANE ( 'NONE',  #4164 ) ;
#35198=AXIS2_PLACEMENT_3D ( 'NONE', #48532, #28326, #13174 ) ;
#35199=ORIENTED_EDGE ( 'NONE', *, *, #45305, .F. ) ;
#35228=ORIENTED_EDGE ( 'NONE', *, *, #7694, .T. ) ;
#35238=VERTEX_POINT ( 'NONE', #23665 ) ;
#35241=VECTOR ( 'NONE', #25952, 1000.000000000000000 ) ;
#35246=VERTEX_POINT ( 'NONE', #8533 ) ;
#35249=ORIENTED_EDGE ( 'NONE', *, *, #15004, .F. ) ;
#35256=VERTEX_POINT ( 'NONE', #31117 ) ;
#35257=VERTEX_POINT ( 'NONE', #27772 ) ;
#35269=VECTOR ( 'NONE', #15453, 1000.000000000000000 ) ;
#35282=DIRECTION ( 'NONE',  ( 0.000000000000000000, 0.000000000000000000, -1.000000000000000000 ) ) ;
#35284=EDGE_CURVE ( 'NONE', #30177, #41895, #50560, .T. ) ;
#35286=VECTOR ( 'NONE', #9716, 1000.000000000000000 ) ;
#35288=EDGE_CURVE ( 'NONE', #26701, #11387, #8788, .T. ) ;
#35290=DIRECTION ( 'NONE',  ( 0.000000000000000000, 0.000000000000000000, 1.000000000000000000 ) ) ;
#35296=ORIENTED_EDGE ( 'NONE', *, *, #36928, .F. ) ;
#35301=VERTEX_POINT ( 'NONE', #5671 ) ;
#35309=ADVANCED_FACE ( 'NONE', ( #1082 ), #16980, .F. ) ;
#35320=EDGE_CURVE ( 'NONE', #16290, #50318, #9280, .T. ) ;
#35325=PLANE ( 'NONE',  #30708 ) ;
#35328=DIRECTION ( 'NONE',  ( 0.000000000000000000, 0.000000000000000000, 1.000000000000000000 ) ) ;
#35339=DIRECTION ( 'NONE',  ( 1.000000000000000000, 0.000000000000000000, -0.000000000000000000 ) ) ;
#35351=EDGE_CURVE ( 'NONE', #3258, #41868, #24938, .T. ) ;
#35364=ORIENTED_EDGE ( 'NONE', *, *, #35984, .T. ) ;
#35371=EDGE_LOOP ( 'NONE', ( #43978, #11186, #2573, #16923 ) ) ;
#35375=EDGE_CURVE ( 'NONE', #418, #13598, #30546, .T. ) ;
#35380=ORIENTED_EDGE ( 'NONE', *, *, #12101, .T. ) ;
#35389=ORIENTED_EDGE ( 'NONE', *, *, #15214, .T. ) ;
#35392=VECTOR ( 'NONE', #50039, 1000.000000000000000 ) ;
#35413=DIRECTION ( 'NONE',  ( 0.000000000000000000, 0.000000000000000000, -1.000000000000000000 ) ) ;
#35426=EDGE_CURVE ( 'NONE', #3803, #30626, #3078, .T. ) ;
#35432=DIRECTION ( 'NONE',  ( -0.000000000000000000, -0.000000000000000000, -1.000000000000000000 ) ) ;
#35442=PLANE ( 'NONE',  #31904 ) ;
#35445=LINE ( 'NONE', #4377, #14741 ) ;
#35448=ORIENTED_EDGE ( 'NONE', *, *, #39743, .F. ) ;
#35452=LINE ( 'NONE', #15423, #48662 ) ;
#35461=ORIENTED_EDGE ( 'NONE', *, *, #4340, .T. ) ;
#35468=VECTOR ( 'NONE', #9606, 1000.000000000000000 ) ;
#35499=AXIS2_PLACEMENT_3D ( 'NONE', #12459, #50406, #16319 ) ;
#35504=CARTESIAN_POINT ( 'NONE',  ( -119.9999999999978400, 17.00000000000000000, 95.00000000000000000 ) ) ;
#35505=EDGE_CURVE ( 'NONE', #32969, #19150, #7198, .T. ) ;
#35513=CARTESIAN_POINT ( 'NONE',  ( 164.9999999999999716, 17.00000000000000000, -1.387778780781445676E-14 ) ) ;
#35523=VERTEX_POINT ( 'NONE', #30295 ) ;
#35525=CARTESIAN_POINT ( 'NONE',  ( 164.9999999999999716, 17.00000000000000000, 115.0000000000000142 ) ) ;
#35541=FACE_OUTER_BOUND ( 'NONE', #313, .T. ) ;
#35542=EDGE_LOOP ( 'NONE', ( #36135, #39083, #13063, #9581 ) ) ;
#35545=CARTESIAN_POINT ( 'NONE',  ( 30.00000000000029132, 16.00000000000000000, -60.00000000000000000 ) ) ;
#35548=EDGE_CURVE ( 'NONE', #45538, #14054, #17967, .T. ) ;
#35549=EDGE_CURVE ( 'NONE', #14126, #30097, #14118, .T. ) ;
#35553=( GEOMETRIC_REPRESENTATION_CONTEXT ( 3 ) GLOBAL_UNCERTAINTY_ASSIGNED_CONTEXT ( ( #23514 ) ) GLOBAL_UNIT_ASSIGNED_CONTEXT ( ( #13364, #17962, #41079 ) ) REPRESENTATION_CONTEXT ( 'NONE', 'WORKASPACE' ) );
#35555=EDGE_CURVE ( 'NONE', #46181, #11387, #16167, .T. ) ;
#35562=ORIENTED_EDGE ( 'NONE', *, *, #45374, .T. ) ;
#35563=ORIENTED_EDGE ( 'NONE', *, *, #34656, .F. ) ;
#35568=EDGE_CURVE ( 'NONE', #41244, #22918, #15404, .T. ) ;
#35572=CARTESIAN_POINT ( 'NONE',  ( 35.00000000000186162, 16.00000000000000000, 90.00000000000000000 ) ) ;
#35573=LINE ( 'NONE', #15548, #10700 ) ;
#35574=ORIENTED_EDGE ( 'NONE', *, *, #32920, .T. ) ;
#35583=CARTESIAN_POINT ( 'NONE',  ( -114.9999999999981526, 17.00000000000000000, 65.00000000000000000 ) ) ;
#35584=DIRECTION ( 'NONE',  ( -0.000000000000000000, -0.000000000000000000, -1.000000000000000000 ) ) ;
#35587=CARTESIAN_POINT ( 'NONE',  ( 30.00000000000092726, 17.00000000000000000, -24.99999999999999289 ) ) ;
#35593=VECTOR ( 'NONE', #46888, 1000.000000000000000 ) ;
#35596=PLANE ( 'NONE',  #44064 ) ;
#35603=EDGE_CURVE ( 'NONE', #28634, #11806, #12302, .T. ) ;
#35615=ORIENTED_EDGE ( 'NONE', *, *, #32781, .F. ) ;
#35624=VECTOR ( 'NONE', #3921, 1000.000000000000000 ) ;
#35629=ORIENTED_EDGE ( 'NONE', *, *, #3841, .T. ) ;
#35638=DIRECTION ( 'NONE',  ( -0.000000000000000000, -1.000000000000000000, -0.000000000000000000 ) ) ;
#35643=CARTESIAN_POINT ( 'NONE',  ( 135.0000000000003411, 17.00000000000000000, -60.00000000000000000 ) ) ;
#35644=EDGE_CURVE ( 'NONE', #42413, #22765, #43101, .T. ) ;
#35651=LINE ( 'NONE', #27419, #48699 ) ;
#35660=CARTESIAN_POINT ( 'NONE',  ( -114.9999999999997158, 17.00000000000000000, -60.00000000000000000 ) ) ;
#35667=CARTESIAN_POINT ( 'NONE',  ( -64.99999999999877787, 17.00000000000000000, 5.000000000000004441 ) ) ;
#35671=DIRECTION ( 'NONE',  ( -0.000000000000000000, -1.000000000000000000, -0.000000000000000000 ) ) ;
#35676=VERTEX_POINT ( 'NONE', #43852 ) ;
#35680=EDGE_CURVE ( 'NONE', #44903, #23347, #40271, .T. ) ;
#35688=LINE ( 'NONE', #39271, #311 ) ;
#35690=VERTEX_POINT ( 'NONE', #5609 ) ;
#35699=ADVANCED_FACE ( 'NONE', ( #24623 ), #25373, .F. ) ;
#35701=VECTOR ( 'NONE', #15112, 1000.000000000000000 ) ;
#35703=VECTOR ( 'NONE', #16673, 1000.000000000000000 ) ;
#35715=EDGE_CURVE ( 'NONE', #25915, #48491, #13056, .T. ) ;
#35720=EDGE_CURVE ( 'NONE', #36600, #7468, #36178, .T. ) ;
#35737=VERTEX_POINT ( 'NONE', #17168 ) ;
#35754=LINE ( 'NONE', #11873, #38843 ) ;
#35760=VECTOR ( 'NONE', #26703, 1000.000000000000000 ) ;
#35761=EDGE_CURVE ( 'NONE', #11032, #11806, #1526, .T. ) ;
#35762=VERTEX_POINT ( 'NONE', #16929 ) ;
#35765=CARTESIAN_POINT ( 'NONE',  ( 130.0000000000015064, 17.00000000000000000, 35.00000000000000000 ) ) ;
#35777=VERTEX_POINT ( 'NONE', #37448 ) ;
#35779=ORIENTED_EDGE ( 'NONE', *, *, #36329, .F. ) ;
#35781=EDGE_CURVE ( 'NONE', #5809, #32394, #25627, .T. ) ;
#35785=DIRECTION ( 'NONE',  ( 0.000000000000000000, -0.000000000000000000, -1.000000000000000000 ) ) ;
#35794=LINE ( 'NONE', #28314, #14342 ) ;
#35806=PLANE ( 'NONE',  #35198 ) ;
#35813=VECTOR ( 'NONE', #13326, 1000.000000000000000 ) ;
#35815=CARTESIAN_POINT ( 'NONE',  ( 35.00000000000152767, 16.00000000000000000, 35.00000000000000000 ) ) ;
#35819=DIRECTION ( 'NONE',  ( 0.000000000000000000, -1.000000000000000000, 0.000000000000000000 ) ) ;
#35820=AXIS2_PLACEMENT_3D ( 'NONE', #29231, #17676, #22528 ) ;
#35825=FACE_OUTER_BOUND ( 'NONE', #47676, .T. ) ;
#35838=ADVANCED_FACE ( 'NONE', ( #14826 ), #30481, .F. ) ;
#35848=CARTESIAN_POINT ( 'NONE',  ( 35.00000000000028422, 17.00000000000000000, -60.00000000000000000 ) ) ;
#35850=CARTESIAN_POINT ( 'NONE',  ( 29.99999999999998579, 17.00000000000000000, -90.00000000000000000 ) ) ;
#35865=ORIENTED_EDGE ( 'NONE', *, *, #23099, .F. ) ;
#35879=DIRECTION ( 'NONE',  ( -1.000000000000000000, 0.000000000000000000, -0.000000000000000000 ) ) ;
#35886=ORIENTED_EDGE ( 'NONE', *, *, #35644, .F. ) ;
#35887=ORIENTED_EDGE ( 'NONE', *, *, #28790, .F. ) ;
#35895=DIRECTION ( 'NONE',  ( 0.000000000000000000, 0.000000000000000000, 1.000000000000000000 ) ) ;
#35904=PLANE ( 'NONE',  #30552 ) ;
#35905=LINE ( 'NONE', #20733, #30154 ) ;
#35913=EDGE_CURVE ( 'NONE', #37462, #19934, #29983, .T. ) ;
#35920=FACE_OUTER_BOUND ( 'NONE', #39428, .T. ) ;
#35931=CARTESIAN_POINT ( 'NONE',  ( -69.99999999999940314, 17.00000000000000000, -30.00000000000000000 ) ) ;
#35934=DIRECTION ( 'NONE',  ( 0.000000000000000000, 0.000000000000000000, 1.000000000000000000 ) ) ;
#35946=LINE ( 'NONE', #781, #40891 ) ;
#35965=AXIS2_PLACEMENT_3D ( 'NONE', #19852, #24984, #20617 ) ;
#35975=EDGE_CURVE ( 'NONE', #43110, #24017, #11493, .T. ) ;
#35976=VERTEX_POINT ( 'NONE', #12245 ) ;
#35984=EDGE_CURVE ( 'NONE', #29962, #42166, #46596, .T. ) ;
#36002=FACE_OUTER_BOUND ( 'NONE', #44047, .T. ) ;
#36003=VECTOR ( 'NONE', #11456, 1000.000000000000000 ) ;
#36005=ORIENTED_EDGE ( 'NONE', *, *, #12915, .F. ) ;
#36006=DIRECTION ( 'NONE',  ( -1.000000000000000000, 0.000000000000000000, -0.000000000000000000 ) ) ;
#36008=LINE ( 'NONE', #8546, #30499 ) ;
#36028=FACE_OUTER_BOUND ( 'NONE', #12562, .T. ) ;
#36034=ORIENTED_EDGE ( 'NONE', *, *, #24672, .F. ) ;
#36048=EDGE_CURVE ( 'NONE', #22765, #14851, #31512, .T. ) ;
#36049=ADVANCED_FACE ( 'NONE', ( #5042 ), #16865, .F. ) ;
#36058=VERTEX_POINT ( 'NONE', #1220 ) ;
#36063=LINE ( 'NONE', #47301, #34634 ) ;
#36065=DIRECTION ( 'NONE',  ( -0.000000000000000000, -1.000000000000000000, -0.000000000000000000 ) ) ;
#36078=EDGE_CURVE ( 'NONE', #30725, #29367, #39970, .T. ) ;
#36089=VECTOR ( 'NONE', #47732, 1000.000000000000000 ) ;
#36095=DIRECTION ( 'NONE',  ( -1.000000000000000000, 0.000000000000000000, 0.000000000000000000 ) ) ;
#36104=DIRECTION ( 'NONE',  ( -1.000000000000000000, -0.000000000000000000, -0.000000000000000000 ) ) ;
#36114=AXIS2_PLACEMENT_3D ( 'NONE', #35643, #42786, #11261 ) ;
#36115=VECTOR ( 'NONE', #17192, 1000.000000000000000 ) ;
#36117=AXIS2_PLACEMENT_3D ( 'NONE', #29450, #41006, #40252 ) ;
#36123=CARTESIAN_POINT ( 'NONE',  ( 130.0000000000012221, 16.00000000000000000, 30.00000000000000000 ) ) ;
#36126=FACE_OUTER_BOUND ( 'NONE', #33816, .T. ) ;
#36127=VERTEX_POINT ( 'NONE', #36123 ) ;
#36130=DIRECTION ( 'NONE',  ( -1.000000000000000000, -0.000000000000000000, -0.000000000000000000 ) ) ;
#36135=ORIENTED_EDGE ( 'NONE', *, *, #12404, .T. ) ;
#36139=ORIENTED_EDGE ( 'NONE', *, *, #26929, .T. ) ;
#36140=EDGE_CURVE ( 'NONE', #50570, #45326, #20201, .T. ) ;
#36150=PLANE ( 'NONE',  #44656 ) ;
#36161=ORIENTED_EDGE ( 'NONE', *, *, #17824, .F. ) ;
#36178=LINE ( 'NONE', #21511, #36888 ) ;
#36181=PLANE ( 'NONE',  #36904 ) ;
#36189=ORIENTED_EDGE ( 'NONE', *, *, #44978, .F. ) ;
#36203=LINE ( 'NONE', #789, #7389 ) ;
#36207=ORIENTED_EDGE ( 'NONE', *, *, #2908, .T. ) ;
#36208=DIRECTION ( 'NONE',  ( 0.000000000000000000, -0.000000000000000000, -1.000000000000000000 ) ) ;
#36210=VECTOR ( 'NONE', #34233, 1000.000000000000000 ) ;
#36220=PLANE ( 'NONE',  #20736 ) ;
#36235=LINE ( 'NONE', #16471, #25430 ) ;
#36241=ORIENTED_EDGE ( 'NONE', *, *, #11922, .F. ) ;
#36243=LINE ( 'NONE', #40581, #11413 ) ;
#36254=VECTOR ( 'NONE', #49282, 1000.000000000000000 ) ;
#36262=CARTESIAN_POINT ( 'NONE',  ( 164.9999999999999716, 16.00000000000000000, -24.99999999999999289 ) ) ;
#36265=CARTESIAN_POINT ( 'NONE',  ( 135.0000000000000000, 17.00000000000000000, -114.9999999999999858 ) ) ;
#36267=DIRECTION ( 'NONE',  ( 1.000000000000000000, 0.000000000000000000, 0.000000000000000000 ) ) ;
#36271=ORIENTED_EDGE ( 'NONE', *, *, #44298, .F. ) ;
#36275=DIRECTION ( 'NONE',  ( 1.000000000000000000, 0.000000000000000000, -0.000000000000000000 ) ) ;
#36276=DIRECTION ( 'NONE',  ( -1.000000000000000000, 0.000000000000000000, 0.000000000000000000 ) ) ;
#36301=CARTESIAN_POINT ( 'NONE',  ( -164.9999999999990905, 17.00000000000000000, -24.99999999999999289 ) ) ;
#36312=VECTOR ( 'NONE', #33413, 1000.000000000000000 ) ;
#36326=ORIENTED_EDGE ( 'NONE', *, *, #29694, .F. ) ;
#36329=EDGE_CURVE ( 'NONE', #45864, #43342, #50631, .T. ) ;
#36356=VECTOR ( 'NONE', #45312, 1000.000000000000000 ) ;
#36374=CARTESIAN_POINT ( 'NONE',  ( -165.0000000000000284, 16.00000000000000000, -114.9999999999999858 ) ) ;
#36379=EDGE_LOOP ( 'NONE', ( #8665, #2415, #47918, #24886 ) ) ;
#36382=ORIENTED_EDGE ( 'NONE', *, *, #29686, .F. ) ;
#36383=ORIENTED_EDGE ( 'NONE', *, *, #21469, .F. ) ;
#36393=VECTOR ( 'NONE', #42337, 1000.000000000000000 ) ;
#36394=ORIENTED_EDGE ( 'NONE', *, *, #2138, .T. ) ;
#36400=DIRECTION ( 'NONE',  ( -0.000000000000000000, -0.000000000000000000, -1.000000000000000000 ) ) ;
#36403=DIRECTION ( 'NONE',  ( -1.000000000000000000, -0.000000000000000000, -0.000000000000000000 ) ) ;
#36417=DIRECTION ( 'NONE',  ( -0.000000000000000000, -1.000000000000000000, -0.000000000000000000 ) ) ;
#36420=LINE ( 'NONE', #42193, #25354 ) ;
#36428=LINE ( 'NONE', #43842, #7334 ) ;
#36432=ORIENTED_EDGE ( 'NONE', *, *, #12452, .F. ) ;
#36446=ORIENTED_EDGE ( 'NONE', *, *, #15994, .T. ) ;
#36454=ORIENTED_EDGE ( 'NONE', *, *, #14862, .F. ) ;
#36470=ORIENTED_EDGE ( 'NONE', *, *, #8476, .T. ) ;
#36481=ADVANCED_FACE ( 'NONE', ( #35825 ), #1162, .F. ) ;
#36482=ORIENTED_EDGE ( 'NONE', *, *, #1734, .F. ) ;
#36485=EDGE_LOOP ( 'NONE', ( #38769, #48014, #43993, #36734 ) ) ;
#36493=CARTESIAN_POINT ( 'NONE',  ( 135.0000000000003411, 16.00000000000000000, -60.00000000000000000 ) ) ;
#36506=VERTEX_POINT ( 'NONE', #39912 ) ;
#36510=AXIS2_PLACEMENT_3D ( 'NONE', #23187, #7285, #43198 ) ;
#36512=PLANE ( 'NONE',  #17577 ) ;
#36516=DIRECTION ( 'NONE',  ( -0.000000000000000000, -0.000000000000000000, -1.000000000000000000 ) ) ;
#36525=EDGE_CURVE ( 'NONE', #29858, #36660, #36063, .T. ) ;
#36528=VECTOR ( 'NONE', #25607, 1000.000000000000000 ) ;
#36554=LINE ( 'NONE', #43709, #20661 ) ;
#36558=CARTESIAN_POINT ( 'NONE',  ( -119.9999999999990905, 17.00000000000000000, -24.99999999999999289 ) ) ;
#36560=EDGE_CURVE ( 'NONE', #38860, #16290, #22601, .T. ) ;
#36561=CARTESIAN_POINT ( 'NONE',  ( 130.0000000000021032, 17.00000000000000000, 95.00000000000000000 ) ) ;
#36600=VERTEX_POINT ( 'NONE', #34414 ) ;
#36601=ORIENTED_EDGE ( 'NONE', *, *, #22880, .F. ) ;
#36607=CARTESIAN_POINT ( 'NONE',  ( 35.00000000000216716, 17.00000000000000000, 95.00000000000000000 ) ) ;
#36613=EDGE_CURVE ( 'NONE', #50318, #31422, #13695, .T. ) ;
#36625=CARTESIAN_POINT ( 'NONE',  ( 130.0000000000002842, 16.00000000000000000, -60.00000000000000000 ) ) ;
#36635=CARTESIAN_POINT ( 'NONE',  ( 85.00000000000213163, 16.00000000000000000, 95.00000000000000000 ) ) ;
#36640=LINE ( 'NONE', #36374, #38191 ) ;
#36641=EDGE_CURVE ( 'NONE', #16065, #6629, #30558, .T. ) ;
#36646=CARTESIAN_POINT ( 'NONE',  ( 135.0000000000015632, 17.00000000000000000, 60.00000000000000000 ) ) ;
#36655=CARTESIAN_POINT ( 'NONE',  ( -164.9999999999990905, 16.00000000000000000, -24.99999999999999289 ) ) ;
#36660=VERTEX_POINT ( 'NONE', #12561 ) ;
#36665=VECTOR ( 'NONE', #45726, 1000.000000000000000 ) ;
#36670=DIRECTION ( 'NONE',  ( -1.000000000000000000, -0.000000000000000000, -0.000000000000000000 ) ) ;
#36675=DIRECTION ( 'NONE',  ( -0.000000000000000000, -1.000000000000000000, -0.000000000000000000 ) ) ;
#36682=DIRECTION ( 'NONE',  ( -0.000000000000000000, -1.000000000000000000, -0.000000000000000000 ) ) ;
#36688=EDGE_CURVE ( 'NONE', #35301, #44339, #28230, .T. ) ;
#36690=PLANE ( 'NONE',  #18817 ) ;
#36691=ORIENTED_EDGE ( 'NONE', *, *, #6538, .T. ) ;
#36721=ORIENTED_EDGE ( 'NONE', *, *, #7190, .T. ) ;
#36724=EDGE_LOOP ( 'NONE', ( #41969, #11485, #28822, #25121 ) ) ;
#36726=LINE ( 'NONE', #25652, #48318 ) ;
#36728=ORIENTED_EDGE ( 'NONE', *, *, #39395, .F. ) ;
#36734=ORIENTED_EDGE ( 'NONE', *, *, #48490, .T. ) ;
#36736=VERTEX_POINT ( 'NONE', #34936 ) ;
#36776=FACE_OUTER_BOUND ( 'NONE', #40968, .T. ) ;
#36778=VECTOR ( 'NONE', #123, 1000.000000000000000 ) ;
#36786=EDGE_LOOP ( 'NONE', ( #6520, #33298, #29105, #39658 ) ) ;
#36790=CARTESIAN_POINT ( 'NONE',  ( -64.99999999999783995, 17.00000000000000000, 115.0000000000000142 ) ) ;
#36800=CARTESIAN_POINT ( 'NONE',  ( -119.9999999999994174, 17.00000000000000000, -54.99999999999999289 ) ) ;
#36801=CARTESIAN_POINT ( 'NONE',  ( 80.00000000000153477, 17.00000000000000000, 60.00000000000000000 ) ) ;
#36808=VECTOR ( 'NONE', #50344, 1000.000000000000000 ) ;
#36819=ORIENTED_EDGE ( 'NONE', *, *, #13028, .F. ) ;
#36823=ADVANCED_FACE ( 'NONE', ( #25 ), #15660, .F. ) ;
#36826=VECTOR ( 'NONE', #42522, 1000.000000000000000 ) ;
#36829=DIRECTION ( 'NONE',  ( 1.000000000000000000, 0.000000000000000000, -4.625929269271584521E-16 ) ) ;
#36833=ORIENTED_EDGE ( 'NONE', *, *, #17539, .F. ) ;
#36834=ORIENTED_EDGE ( 'NONE', *, *, #40232, .F. ) ;
#36835=ORIENTED_EDGE ( 'NONE', *, *, #45604, .T. ) ;
#36836=ADVANCED_FACE ( 'NONE', ( #4858 ), #40530, .F. ) ;
#36846=ORIENTED_EDGE ( 'NONE', *, *, #48830, .F. ) ;
#36862=ORIENTED_EDGE ( 'NONE', *, *, #3616, .F. ) ;
#36865=DIRECTION ( 'NONE',  ( 0.000000000000000000, 0.000000000000000000, 1.000000000000000000 ) ) ;
#36874=CARTESIAN_POINT ( 'NONE',  ( 175.0000000000000000, 0.000000000000000000, 122.5000000000000142 ) ) ;
#36878=LINE ( 'NONE', #9894, #25650 ) ;
#36881=DIRECTION ( 'NONE',  ( 0.000000000000000000, 0.000000000000000000, 1.000000000000000000 ) ) ;
#36888=VECTOR ( 'NONE', #1020, 1000.000000000000000 ) ;
#36889=LINE ( 'NONE', #6054, #28359 ) ;
#36894=ORIENTED_EDGE ( 'NONE', *, *, #12915, .T. ) ;
#36897=EDGE_LOOP ( 'NONE', ( #3674, #31595, #651, #32749 ) ) ;
#36898=ORIENTED_EDGE ( 'NONE', *, *, #49926, .F. ) ;
#36904=AXIS2_PLACEMENT_3D ( 'NONE', #4852, #16660, #20265 ) ;
#36906=DIRECTION ( 'NONE',  ( 0.000000000000000000, -1.000000000000000000, 0.000000000000000000 ) ) ;
#36907=DIRECTION ( 'NONE',  ( -1.000000000000000000, 0.000000000000000000, 0.000000000000000000 ) ) ;
#36911=ORIENTED_EDGE ( 'NONE', *, *, #32781, .T. ) ;
#36922=DIRECTION ( 'NONE',  ( 0.000000000000000000, -0.000000000000000000, -1.000000000000000000 ) ) ;
#36923=DIRECTION ( 'NONE',  ( 0.000000000000000000, 0.000000000000000000, 1.000000000000000000 ) ) ;
#36924=EDGE_CURVE ( 'NONE', #2086, #14979, #46092, .T. ) ;
#36928=EDGE_CURVE ( 'NONE', #40248, #27664, #41776, .T. ) ;
#36931=VECTOR ( 'NONE', #30043, 1000.000000000000000 ) ;
#36933=EDGE_LOOP ( 'NONE', ( #2579, #30467, #4568, #41323 ) ) ;
#36934=VECTOR ( 'NONE', #39483, 1000.000000000000000 ) ;
#36941=CARTESIAN_POINT ( 'NONE',  ( 85.00000000000123634, 17.00000000000000000, 5.000000000000004441 ) ) ;
#36952=DIRECTION ( 'NONE',  ( 1.000000000000000000, 0.000000000000000000, 0.000000000000000000 ) ) ;
#36966=CARTESIAN_POINT ( 'NONE',  ( -64.99999999999940314, 17.00000000000000000, -30.00000000000000000 ) ) ;
#36968=VERTEX_POINT ( 'NONE', #49928 ) ;
#36971=DIRECTION ( 'NONE',  ( 0.000000000000000000, 0.000000000000000000, 1.000000000000000000 ) ) ;
#36979=EDGE_CURVE ( 'NONE', #1481, #11106, #26385, .T. ) ;
#36993=CARTESIAN_POINT ( 'NONE',  ( -64.99999999999815259, 16.00000000000000000, 65.00000000000000000 ) ) ;
#37024=ORIENTED_EDGE ( 'NONE', *, *, #37397, .T. ) ;
#37029=VECTOR ( 'NONE', #37404, 1000.000000000000000 ) ;
#37031=ORIENTED_EDGE ( 'NONE', *, *, #7749, .F. ) ;
#37038=CARTESIAN_POINT ( 'NONE',  ( 164.9999999999999716, 17.00000000000000000, 4.999999999999990230 ) ) ;
#37043=ORIENTED_EDGE ( 'NONE', *, *, #2483, .T. ) ;
#37053=EDGE_CURVE ( 'NONE', #6217, #50559, #47767, .T. ) ;
#37063=LINE ( 'NONE', #9336, #6151 ) ;
#37064=DIRECTION ( 'NONE',  ( -0.000000000000000000, -1.000000000000000000, -0.000000000000000000 ) ) ;
#37066=ORIENTED_EDGE ( 'NONE', *, *, #1148, .T. ) ;
#37068=CARTESIAN_POINT ( 'NONE',  ( 85.00000000000090949, 16.00000000000000000, -24.99999999999999289 ) ) ;
#37075=CARTESIAN_POINT ( 'NONE',  ( 164.9999999999999716, 17.00000000000000000, 90.00000000000000000 ) ) ;
#37092=CARTESIAN_POINT ( 'NONE',  ( 0.000000000000000000, 17.00000000000000000, 0.000000000000000000 ) ) ;
#37094=CARTESIAN_POINT ( 'NONE',  ( -20.00000000000003197, 17.00000000000000000, -90.00000000000000000 ) ) ;
#37101=DIRECTION ( 'NONE',  ( 1.000000000000000000, 0.000000000000000000, 0.000000000000000000 ) ) ;
#37120=LINE ( 'NONE', #5792, #4205 ) ;
#37139=EDGE_LOOP ( 'NONE', ( #5690, #12410, #30949, #42722 ) ) ;
#37143=ORIENTED_EDGE ( 'NONE', *, *, #7544, .F. ) ;
#37158=ORIENTED_EDGE ( 'NONE', *, *, #12225, .F. ) ;
#37163=CARTESIAN_POINT ( 'NONE',  ( 135.0000000000003411, 17.00000000000000000, -84.99999999999998579 ) ) ;
#37165=VECTOR ( 'NONE', #25361, 1000.000000000000000 ) ;
#37167=PLANE ( 'NONE',  #24138 ) ;
#37171=DIRECTION ( 'NONE',  ( 1.000000000000000000, 0.000000000000000000, -0.000000000000000000 ) ) ;
#37173=DIRECTION ( 'NONE',  ( 1.000000000000000000, 0.000000000000000000, 0.000000000000000000 ) ) ;
#37174=AXIS2_PLACEMENT_3D ( 'NONE', #33397, #49487, #25686 ) ;
#37181=DIRECTION ( 'NONE',  ( -0.000000000000000000, -1.000000000000000000, -0.000000000000000000 ) ) ;
#37184=EDGE_LOOP ( 'NONE', ( #48850, #49696, #23006, #7523 ) ) ;
#37186=VECTOR ( 'NONE', #31149, 1000.000000000000000 ) ;
#37192=VERTEX_POINT ( 'NONE', #40630 ) ;
#37194=EDGE_CURVE ( 'NONE', #15096, #6217, #28821, .T. ) ;
#37199=EDGE_CURVE ( 'NONE', #34173, #15322, #5464, .T. ) ;
#37211=PLANE ( 'NONE',  #35820 ) ;
#37216=ORIENTED_EDGE ( 'NONE', *, *, #10202, .T. ) ;
#37219=ORIENTED_EDGE ( 'NONE', *, *, #50522, .F. ) ;
#37236=ORIENTED_EDGE ( 'NONE', *, *, #39456, .F. ) ;
#37246=EDGE_CURVE ( 'NONE', #33102, #45555, #1628, .T. ) ;
#37250=VECTOR ( 'NONE', #41520, 1000.000000000000000 ) ;
#37254=VERTEX_POINT ( 'NONE', #45188 ) ;
#37258=DIRECTION ( 'NONE',  ( -1.000000000000000000, 0.000000000000000000, -0.000000000000000000 ) ) ;
#37262=EDGE_CURVE ( 'NONE', #5959, #15096, #29075, .T. ) ;
#37270=DIRECTION ( 'NONE',  ( -0.000000000000000000, -1.000000000000000000, -0.000000000000000000 ) ) ;
#37279=DIRECTION ( 'NONE',  ( 1.000000000000000000, 0.000000000000000000, -0.000000000000000000 ) ) ;
#37280=VECTOR ( 'NONE', #29604, 1000.000000000000000 ) ;
#37283=ADVANCED_FACE ( 'NONE', ( #10569 ), #49526, .F. ) ;
#37291=LINE ( 'NONE', #3102, #29663 ) ;
#37298=DIRECTION ( 'NONE',  ( 0.000000000000000000, 0.000000000000000000, 1.000000000000000000 ) ) ;
#37302=ORIENTED_EDGE ( 'NONE', *, *, #42133, .F. ) ;
#37307=DIRECTION ( 'NONE',  ( 0.000000000000000000, 0.000000000000000000, 1.000000000000000000 ) ) ;
#37312=CARTESIAN_POINT ( 'NONE',  ( 80.00000000000122213, 16.00000000000000000, 5.000000000000004441 ) ) ;
#37323=EDGE_CURVE ( 'NONE', #35256, #36058, #15438, .T. ) ;
#37333=ADVANCED_FACE ( 'NONE', ( #50023 ), #23129, .F. ) ;
#37350=VECTOR ( 'NONE', #37101, 1000.000000000000000 ) ;
#37363=CARTESIAN_POINT ( 'NONE',  ( 85.00000000000056843, 16.00000000000000000, -30.00000000000000000 ) ) ;
#37365=PLANE ( 'NONE',  #10661 ) ;
#37367=ORIENTED_EDGE ( 'NONE', *, *, #32789, .T. ) ;
#37374=VECTOR ( 'NONE', #20905, 1000.000000000000000 ) ;
#37389=ORIENTED_EDGE ( 'NONE', *, *, #13260, .T. ) ;
#37391=CARTESIAN_POINT ( 'NONE',  ( -165.0000000000000284, 16.00000000000000000, 115.0000000000000142 ) ) ;
#37393=VERTEX_POINT ( 'NONE', #3118 ) ;
#37397=EDGE_CURVE ( 'NONE', #50570, #45549, #49774, .T. ) ;
#37399=LINE ( 'NONE', #33288, #22509 ) ;
#37403=CARTESIAN_POINT ( 'NONE',  ( 85.00000000000123634, 17.00000000000000000, 5.000000000000004441 ) ) ;
#37404=DIRECTION ( 'NONE',  ( -1.000000000000000000, -0.000000000000000000, -0.000000000000000000 ) ) ;
#37413=CARTESIAN_POINT ( 'NONE',  ( -69.99999999999816680, 17.00000000000000000, 65.00000000000000000 ) ) ;
#37417=CARTESIAN_POINT ( 'NONE',  ( -14.99999999999845812, 16.00000000000000000, 60.00000000000000000 ) ) ;
#37423=DIRECTION ( 'NONE',  ( -0.000000000000000000, -0.000000000000000000, -1.000000000000000000 ) ) ;
#37425=CARTESIAN_POINT ( 'NONE',  ( 85.00000000000152056, 17.00000000000000000, 35.00000000000000000 ) ) ;
#37427=DIRECTION ( 'NONE',  ( 0.000000000000000000, -0.000000000000000000, -1.000000000000000000 ) ) ;
#37439=LINE ( 'NONE', #48657, #21690 ) ;
#37444=ORIENTED_EDGE ( 'NONE', *, *, #15214, .F. ) ;
#37447=VERTEX_POINT ( 'NONE', #811 ) ;
#37448=CARTESIAN_POINT ( 'NONE',  ( -119.9999999999997158, 17.00000000000000000, -84.99999999999998579 ) ) ;
#37462=VERTEX_POINT ( 'NONE', #32361 ) ;
#37463=LINE ( 'NONE', #1289, #27581 ) ;
#37468=DIRECTION ( 'NONE',  ( -0.000000000000000000, -1.000000000000000000, -0.000000000000000000 ) ) ;
#37470=VERTEX_POINT ( 'NONE', #43891 ) ;
#37475=AXIS2_PLACEMENT_3D ( 'NONE', #30014, #9736, #41297 ) ;
#37483=VERTEX_POINT ( 'NONE', #20551 ) ;
#37489=DIRECTION ( 'NONE',  ( -3.469446951953611231E-16, -0.000000000000000000, -1.000000000000000000 ) ) ;
#37495=ADVANCED_FACE ( 'NONE', ( #24418 ), #36220, .F. ) ;
#37515=DIRECTION ( 'NONE',  ( -1.000000000000000000, 0.000000000000000000, 0.000000000000000000 ) ) ;
#37523=DIRECTION ( 'NONE',  ( -0.000000000000000000, -0.000000000000000000, -1.000000000000000000 ) ) ;
#37527=VERTEX_POINT ( 'NONE', #41060 ) ;
#37537=CARTESIAN_POINT ( 'NONE',  ( -119.9999999999994174, 16.00000000000000000, -54.99999999999999289 ) ) ;
#37539=LINE ( 'NONE', #33433, #29701 ) ;
#37540=EDGE_LOOP ( 'NONE', ( #34047, #7250, #9274, #32342 ) ) ;
#37546=EDGE_CURVE ( 'NONE', #42631, #44556, #14099, .T. ) ;
#37548=AXIS2_PLACEMENT_3D ( 'NONE', #12525, #29201, #20235 ) ;
#37564=LINE ( 'NONE', #48284, #27475 ) ;
#37565=EDGE_CURVE ( 'NONE', #8207, #45606, #49213, .T. ) ;
#37572=DIRECTION ( 'NONE',  ( -0.000000000000000000, -1.000000000000000000, -0.000000000000000000 ) ) ;
#37583=PLANE ( 'NONE',  #12470 ) ;
#37590=ORIENTED_EDGE ( 'NONE', *, *, #20285, .F. ) ;
#37595=DIRECTION ( 'NONE',  ( 0.000000000000000000, 0.000000000000000000, 1.000000000000000000 ) ) ;
#37599=LINE ( 'NONE', #18820, #14560 ) ;
#37604=CARTESIAN_POINT ( 'NONE',  ( 135.0000000000003411, 17.00000000000000000, -60.00000000000000000 ) ) ;
#37624=CARTESIAN_POINT ( 'NONE',  ( -19.99999999999940670, 17.00000000000000000, -30.00000000000000000 ) ) ;
#37628=CARTESIAN_POINT ( 'NONE',  ( -14.99999999999876366, 16.00000000000000000, 5.000000000000004441 ) ) ;
#37634=FACE_OUTER_BOUND ( 'NONE', #48434, .T. ) ;
#37637=CARTESIAN_POINT ( 'NONE',  ( 135.0000000000009663, 17.00000000000000000, 0.000000000000000000 ) ) ;
#37638=ORIENTED_EDGE ( 'NONE', *, *, #49676, .F. ) ;
#37665=CARTESIAN_POINT ( 'NONE',  ( 35.00000000000028422, 16.00000000000000000, -60.00000000000000000 ) ) ;
#37666=CARTESIAN_POINT ( 'NONE',  ( -64.99999999999877787, 17.00000000000000000, 5.000000000000004441 ) ) ;
#37670=VERTEX_POINT ( 'NONE', #34898 ) ;
#37673=VECTOR ( 'NONE', #47919, 1000.000000000000000 ) ;
#37676=ORIENTED_EDGE ( 'NONE', *, *, #45374, .F. ) ;
#37678=VECTOR ( 'NONE', #36682, 1000.000000000000000 ) ;
#37681=CARTESIAN_POINT ( 'NONE',  ( -19.99999999999971223, 16.00000000000000000, -84.99999999999998579 ) ) ;
#37682=CARTESIAN_POINT ( 'NONE',  ( -114.9999999999991047, 17.00000000000000000, -24.99999999999999289 ) ) ;
#37684=PLANE ( 'NONE',  #16797 ) ;
#37688=VERTEX_POINT ( 'NONE', #14361 ) ;
#37700=CARTESIAN_POINT ( 'NONE',  ( -165.0000000000000284, 16.00000000000000000, -54.99999999999999289 ) ) ;
#37701=CARTESIAN_POINT ( 'NONE',  ( 35.00000000000122213, 16.00000000000000000, 5.000000000000004441 ) ) ;
#37713=VECTOR ( 'NONE', #20065, 1000.000000000000000 ) ;
#37726=LINE ( 'NONE', #42055, #2698 ) ;
#37731=CARTESIAN_POINT ( 'NONE',  ( -119.9999999999978400, 16.00000000000000000, 95.00000000000000000 ) ) ;
#37747=DIRECTION ( 'NONE',  ( -0.000000000000000000, -1.000000000000000000, -0.000000000000000000 ) ) ;
#37761=CARTESIAN_POINT ( 'NONE',  ( 80.00000000000028422, 16.00000000000000000, -60.00000000000000000 ) ) ;
#37771=DIRECTION ( 'NONE',  ( 0.000000000000000000, 0.000000000000000000, -1.000000000000000000 ) ) ;
#37792=FACE_OUTER_BOUND ( 'NONE', #5169, .T. ) ;
#37803=CARTESIAN_POINT ( 'NONE',  ( 135.0000000000009663, 17.00000000000000000, 0.000000000000000000 ) ) ;
#37813=CARTESIAN_POINT ( 'NONE',  ( -14.99999999999812594, 17.00000000000000000, 65.00000000000000000 ) ) ;
#37815=ADVANCED_FACE ( 'NONE', ( #9387 ), #40697, .F. ) ;
#37818=ORIENTED_EDGE ( 'NONE', *, *, #26308, .T. ) ;
#37824=ORIENTED_EDGE ( 'NONE', *, *, #32920, .F. ) ;
#37825=CARTESIAN_POINT ( 'NONE',  ( -175.0000000000000000, 15.00000000000000000, 122.5000000000000142 ) ) ;
#37827=VECTOR ( 'NONE', #36670, 1000.000000000000000 ) ;
#37833=FACE_OUTER_BOUND ( 'NONE', #9228, .T. ) ;
#37834=DIRECTION ( 'NONE',  ( 1.000000000000000000, 0.000000000000000000, 0.000000000000000000 ) ) ;
#37835=ORIENTED_EDGE ( 'NONE', *, *, #3926, .F. ) ;
#37836=CARTESIAN_POINT ( 'NONE',  ( -14.99999999999876366, 16.00000000000000000, 5.000000000000004441 ) ) ;
#37841=EDGE_CURVE ( 'NONE', #13598, #30589, #8196, .T. ) ;
#37846=LINE ( 'NONE', #2416, #21859 ) ;
#37856=CARTESIAN_POINT ( 'NONE',  ( 164.9999999999999716, 17.00000000000000000, 65.00000000000000000 ) ) ;
#37859=DIRECTION ( 'NONE',  ( -0.000000000000000000, -1.000000000000000000, -0.000000000000000000 ) ) ;
#37870=EDGE_CURVE ( 'NONE', #13622, #45864, #13976, .T. ) ;
#37871=CARTESIAN_POINT ( 'NONE',  ( 0.000000000000000000, 17.00000000000000000, 0.000000000000000000 ) ) ;
#37876=DIRECTION ( 'NONE',  ( 0.000000000000000000, 0.000000000000000000, 1.000000000000000000 ) ) ;
#37881=ORIENTED_EDGE ( 'NONE', *, *, #27102, .F. ) ;
#37883=PLANE ( 'NONE',  #5382 ) ;
#37905=PLANE ( 'NONE',  #26343 ) ;
#37906=DIRECTION ( 'NONE',  ( -0.000000000000000000, -0.000000000000000000, -1.000000000000000000 ) ) ;
#37907=EDGE_LOOP ( 'NONE', ( #47896, #42913, #43008, #2183 ) ) ;
#37908=ORIENTED_EDGE ( 'NONE', *, *, #10848, .F. ) ;
#37920=DIRECTION ( 'NONE',  ( 0.000000000000000000, 0.000000000000000000, 1.000000000000000000 ) ) ;
#37921=VECTOR ( 'NONE', #49683, 1000.000000000000000 ) ;
#37933=EDGE_CURVE ( 'NONE', #47156, #44725, #2444, .T. ) ;
#37937=FACE_OUTER_BOUND ( 'NONE', #802, .T. ) ;
#37938=ORIENTED_EDGE ( 'NONE', *, *, #25555, .T. ) ;
#37940=FACE_OUTER_BOUND ( 'NONE', #37943, .T. ) ;
#37943=EDGE_LOOP ( 'NONE', ( #7711, #47549, #31694, #13794 ) ) ;
#37956=DIRECTION ( 'NONE',  ( -0.000000000000000000, -1.000000000000000000, -0.000000000000000000 ) ) ;
#37960=DIRECTION ( 'NONE',  ( 0.000000000000000000, 0.000000000000000000, 1.000000000000000000 ) ) ;
#37966=ORIENTED_EDGE ( 'NONE', *, *, #24902, .F. ) ;
#37970=LINE ( 'NONE', #14337, #48735 ) ;
#37975=LINE ( 'NONE', #2791, #27224 ) ;
#37981=DIRECTION ( 'NONE',  ( -0.000000000000000000, -1.000000000000000000, -0.000000000000000000 ) ) ;
#37984=CARTESIAN_POINT ( 'NONE',  ( -164.9999999999990905, 17.00000000000000000, -24.99999999999999289 ) ) ;
#37994=CARTESIAN_POINT ( 'NONE',  ( 80.00000000000153477, 17.00000000000000000, 35.00000000000000000 ) ) ;
#38004=VECTOR ( 'NONE', #35171, 1000.000000000000000 ) ;
#38012=EDGE_LOOP ( 'NONE', ( #43229, #47488, #44198, #26335 ) ) ;
#38025=VERTEX_POINT ( 'NONE', #50610 ) ;
#38027=DIRECTION ( 'NONE',  ( -0.000000000000000000, -1.000000000000000000, -0.000000000000000000 ) ) ;
#38042=CARTESIAN_POINT ( 'NONE',  ( 30.00000000000062172, 17.00000000000000000, -54.99999999999999289 ) ) ;
#38065=VECTOR ( 'NONE', #34226, 1000.000000000000000 ) ;
#38074=EDGE_CURVE ( 'NONE', #26042, #9263, #19604, .T. ) ;
#38082=CARTESIAN_POINT ( 'NONE',  ( 135.0000000000009663, 17.00000000000000000, 0.000000000000000000 ) ) ;
#38090=VERTEX_POINT ( 'NONE', #125 ) ;
#38100=PLANE ( 'NONE',  #43865 ) ;
#38103=PLANE ( 'NONE',  #30223 ) ;
#38119=EDGE_CURVE ( 'NONE', #42669, #41952, #38622, .T. ) ;
#38123=VECTOR ( 'NONE', #34268, 1000.000000000000000 ) ;
#38127=VECTOR ( 'NONE', #2504, 1000.000000000000000 ) ;
#38134=LINE ( 'NONE', #46023, #44701 ) ;
#38137=EDGE_CURVE ( 'NONE', #39319, #7126, #36554, .T. ) ;
#38155=LINE ( 'NONE', #7344, #8160 ) ;
#38166=VECTOR ( 'NONE', #5486, 1000.000000000000000 ) ;
#38172=VERTEX_POINT ( 'NONE', #44207 ) ;
#38191=VECTOR ( 'NONE', #13497, 1000.000000000000000 ) ;
#38192=EDGE_CURVE ( 'NONE', #970, #13545, #14435, .T. ) ;
#38196=LINE ( 'NONE', #34580, #32111 ) ;
#38210=VECTOR ( 'NONE', #46482, 1000.000000000000000 ) ;
#38218=CARTESIAN_POINT ( 'NONE',  ( -14.99999999999906919, 16.00000000000000000, -24.99999999999999289 ) ) ;
#38232=LINE ( 'NONE', #14593, #14275 ) ;
#38233=FACE_BOUND ( 'NONE', #10067, .T. ) ;
#38242=EDGE_CURVE ( 'NONE', #16517, #42175, #9330, .T. ) ;
#38259=VECTOR ( 'NONE', #33746, 1000.000000000000000 ) ;
#38262=LINE ( 'NONE', #33638, #30340 ) ;
#38276=ORIENTED_EDGE ( 'NONE', *, *, #7117, .F. ) ;
#38277=VERTEX_POINT ( 'NONE', #33448 ) ;
#38293=PLANE ( 'NONE',  #1707 ) ;
#38300=AXIS2_PLACEMENT_3D ( 'NONE', #47499, #39102, #38846 ) ;
#38301=EDGE_LOOP ( 'NONE', ( #1181, #45296, #12482, #785 ) ) ;
#38311=CARTESIAN_POINT ( 'NONE',  ( -19.99999999999878142, 17.00000000000000000, 5.000000000000004441 ) ) ;
#38319=FACE_OUTER_BOUND ( 'NONE', #25687, .T. ) ;
#38337=CARTESIAN_POINT ( 'NONE',  ( -114.9999999999984652, 16.00000000000000000, 60.00000000000000000 ) ) ;
#38339=LINE ( 'NONE', #7269, #36665 ) ;
#38342=LINE ( 'NONE', #35504, #1743 ) ;
#38351=PLANE ( 'NONE',  #48483 ) ;
#38352=ORIENTED_EDGE ( 'NONE', *, *, #26822, .F. ) ;
#38365=DIRECTION ( 'NONE',  ( 0.000000000000000000, 0.000000000000000000, 1.000000000000000000 ) ) ;
#38374=EDGE_CURVE ( 'NONE', #35246, #14478, #14942, .T. ) ;
#38386=ORIENTED_EDGE ( 'NONE', *, *, #20542, .T. ) ;
#38392=ORIENTED_EDGE ( 'NONE', *, *, #23811, .T. ) ;
#38401=EDGE_CURVE ( 'NONE', #31946, #21137, #28518, .T. ) ;
#38405=EDGE_LOOP ( 'NONE', ( #24009, #24459, #9963, #17996 ) ) ;
#38413=ORIENTED_EDGE ( 'NONE', *, *, #34684, .T. ) ;
#38416=CARTESIAN_POINT ( 'NONE',  ( -164.9999999999987779, 17.00000000000000000, 30.00000000000000000 ) ) ;
#38421=CARTESIAN_POINT ( 'NONE',  ( -114.9999999999997158, 16.00000000000000000, -84.99999999999998579 ) ) ;
#38429=ORIENTED_EDGE ( 'NONE', *, *, #24245, .T. ) ;
#38432=DIRECTION ( 'NONE',  ( -1.000000000000000000, -0.000000000000000000, -0.000000000000000000 ) ) ;
#38437=ORIENTED_EDGE ( 'NONE', *, *, #40619, .T. ) ;
#38440=LINE ( 'NONE', #2513, #46100 ) ;
#38443=LINE ( 'NONE', #14309, #19147 ) ;
#38453=LINE ( 'NONE', #6881, #2768 ) ;
#38463=PLANE ( 'NONE',  #3766 ) ;
#38465=EDGE_CURVE ( 'NONE', #42661, #29738, #32623, .T. ) ;
#38482=FACE_BOUND ( 'NONE', #26497, .T. ) ;
#38486=DIRECTION ( 'NONE',  ( -1.000000000000000000, 0.000000000000000000, -0.000000000000000000 ) ) ;
#38510=ORIENTED_EDGE ( 'NONE', *, *, #12381, .F. ) ;
#38514=DIRECTION ( 'NONE',  ( 1.000000000000000000, 0.000000000000000000, 0.000000000000000000 ) ) ;
#38517=CARTESIAN_POINT ( 'NONE',  ( -119.9999999999981668, 17.00000000000000000, 65.00000000000000000 ) ) ;
#38518=DIRECTION ( 'NONE',  ( 0.000000000000000000, 0.000000000000000000, 1.000000000000000000 ) ) ;
#38521=ORIENTED_EDGE ( 'NONE', *, *, #26308, .F. ) ;
#38523=VECTOR ( 'NONE', #15911, 1000.000000000000000 ) ;
#38527=VECTOR ( 'NONE', #42951, 1000.000000000000000 ) ;
#38541=CARTESIAN_POINT ( 'NONE',  ( 80.00000000000028422, 17.00000000000000000, -84.99999999999998579 ) ) ;
#38545=VERTEX_POINT ( 'NONE', #6172 ) ;
#38548=EDGE_CURVE ( 'NONE', #48491, #40717, #2074, .T. ) ;
#38549=DIRECTION ( 'NONE',  ( -0.000000000000000000, -1.000000000000000000, -0.000000000000000000 ) ) ;
#38550=VERTEX_POINT ( 'NONE', #5406 ) ;
#38553=CARTESIAN_POINT ( 'NONE',  ( -14.99999999999906919, 17.00000000000000000, -24.99999999999999289 ) ) ;
#38556=CARTESIAN_POINT ( 'NONE',  ( 135.0000000000006253, 17.00000000000000000, -54.99999999999999289 ) ) ;
#38562=AXIS2_PLACEMENT_3D ( 'NONE', #36646, #1471, #12752 ) ;
#38564=DIRECTION ( 'NONE',  ( -0.000000000000000000, -0.000000000000000000, -1.000000000000000000 ) ) ;
#38565=EDGE_LOOP ( 'NONE', ( #2319, #7742, #42840, #15776 ) ) ;
#38611=VERTEX_POINT ( 'NONE', #30795 ) ;
#38618=LINE ( 'NONE', #4657, #27327 ) ;
#38619=CARTESIAN_POINT ( 'NONE',  ( 135.0000000000019043, 17.00000000000000000, 65.00000000000000000 ) ) ;
#38622=LINE ( 'NONE', #889, #7564 ) ;
#38623=LINE ( 'NONE', #22696, #40929 ) ;
#38624=ORIENTED_EDGE ( 'NONE', *, *, #30533, .F. ) ;
#38635=ORIENTED_EDGE ( 'NONE', *, *, #44322, .F. ) ;
#38644=LINE ( 'NONE', #3202, #26724 ) ;
#38651=CARTESIAN_POINT ( 'NONE',  ( -64.99999999999940314, 16.00000000000000000, -54.99999999999999289 ) ) ;
#38654=ORIENTED_EDGE ( 'NONE', *, *, #48708, .F. ) ;
#38656=EDGE_CURVE ( 'NONE', #8813, #6749, #3065, .T. ) ;
#38658=VECTOR ( 'NONE', #11638, 1000.000000000000000 ) ;
#38670=DIRECTION ( 'NONE',  ( 1.000000000000000000, 0.000000000000000000, -2.312964634635843537E-16 ) ) ;
#38680=EDGE_CURVE ( 'NONE', #9263, #35257, #3317, .T. ) ;
#38682=EDGE_CURVE ( 'NONE', #40254, #37254, #18707, .T. ) ;
#38694=ORIENTED_EDGE ( 'NONE', *, *, #22763, .F. ) ;
#38697=ORIENTED_EDGE ( 'NONE', *, *, #8275, .F. ) ;
#38706=DIRECTION ( 'NONE',  ( -0.000000000000000000, -1.000000000000000000, -0.000000000000000000 ) ) ;
#38710=EDGE_CURVE ( 'NONE', #16028, #21378, #8716, .T. ) ;
#38723=FACE_BOUND ( 'NONE', #19668, .T. ) ;
#38730=PLANE ( 'NONE',  #47900 ) ;
#38733=FACE_OUTER_BOUND ( 'NONE', #41266, .T. ) ;
#38735=VECTOR ( 'NONE', #25474, 1000.000000000000000 ) ;
#38754=CARTESIAN_POINT ( 'NONE',  ( -14.99999999999970868, 17.00000000000000000, -84.99999999999998579 ) ) ;
#38765=LINE ( 'NONE', #38517, #845 ) ;
#38766=CARTESIAN_POINT ( 'NONE',  ( -64.99999999999940314, 17.00000000000000000, -54.99999999999999289 ) ) ;
#38767=VECTOR ( 'NONE', #32608, 1000.000000000000000 ) ;
#38769=ORIENTED_EDGE ( 'NONE', *, *, #44331, .T. ) ;
#38789=ORIENTED_EDGE ( 'NONE', *, *, #47177, .T. ) ;
#38803=DIRECTION ( 'NONE',  ( 0.000000000000000000, 0.000000000000000000, -1.000000000000000000 ) ) ;
#38804=VERTEX_POINT ( 'NONE', #31813 ) ;
#38805=LINE ( 'NONE', #50281, #13254 ) ;
#38813=EDGE_CURVE ( 'NONE', #18558, #3258, #29455, .T. ) ;
#38814=ORIENTED_EDGE ( 'NONE', *, *, #21249, .F. ) ;
#38818=CARTESIAN_POINT ( 'NONE',  ( 79.99999999999997158, 16.00000000000000000, -90.00000000000000000 ) ) ;
#38820=EDGE_CURVE ( 'NONE', #4352, #29552, #21251, .T. ) ;
#38821=LINE ( 'NONE', #4167, #43563 ) ;
#38832=LINE ( 'NONE', #33955, #2112 ) ;
#38833=ADVANCED_FACE ( 'NONE', ( #13787 ), #40509, .F. ) ;
#38839=ORIENTED_EDGE ( 'NONE', *, *, #49621, .F. ) ;
#38843=VECTOR ( 'NONE', #27773, 1000.000000000000000 ) ;
#38846=DIRECTION ( 'NONE',  ( 0.000000000000000000, -0.000000000000000000, -1.000000000000000000 ) ) ;
#38859=DIRECTION ( 'NONE',  ( 0.000000000000000000, 0.000000000000000000, -1.000000000000000000 ) ) ;
#38860=VERTEX_POINT ( 'NONE', #25111 ) ;
#38869=DIRECTION ( 'NONE',  ( -0.000000000000000000, -0.000000000000000000, -1.000000000000000000 ) ) ;
#38878=EDGE_CURVE ( 'NONE', #26946, #8841, #17890, .T. ) ;
#38880=VECTOR ( 'NONE', #1964, 1000.000000000000000 ) ;
#38898=VECTOR ( 'NONE', #3630, 1000.000000000000000 ) ;
#38899=ORIENTED_EDGE ( 'NONE', *, *, #39100, .F. ) ;
#38900=EDGE_LOOP ( 'NONE', ( #47217, #37818, #22928, #12115 ) ) ;
#38913=EDGE_LOOP ( 'NONE', ( #48029, #35249, #22273, #41467 ) ) ;
#38946=DIRECTION ( 'NONE',  ( 1.000000000000000000, 0.000000000000000000, 0.000000000000000000 ) ) ;
#38963=CARTESIAN_POINT ( 'NONE',  ( -114.9999999999984652, 17.00000000000000000, 60.00000000000000000 ) ) ;
#38967=FACE_OUTER_BOUND ( 'NONE', #8055, .T. ) ;
#38971=VECTOR ( 'NONE', #37181, 1000.000000000000000 ) ;
#38974=CARTESIAN_POINT ( 'NONE',  ( 35.00000000000091660, 17.00000000000000000, -24.99999999999999289 ) ) ;
#38975=VECTOR ( 'NONE', #50530, 1000.000000000000000 ) ;
#38980=DIRECTION ( 'NONE',  ( -1.000000000000000000, -0.000000000000000000, -0.000000000000000000 ) ) ;
#38993=CARTESIAN_POINT ( 'NONE',  ( 130.0000000000018474, 17.00000000000000000, 90.00000000000000000 ) ) ;
#39006=EDGE_CURVE ( 'NONE', #24564, #32291, #41509, .T. ) ;
#39009=ORIENTED_EDGE ( 'NONE', *, *, #10322, .F. ) ;
#39013=ORIENTED_EDGE ( 'NONE', *, *, #35715, .F. ) ;
#39021=LINE ( 'NONE', #529, #6031 ) ;
#39023=ORIENTED_EDGE ( 'NONE', *, *, #30614, .F. ) ;
#39034=VERTEX_POINT ( 'NONE', #26101 ) ;
#39041=DIRECTION ( 'NONE',  ( 0.000000000000000000, -0.000000000000000000, -1.000000000000000000 ) ) ;
#39058=AXIS2_PLACEMENT_3D ( 'NONE', #42978, #47050, #42467 ) ;
#39080=CARTESIAN_POINT ( 'NONE',  ( 80.00000000000061107, 17.00000000000000000, -54.99999999999999289 ) ) ;
#39083=ORIENTED_EDGE ( 'NONE', *, *, #794, .F. ) ;
#39087=ORIENTED_EDGE ( 'NONE', *, *, #6541, .T. ) ;
#39093=EDGE_LOOP ( 'NONE', ( #21341, #46503, #1421, #13797 ) ) ;
#39100=EDGE_CURVE ( 'NONE', #12877, #19097, #442, .T. ) ;
#39102=DIRECTION ( 'NONE',  ( 0.000000000000000000, -1.000000000000000000, 0.000000000000000000 ) ) ;
#39103=EDGE_LOOP ( 'NONE', ( #46191, #14918, #23403, #33660 ) ) ;
#39106=CARTESIAN_POINT ( 'NONE',  ( 130.0000000000021032, 17.00000000000000000, 95.00000000000000000 ) ) ;
#39111=ORIENTED_EDGE ( 'NONE', *, *, #47512, .F. ) ;
#39113=DIRECTION ( 'NONE',  ( 0.000000000000000000, 0.000000000000000000, 1.000000000000000000 ) ) ;
#39116=ORIENTED_EDGE ( 'NONE', *, *, #13150, .F. ) ;
#39122=EDGE_CURVE ( 'NONE', #24991, #2139, #27894, .T. ) ;
#39126=VECTOR ( 'NONE', #7594, 1000.000000000000000 ) ;
#39132=FACE_OUTER_BOUND ( 'NONE', #24271, .T. ) ;
#39147=CARTESIAN_POINT ( 'NONE',  ( -69.99999999999940314, 16.00000000000000000, -54.99999999999999289 ) ) ;
#39153=DIRECTION ( 'NONE',  ( 0.000000000000000000, 0.000000000000000000, -1.000000000000000000 ) ) ;
#39154=FACE_OUTER_BOUND ( 'NONE', #23504, .T. ) ;
#39155=ORIENTED_EDGE ( 'NONE', *, *, #26229, .T. ) ;
#39169=CARTESIAN_POINT ( 'NONE',  ( -164.9999999999984936, 17.00000000000000000, 35.00000000000000000 ) ) ;
#39178=VERTEX_POINT ( 'NONE', #21436 ) ;
#39181=CARTESIAN_POINT ( 'NONE',  ( -119.9999999999987921, 16.00000000000000000, 5.000000000000004441 ) ) ;
#39182=DIRECTION ( 'NONE',  ( -1.000000000000000000, -0.000000000000000000, -0.000000000000000000 ) ) ;
#39187=EDGE_CURVE ( 'NONE', #15972, #15720, #36878, .T. ) ;
#39188=CARTESIAN_POINT ( 'NONE',  ( 164.9999999999999716, 16.00000000000000000, 5.000000000000004441 ) ) ;
#39194=DIRECTION ( 'NONE',  ( 1.000000000000000000, 0.000000000000000000, 0.000000000000000000 ) ) ;
#39199=PLANE ( 'NONE',  #45004 ) ;
#39210=VERTEX_POINT ( 'NONE', #11864 ) ;
#39240=ADVANCED_FACE ( 'NONE', ( #34014 ), #17843, .F. ) ;
#39246=CARTESIAN_POINT ( 'NONE',  ( -119.9999999999987921, 16.00000000000000000, 5.000000000000004441 ) ) ;
#39251=LINE ( 'NONE', #4093, #23838 ) ;
#39259=ORIENTED_EDGE ( 'NONE', *, *, #17496, .T. ) ;
#39260=VECTOR ( 'NONE', #49189, 1000.000000000000000 ) ;
#39268=AXIS2_PLACEMENT_3D ( 'NONE', #6185, #18217, #49232 ) ;
#39269=VERTEX_POINT ( 'NONE', #6802 ) ;
#39270=CARTESIAN_POINT ( 'NONE',  ( -14.99999999999812594, 16.00000000000000000, 65.00000000000000000 ) ) ;
#39271=CARTESIAN_POINT ( 'NONE',  ( -119.9999999999997158, 17.00000000000000000, -84.99999999999998579 ) ) ;
#39273=DIRECTION ( 'NONE',  ( -0.000000000000000000, -1.000000000000000000, -0.000000000000000000 ) ) ;
#39284=VERTEX_POINT ( 'NONE', #45265 ) ;
#39288=CARTESIAN_POINT ( 'NONE',  ( -69.99999999999816680, 16.00000000000000000, 65.00000000000000000 ) ) ;
#39311=DIRECTION ( 'NONE',  ( 0.000000000000000000, 0.000000000000000000, 1.000000000000000000 ) ) ;
#39319=VERTEX_POINT ( 'NONE', #37624 ) ;
#39326=VERTEX_POINT ( 'NONE', #24180 ) ;
#39331=CARTESIAN_POINT ( 'NONE',  ( 85.00000000000029843, 17.00000000000000000, -60.00000000000000000 ) ) ;
#39342=PLANE ( 'NONE',  #2951 ) ;
#39361=EDGE_CURVE ( 'NONE', #35762, #15096, #4672, .T. ) ;
#39365=VECTOR ( 'NONE', #6122, 1000.000000000000000 ) ;
#39374=PLANE ( 'NONE',  #43228 ) ;
#39376=VECTOR ( 'NONE', #11151, 1000.000000000000000 ) ;
#39382=VECTOR ( 'NONE', #21468, 1000.000000000000000 ) ;
#39395=EDGE_CURVE ( 'NONE', #39034, #7468, #8271, .T. ) ;
#39396=EDGE_CURVE ( 'NONE', #38090, #49813, #826, .T. ) ;
#39404=DIRECTION ( 'NONE',  ( 0.000000000000000000, -0.000000000000000000, -1.000000000000000000 ) ) ;
#39405=EDGE_CURVE ( 'NONE', #36736, #23599, #47720, .T. ) ;
#39409=ORIENTED_EDGE ( 'NONE', *, *, #25215, .T. ) ;
#39423=VERTEX_POINT ( 'NONE', #1829 ) ;
#39428=EDGE_LOOP ( 'NONE', ( #46732, #221, #44838, #28653 ) ) ;
#39435=FACE_OUTER_BOUND ( 'NONE', #30383, .T. ) ;
#39437=ORIENTED_EDGE ( 'NONE', *, *, #6631, .F. ) ;
#39446=CARTESIAN_POINT ( 'NONE',  ( 164.9999999999999716, 16.00000000000000000, 115.0000000000000142 ) ) ;
#39449=ADVANCED_FACE ( 'NONE', ( #45649 ), #13621, .F. ) ;
#39453=CARTESIAN_POINT ( 'NONE',  ( 80.00000000000186162, 17.00000000000000000, 65.00000000000000000 ) ) ;
#39456=EDGE_CURVE ( 'NONE', #43496, #30589, #10029, .T. ) ;
#39459=ORIENTED_EDGE ( 'NONE', *, *, #31562, .F. ) ;
#39460=ORIENTED_EDGE ( 'NONE', *, *, #22357, .T. ) ;
#39461=CARTESIAN_POINT ( 'NONE',  ( 85.00000000000029843, 16.00000000000000000, -84.99999999999998579 ) ) ;
#39467=DIRECTION ( 'NONE',  ( 0.000000000000000000, 0.000000000000000000, -1.000000000000000000 ) ) ;
#39479=MANIFOLD_SOLID_BREP ( 'Boss-Extrude3', #45729 ) ;
#39483=DIRECTION ( 'NONE',  ( 0.000000000000000000, 0.000000000000000000, 1.000000000000000000 ) ) ;
#39486=EDGE_LOOP ( 'NONE', ( #41214, #47672, #32785, #44145 ) ) ;
#39488=DIRECTION ( 'NONE',  ( -0.000000000000000000, -1.000000000000000000, -0.000000000000000000 ) ) ;
#39504=CARTESIAN_POINT ( 'NONE',  ( -164.9999999999984936, 17.00000000000000000, 60.00000000000000000 ) ) ;
#39505=AXIS2_PLACEMENT_3D ( 'NONE', #45422, #5695, #45168 ) ;
#39506=CARTESIAN_POINT ( 'NONE',  ( 130.0000000000012221, 17.00000000000000000, 5.000000000000004441 ) ) ;
#39510=ORIENTED_EDGE ( 'NONE', *, *, #19266, .T. ) ;
#39516=DIRECTION ( 'NONE',  ( -0.000000000000000000, -1.000000000000000000, -0.000000000000000000 ) ) ;
#39519=EDGE_LOOP ( 'NONE', ( #4520, #20717, #12152, #33620 ) ) ;
#39526=ORIENTED_EDGE ( 'NONE', *, *, #23807, .T. ) ;
#39534=DIRECTION ( 'NONE',  ( -0.000000000000000000, -1.000000000000000000, -0.000000000000000000 ) ) ;
#39535=ORIENTED_EDGE ( 'NONE', *, *, #7117, .T. ) ;
#39537=DIRECTION ( 'NONE',  ( -1.000000000000000000, 0.000000000000000000, 0.000000000000000000 ) ) ;
#39553=CARTESIAN_POINT ( 'NONE',  ( 164.9999999999999716, 17.00000000000000000, 95.00000000000000000 ) ) ;
#39564=CARTESIAN_POINT ( 'NONE',  ( -114.9999999999984652, 16.00000000000000000, 60.00000000000000000 ) ) ;
#39573=ORIENTED_EDGE ( 'NONE', *, *, #35644, .T. ) ;
#39575=VECTOR ( 'NONE', #41745, 1000.000000000000000 ) ;
#39576=DIRECTION ( 'NONE',  ( 1.000000000000000000, 0.000000000000000000, 0.000000000000000000 ) ) ;
#39588=FACE_OUTER_BOUND ( 'NONE', #6668, .T. ) ;
#39589=EDGE_CURVE ( 'NONE', #13970, #22765, #18978, .T. ) ;
#39601=LINE ( 'NONE', #36265, #19359 ) ;
#39613=EDGE_CURVE ( 'NONE', #34689, #20602, #50492, .T. ) ;
#39614=ORIENTED_EDGE ( 'NONE', *, *, #9676, .T. ) ;
#39618=CARTESIAN_POINT ( 'NONE',  ( -114.9999999999987779, 17.00000000000000000, 5.000000000000004441 ) ) ;
#39638=VECTOR ( 'NONE', #9463, 1000.000000000000000 ) ;
#39658=ORIENTED_EDGE ( 'NONE', *, *, #23850, .T. ) ;
#39659=VERTEX_POINT ( 'NONE', #28215 ) ;
#39664=ORIENTED_EDGE ( 'NONE', *, *, #27088, .T. ) ;
#39670=VERTEX_POINT ( 'NONE', #27705 ) ;
#39680=DIRECTION ( 'NONE',  ( 0.000000000000000000, 0.000000000000000000, -1.000000000000000000 ) ) ;
#39683=LINE ( 'NONE', #34830, #46199 ) ;
#39698=EDGE_LOOP ( 'NONE', ( #36691, #10129, #44869, #30656 ) ) ;
#39705=DIRECTION ( 'NONE',  ( -1.000000000000000000, 0.000000000000000000, 0.000000000000000000 ) ) ;
#39707=CARTESIAN_POINT ( 'NONE',  ( 164.9999999999999716, 17.00000000000000000, -85.00000000000001421 ) ) ;
#39713=CARTESIAN_POINT ( 'NONE',  ( 30.00000000000153833, 17.00000000000000000, 35.00000000000000000 ) ) ;
#39737=CARTESIAN_POINT ( 'NONE',  ( -19.99999999999846523, 17.00000000000000000, 35.00000000000000000 ) ) ;
#39738=DIRECTION ( 'NONE',  ( -0.000000000000000000, -1.000000000000000000, -0.000000000000000000 ) ) ;
#39743=EDGE_CURVE ( 'NONE', #24017, #28153, #2516, .T. ) ;
#39745=PLANE ( 'NONE',  #42296 ) ;
#39747=ADVANCED_FACE ( 'NONE', ( #9707 ), #6363, .F. ) ;
#39748=FACE_OUTER_BOUND ( 'NONE', #41479, .T. ) ;
#39751=EDGE_CURVE ( 'NONE', #41862, #17026, #21766, .T. ) ;
#39776=APPLICATION_CONTEXT ( 'automotive_design' ) ;
#39777=ORIENTED_EDGE ( 'NONE', *, *, #20330, .F. ) ;
#39780=DIRECTION ( 'NONE',  ( -1.000000000000000000, -0.000000000000000000, -0.000000000000000000 ) ) ;
#39782=DIRECTION ( 'NONE',  ( 0.000000000000000000, 0.000000000000000000, 1.000000000000000000 ) ) ;
#39804=LINE ( 'NONE', #4876, #16080 ) ;
#39812=DIRECTION ( 'NONE',  ( -1.000000000000000000, 0.000000000000000000, -0.000000000000000000 ) ) ;
#39822=DIRECTION ( 'NONE',  ( 2.312964634635864737E-16, -0.000000000000000000, 1.000000000000000000 ) ) ;
#39828=AXIS2_PLACEMENT_3D ( 'NONE', #43888, #27992, #24162 ) ;
#39843=DIRECTION ( 'NONE',  ( -1.000000000000000000, 0.000000000000000000, 0.000000000000000000 ) ) ;
#39845=ORIENTED_EDGE ( 'NONE', *, *, #17586, .F. ) ;
#39876=AXIS2_PLACEMENT_3D ( 'NONE', #1593, #25188, #40833 ) ;
#39880=DIRECTION ( 'NONE',  ( 1.000000000000000000, 0.000000000000000000, 0.000000000000000000 ) ) ;
#39883=PLANE ( 'NONE',  #32421 ) ;
#39907=VECTOR ( 'NONE', #7020, 1000.000000000000000 ) ;
#39912=CARTESIAN_POINT ( 'NONE',  ( 30.00000000000029132, 16.00000000000000000, -84.99999999999998579 ) ) ;
#39916=DIRECTION ( 'NONE',  ( 0.000000000000000000, 0.000000000000000000, -1.000000000000000000 ) ) ;
#39921=VECTOR ( 'NONE', #1014, 1000.000000000000000 ) ;
#39924=ORIENTED_EDGE ( 'NONE', *, *, #21834, .F. ) ;
#39931=CARTESIAN_POINT ( 'NONE',  ( -70.00000000000002842, 17.00000000000000000, -114.9999999999999858 ) ) ;
#39933=PLANE ( 'NONE',  #28919 ) ;
#39935=DIRECTION ( 'NONE',  ( -1.000000000000000000, 0.000000000000000000, -0.000000000000000000 ) ) ;
#39938=EDGE_CURVE ( 'NONE', #9083, #34191, #38443, .T. ) ;
#39948=DIRECTION ( 'NONE',  ( -0.000000000000000000, -1.000000000000000000, -0.000000000000000000 ) ) ;
#39949=DIRECTION ( 'NONE',  ( 1.000000000000000000, 0.000000000000000000, 0.000000000000000000 ) ) ;
#39952=VECTOR ( 'NONE', #8463, 1000.000000000000000 ) ;
#39955=FACE_OUTER_BOUND ( 'NONE', #4142, .T. ) ;
#39970=LINE ( 'NONE', #48610, #18017 ) ;
#39977=CARTESIAN_POINT ( 'NONE',  ( 80.00000000000061107, 17.00000000000000000, -30.00000000000000000 ) ) ;
#39984=EDGE_LOOP ( 'NONE', ( #14392, #14884, #6801, #27264 ) ) ;
#40006=CARTESIAN_POINT ( 'NONE',  ( 0.000000000000000000, 17.00000000000000000, 0.000000000000000000 ) ) ;
#40010=DIRECTION ( 'NONE',  ( -0.000000000000000000, -0.000000000000000000, 1.000000000000000000 ) ) ;
#40039=ORIENTED_EDGE ( 'NONE', *, *, #31177, .T. ) ;
#40043=PLANE ( 'NONE',  #19649 ) ;
#40052=ORIENTED_EDGE ( 'NONE', *, *, #2256, .F. ) ;
#40053=PLANE ( 'NONE',  #19570 ) ;
#40054=FACE_OUTER_BOUND ( 'NONE', #28110, .T. ) ;
#40061=AXIS2_PLACEMENT_3D ( 'NONE', #42185, #38365, #34777 ) ;
#40063=DIRECTION ( 'NONE',  ( -0.000000000000000000, -1.000000000000000000, -0.000000000000000000 ) ) ;
#40065=ORIENTED_EDGE ( 'NONE', *, *, #46921, .T. ) ;
#40073=VERTEX_POINT ( 'NONE', #5547 ) ;
#40077=CARTESIAN_POINT ( 'NONE',  ( 84.99999999999997158, 17.00000000000000000, -114.9999999999999858 ) ) ;
#40079=DIRECTION ( 'NONE',  ( 1.000000000000000000, 0.000000000000000000, -4.625929269271542120E-16 ) ) ;
#40080=ORIENTED_EDGE ( 'NONE', *, *, #12422, .T. ) ;
#40085=ORIENTED_EDGE ( 'NONE', *, *, #48076, .F. ) ;
#40097=AXIS2_PLACEMENT_3D ( 'NONE', #27999, #27504, #39311 ) ;
#40100=LINE ( 'NONE', #848, #34951 ) ;
#40103=CARTESIAN_POINT ( 'NONE',  ( 30.00000000000029132, 17.00000000000000000, -84.99999999999998579 ) ) ;
#40105=VECTOR ( 'NONE', #4345, 1000.000000000000000 ) ;
#40116=FACE_OUTER_BOUND ( 'NONE', #25834, .T. ) ;
#40132=ADVANCED_FACE ( 'NONE', ( #34288 ), #35325, .F. ) ;
#40133=VECTOR ( 'NONE', #2009, 1000.000000000000000 ) ;
#40139=VECTOR ( 'NONE', #37523, 1000.000000000000000 ) ;
#40153=DIRECTION ( 'NONE',  ( 1.000000000000000000, 0.000000000000000000, 0.000000000000000000 ) ) ;
#40163=VECTOR ( 'NONE', #33264, 1000.000000000000000 ) ;
#40167=VECTOR ( 'NONE', #37468, 1000.000000000000000 ) ;
#40171=ORIENTED_EDGE ( 'NONE', *, *, #50589, .F. ) ;
#40175=ORIENTED_EDGE ( 'NONE', *, *, #16501, .T. ) ;
#40176=AXIS2_PLACEMENT_3D ( 'NONE', #50047, #43171, #15456 ) ;
#40185=EDGE_CURVE ( 'NONE', #27664, #13545, #42470, .T. ) ;
#40190=VECTOR ( 'NONE', #36952, 1000.000000000000000 ) ;
#40199=CARTESIAN_POINT ( 'NONE',  ( 30.00000000000029132, 17.00000000000000000, -60.00000000000000000 ) ) ;
#40200=ORIENTED_EDGE ( 'NONE', *, *, #8710, .T. ) ;
#40202=VECTOR ( 'NONE', #13285, 1000.000000000000000 ) ;
#40226=DIRECTION ( 'NONE',  ( -0.000000000000000000, -1.000000000000000000, -0.000000000000000000 ) ) ;
#40232=EDGE_CURVE ( 'NONE', #13622, #25002, #46040, .T. ) ;
#40236=CARTESIAN_POINT ( 'NONE',  ( -19.99999999999846523, 16.00000000000000000, 60.00000000000000000 ) ) ;
#40248=VERTEX_POINT ( 'NONE', #44912 ) ;
#40251=CARTESIAN_POINT ( 'NONE',  ( -14.99999999999782041, 17.00000000000000000, 115.0000000000000142 ) ) ;
#40252=DIRECTION ( 'NONE',  ( 0.000000000000000000, 0.000000000000000000, -1.000000000000000000 ) ) ;
#40254=VERTEX_POINT ( 'NONE', #47998 ) ;
#40259=CARTESIAN_POINT ( 'NONE',  ( 35.00000000000186162, 16.00000000000000000, 65.00000000000000000 ) ) ;
#40260=CARTESIAN_POINT ( 'NONE',  ( 35.00000000000122213, 16.00000000000000000, 5.000000000000004441 ) ) ;
#40271=LINE ( 'NONE', #13557, #37673 ) ;
#40280=LINE ( 'NONE', #1027, #24344 ) ;
#40297=VECTOR ( 'NONE', #33880, 1000.000000000000000 ) ;
#40303=SHAPE_DEFINITION_REPRESENTATION ( #34362, #8742 ) ;
#40311=ORIENTED_EDGE ( 'NONE', *, *, #24387, .T. ) ;
#40312=EDGE_CURVE ( 'NONE', #42092, #24012, #21595, .T. ) ;
#40313=CARTESIAN_POINT ( 'NONE',  ( 30.00000000000153833, 17.00000000000000000, 35.00000000000000000 ) ) ;
#40326=DIRECTION ( 'NONE',  ( -0.000000000000000000, -0.000000000000000000, -1.000000000000000000 ) ) ;
#40328=ADVANCED_FACE ( 'NONE', ( #48251 ), #33175, .F. ) ;
#40345=FACE_OUTER_BOUND ( 'NONE', #33650, .T. ) ;
#40355=DIRECTION ( 'NONE',  ( 0.000000000000000000, 0.000000000000000000, 1.000000000000000000 ) ) ;
#40369=SHAPE_REPRESENTATION_RELATIONSHIP ( 'NONE' , 'NONE' ,  #8742, #33210 ) ;
#40381=AXIS2_PLACEMENT_3D ( 'NONE', #43684, #16253, #35785 ) ;
#40419=CARTESIAN_POINT ( 'NONE',  ( 135.0000000000003411, 16.00000000000000000, -84.99999999999998579 ) ) ;
#40420=CARTESIAN_POINT ( 'NONE',  ( 85.00000000000152056, 17.00000000000000000, 60.00000000000000000 ) ) ;
#40428=DIRECTION ( 'NONE',  ( 0.000000000000000000, 0.000000000000000000, -1.000000000000000000 ) ) ;
#40432=DIRECTION ( 'NONE',  ( -0.000000000000000000, -0.000000000000000000, -1.000000000000000000 ) ) ;
#40433=FACE_OUTER_BOUND ( 'NONE', #50637, .T. ) ;
#40442=EDGE_CURVE ( 'NONE', #22825, #43501, #35452, .T. ) ;
#40443=VECTOR ( 'NONE', #46720, 1000.000000000000000 ) ;
#40444=ADVANCED_FACE ( 'NONE', ( #23374 ), #34947, .F. ) ;
#40450=ORIENTED_EDGE ( 'NONE', *, *, #45303, .T. ) ;
#40455=LINE ( 'NONE', #28897, #15559 ) ;
#40463=DIRECTION ( 'NONE',  ( -1.000000000000000000, 0.000000000000000000, 0.000000000000000000 ) ) ;
#40477=FACE_OUTER_BOUND ( 'NONE', #34392, .T. ) ;
#40478=CARTESIAN_POINT ( 'NONE',  ( -69.99999999999879208, 17.00000000000000000, 5.000000000000004441 ) ) ;
#40481=EDGE_LOOP ( 'NONE', ( #2011, #28522, #21875, #9048 ) ) ;
#40484=VECTOR ( 'NONE', #42812, 1000.000000000000000 ) ;
#40489=VECTOR ( 'NONE', #24593, 1000.000000000000000 ) ;
#40495=CARTESIAN_POINT ( 'NONE',  ( 35.00000000000122213, 17.00000000000000000, 30.00000000000000000 ) ) ;
#40498=LINE ( 'NONE', #27684, #40489 ) ;
#40501=DIRECTION ( 'NONE',  ( -1.000000000000000000, 0.000000000000000000, 0.000000000000000000 ) ) ;
#40504=LINE ( 'NONE', #28198, #27830 ) ;
#40507=CARTESIAN_POINT ( 'NONE',  ( -165.0000000000000284, 16.00000000000000000, 115.0000000000000142 ) ) ;
#40508=ORIENTED_EDGE ( 'NONE', *, *, #6454, .F. ) ;
#40509=PLANE ( 'NONE',  #26487 ) ;
#40517=VERTEX_POINT ( 'NONE', #11577 ) ;
#40518=DIRECTION ( 'NONE',  ( 0.000000000000000000, 0.000000000000000000, -1.000000000000000000 ) ) ;
#40524=ORIENTED_EDGE ( 'NONE', *, *, #38465, .T. ) ;
#40529=ORIENTED_EDGE ( 'NONE', *, *, #47320, .T. ) ;
#40530=PLANE ( 'NONE',  #24787 ) ;
#40531=VECTOR ( 'NONE', #34249, 1000.000000000000000 ) ;
#40535=VERTEX_POINT ( 'NONE', #27231 ) ;
#40540=LINE ( 'NONE', #8985, #35703 ) ;
#40542=FACE_OUTER_BOUND ( 'NONE', #39984, .T. ) ;
#40546=PLANE ( 'NONE',  #18755 ) ;
#40549=EDGE_LOOP ( 'NONE', ( #517, #11112, #26747, #26055 ) ) ;
#40557=LINE ( 'NONE', #33625, #1945 ) ;
#40564=PLANE ( 'NONE',  #404 ) ;
#40565=EDGE_CURVE ( 'NONE', #12877, #35256, #31603, .T. ) ;
#40567=EDGE_CURVE ( 'NONE', #45555, #49766, #43363, .T. ) ;
#40570=CARTESIAN_POINT ( 'NONE',  ( -70.00000000000002842, 16.00000000000000000, -114.9999999999999858 ) ) ;
#40575=DIRECTION ( 'NONE',  ( 0.000000000000000000, 0.000000000000000000, -1.000000000000000000 ) ) ;
#40581=CARTESIAN_POINT ( 'NONE',  ( -64.99999999999971578, 17.00000000000000000, -60.00000000000000000 ) ) ;
#40583=CARTESIAN_POINT ( 'NONE',  ( 85.00000000000213163, 16.00000000000000000, 95.00000000000000000 ) ) ;
#40591=CARTESIAN_POINT ( 'NONE',  ( 130.0000000000002842, 17.00000000000000000, -60.00000000000000000 ) ) ;
#40597=DIRECTION ( 'NONE',  ( 0.000000000000000000, 0.000000000000000000, 1.000000000000000000 ) ) ;
#40609=ORIENTED_EDGE ( 'NONE', *, *, #14833, .F. ) ;
#40615=FACE_OUTER_BOUND ( 'NONE', #5938, .T. ) ;
#40619=EDGE_CURVE ( 'NONE', #31669, #614, #21535, .T. ) ;
#40624=DIRECTION ( 'NONE',  ( 0.000000000000000000, 0.000000000000000000, 1.000000000000000000 ) ) ;
#40625=LINE ( 'NONE', #5461, #41412 ) ;
#40627=ADVANCED_FACE ( 'NONE', ( #40542 ), #21287, .F. ) ;
#40630=CARTESIAN_POINT ( 'NONE',  ( -64.99999999999877787, 17.00000000000000000, 30.00000000000000000 ) ) ;
#40633=DIRECTION ( 'NONE',  ( 1.000000000000000000, 0.000000000000000000, 0.000000000000000000 ) ) ;
#40635=VECTOR ( 'NONE', #38670, 1000.000000000000000 ) ;
#40652=LINE ( 'NONE', #33712, #38166 ) ;
#40663=DIRECTION ( 'NONE',  ( 1.000000000000000000, 0.000000000000000000, 0.000000000000000000 ) ) ;
#40666=AXIS2_PLACEMENT_3D ( 'NONE', #25716, #1616, #1866 ) ;
#40667=ORIENTED_EDGE ( 'NONE', *, *, #31937, .T. ) ;
#40671=EDGE_CURVE ( 'NONE', #22825, #41411, #38232, .T. ) ;
#40672=DIRECTION ( 'NONE',  ( 0.000000000000000000, 0.000000000000000000, 1.000000000000000000 ) ) ;
#40683=LINE ( 'NONE', #31794, #37350 ) ;
#40697=PLANE ( 'NONE',  #32217 ) ;
#40708=DIRECTION ( 'NONE',  ( -1.000000000000000000, 0.000000000000000000, 0.000000000000000000 ) ) ;
#40717=VERTEX_POINT ( 'NONE', #29495 ) ;
#40721=EDGE_LOOP ( 'NONE', ( #20073, #45178, #47627, #44224 ) ) ;
#40733=ORIENTED_EDGE ( 'NONE', *, *, #28674, .T. ) ;
#40737=ORIENTED_EDGE ( 'NONE', *, *, #22880, .T. ) ;
#40746=FACE_OUTER_BOUND ( 'NONE', #44088, .T. ) ;
#40747=LINE ( 'NONE', #5334, #2872 ) ;
#40750=PLANE ( 'NONE',  #20597 ) ;
#40752=DIRECTION ( 'NONE',  ( -0.000000000000000000, -1.000000000000000000, -0.000000000000000000 ) ) ;
#40754=CARTESIAN_POINT ( 'NONE',  ( -175.0000000000000000, 15.00000000000000000, 122.5000000000000142 ) ) ;
#40760=DIRECTION ( 'NONE',  ( -1.000000000000000000, -0.000000000000000000, -0.000000000000000000 ) ) ;
#40766=VERTEX_POINT ( 'NONE', #10497 ) ;
#40771=ORIENTED_EDGE ( 'NONE', *, *, #11414, .F. ) ;
#40772=CARTESIAN_POINT ( 'NONE',  ( 85.00000000000123634, 17.00000000000000000, 5.000000000000004441 ) ) ;
#40773=CARTESIAN_POINT ( 'NONE',  ( -64.99999999999940314, 17.00000000000000000, -54.99999999999999289 ) ) ;
#40783=VECTOR ( 'NONE', #40432, 1000.000000000000000 ) ;
#40786=ORIENTED_EDGE ( 'NONE', *, *, #2118, .T. ) ;
#40796=ORIENTED_EDGE ( 'NONE', *, *, #37565, .T. ) ;
#40800=VECTOR ( 'NONE', #10124, 1000.000000000000000 ) ;
#40802=ORIENTED_EDGE ( 'NONE', *, *, #31550, .F. ) ;
#40819=ORIENTED_EDGE ( 'NONE', *, *, #43264, .T. ) ;
#40829=LINE ( 'NONE', #2094, #49553 ) ;
#40832=ORIENTED_EDGE ( 'NONE', *, *, #22858, .T. ) ;
#40833=DIRECTION ( 'NONE',  ( 0.000000000000000000, 0.000000000000000000, -1.000000000000000000 ) ) ;
#40844=DIRECTION ( 'NONE',  ( 1.000000000000000000, 0.000000000000000000, -0.000000000000000000 ) ) ;
#40847=ORIENTED_EDGE ( 'NONE', *, *, #21954, .F. ) ;
#40858=ORIENTED_EDGE ( 'NONE', *, *, #1983, .F. ) ;
#40867=CARTESIAN_POINT ( 'NONE',  ( 85.00000000000184741, 16.00000000000000000, 65.00000000000000000 ) ) ;
#40870=DIRECTION ( 'NONE',  ( 0.000000000000000000, 0.000000000000000000, -1.000000000000000000 ) ) ;
#40872=EDGE_CURVE ( 'NONE', #37483, #40254, #11767, .T. ) ;
#40875=EDGE_CURVE ( 'NONE', #19127, #31678, #35651, .T. ) ;
#40877=ORIENTED_EDGE ( 'NONE', *, *, #17496, .F. ) ;
#40891=VECTOR ( 'NONE', #24639, 1000.000000000000000 ) ;
#40898=DIRECTION ( 'NONE',  ( -0.000000000000000000, -0.000000000000000000, -1.000000000000000000 ) ) ;
#40903=ORIENTED_EDGE ( 'NONE', *, *, #46223, .F. ) ;
#40909=ORIENTED_EDGE ( 'NONE', *, *, #3194, .F. ) ;
#40917=PLANE ( 'NONE',  #24323 ) ;
#40919=EDGE_LOOP ( 'NONE', ( #25830, #47040, #34584, #28044 ) ) ;
#40926=CARTESIAN_POINT ( 'NONE',  ( -19.99999999999940670, 17.00000000000000000, -54.99999999999999289 ) ) ;
#40929=VECTOR ( 'NONE', #19360, 1000.000000000000000 ) ;
#40932=VERTEX_POINT ( 'NONE', #47881 ) ;
#40938=CARTESIAN_POINT ( 'NONE',  ( 80.00000000000061107, 17.00000000000000000, -30.00000000000000000 ) ) ;
#40959=VECTOR ( 'NONE', #38514, 1000.000000000000000 ) ;
#40961=PLANE ( 'NONE',  #14801 ) ;
#40968=EDGE_LOOP ( 'NONE', ( #15834, #19157, #21094, #23041 ) ) ;
#40970=AXIS2_PLACEMENT_3D ( 'NONE', #45160, #10048, #33658 ) ;
#40971=CARTESIAN_POINT ( 'NONE',  ( 164.9999999999999716, 16.00000000000000000, -90.00000000000000000 ) ) ;
#40974=VECTOR ( 'NONE', #13374, 1000.000000000000000 ) ;
#40981=ORIENTED_EDGE ( 'NONE', *, *, #28450, .T. ) ;
#40988=LINE ( 'NONE', #37163, #28803 ) ;
#40990=LINE ( 'NONE', #16894, #18550 ) ;
#41001=VECTOR ( 'NONE', #2043, 1000.000000000000000 ) ;
#41006=DIRECTION ( 'NONE',  ( 1.000000000000000000, 0.000000000000000000, 0.000000000000000000 ) ) ;
#41010=DIRECTION ( 'NONE',  ( 0.000000000000000000, 0.000000000000000000, 1.000000000000000000 ) ) ;
#41012=EDGE_LOOP ( 'NONE', ( #30549, #33398, #22337, #46724 ) ) ;
#41013=FACE_OUTER_BOUND ( 'NONE', #7360, .T. ) ;
#41019=DIRECTION ( 'NONE',  ( -1.000000000000000000, 0.000000000000000000, -0.000000000000000000 ) ) ;
#41020=ORIENTED_EDGE ( 'NONE', *, *, #23279, .F. ) ;
#41024=DIRECTION ( 'NONE',  ( -0.000000000000000000, -1.000000000000000000, -0.000000000000000000 ) ) ;
#41035=ORIENTED_EDGE ( 'NONE', *, *, #23647, .F. ) ;
#41048=LINE ( 'NONE', #5888, #20657 ) ;
#41060=CARTESIAN_POINT ( 'NONE',  ( 80.00000000000217426, 17.00000000000000000, 115.0000000000000142 ) ) ;
#41061=ORIENTED_EDGE ( 'NONE', *, *, #27587, .T. ) ;
#41079=( NAMED_UNIT ( * ) SI_UNIT ( $, .STERADIAN. ) SOLID_ANGLE_UNIT ( ) );
#41086=LINE ( 'NONE', #21577, #5395 ) ;
#41095=VERTEX_POINT ( 'NONE', #21473 ) ;
#41101=ADVANCED_FACE ( 'NONE', ( #2484 ), #10686, .F. ) ;
#41102=DIRECTION ( 'NONE',  ( 0.000000000000000000, 0.000000000000000000, -1.000000000000000000 ) ) ;
#41110=CARTESIAN_POINT ( 'NONE',  ( -64.99999999999815259, 17.00000000000000000, 90.00000000000000000 ) ) ;
#41116=LINE ( 'NONE', #32939, #2315 ) ;
#41119=PLANE ( 'NONE',  #15109 ) ;
#41123=DIRECTION ( 'NONE',  ( -0.000000000000000000, -1.000000000000000000, -0.000000000000000000 ) ) ;
#41135=DIRECTION ( 'NONE',  ( -0.000000000000000000, -0.000000000000000000, -1.000000000000000000 ) ) ;
#41137=CARTESIAN_POINT ( 'NONE',  ( -164.9999999999981526, 17.00000000000000000, 65.00000000000000000 ) ) ;
#41142=LINE ( 'NONE', #9843, #31234 ) ;
#41147=LINE ( 'NONE', #49803, #5303 ) ;
#41148=CARTESIAN_POINT ( 'NONE',  ( -114.9999999999987779, 17.00000000000000000, 5.000000000000004441 ) ) ;
#41158=LINE ( 'NONE', #18304, #50477 ) ;
#41170=CARTESIAN_POINT ( 'NONE',  ( -165.0000000000000284, 16.00000000000000000, 5.000000000000004441 ) ) ;
#41177=FACE_BOUND ( 'NONE', #48684, .T. ) ;
#41184=LINE ( 'NONE', #13981, #41880 ) ;
#41187=ADVANCED_FACE ( 'NONE', ( #19402 ), #3478, .F. ) ;
#41194=VECTOR ( 'NONE', #37981, 1000.000000000000000 ) ;
#41197=EDGE_LOOP ( 'NONE', ( #10531, #8351, #9706, #2114 ) ) ;
#41199=VECTOR ( 'NONE', #35102, 1000.000000000000000 ) ;
#41206=ORIENTED_EDGE ( 'NONE', *, *, #9251, .T. ) ;
#41214=ORIENTED_EDGE ( 'NONE', *, *, #27469, .T. ) ;
#41217=PLANE ( 'NONE',  #5046 ) ;
#41220=VERTEX_POINT ( 'NONE', #47065 ) ;
#41231=VECTOR ( 'NONE', #48348, 1000.000000000000000 ) ;
#41239=LINE ( 'NONE', #41499, #34525 ) ;
#41244=VERTEX_POINT ( 'NONE', #4265 ) ;
#41248=EDGE_LOOP ( 'NONE', ( #38386, #49240, #44101, #27989 ) ) ;
#41249=DIRECTION ( 'NONE',  ( -1.000000000000000000, -0.000000000000000000, -0.000000000000000000 ) ) ;
#41250=VECTOR ( 'NONE', #46491, 1000.000000000000000 ) ;
#41252=EDGE_LOOP ( 'NONE', ( #47161, #21095, #17602, #6255 ) ) ;
#41254=CARTESIAN_POINT ( 'NONE',  ( -64.99999999999815259, 17.00000000000000000, 65.00000000000000000 ) ) ;
#41256=ADVANCED_FACE ( 'NONE', ( #17066 ), #4760, .F. ) ;
#41266=EDGE_LOOP ( 'NONE', ( #8302, #40609, #31717, #47754 ) ) ;
#41268=LINE ( 'NONE', #12820, #15898 ) ;
#41276=CARTESIAN_POINT ( 'NONE',  ( -64.99999999999971578, 17.00000000000000000, -60.00000000000000000 ) ) ;
#41285=LINE ( 'NONE', #18685, #18827 ) ;
#41287=DIRECTION ( 'NONE',  ( -0.000000000000000000, -1.000000000000000000, -0.000000000000000000 ) ) ;
#41297=DIRECTION ( 'NONE',  ( 1.000000000000000000, 0.000000000000000000, -0.000000000000000000 ) ) ;
#41303=DIRECTION ( 'NONE',  ( 0.000000000000000000, -1.000000000000000000, 0.000000000000000000 ) ) ;
#41304=EDGE_LOOP ( 'NONE', ( #43617, #4725, #27444, #15271 ) ) ;
#41318=CARTESIAN_POINT ( 'NONE',  ( -70.00000000000002842, 17.00000000000000000, -114.9999999999999858 ) ) ;
#41323=ORIENTED_EDGE ( 'NONE', *, *, #38374, .T. ) ;
#41324=LINE ( 'NONE', #6174, #8190 ) ;
#41326=LINE ( 'NONE', #11033, #32806 ) ;
#41327=CARTESIAN_POINT ( 'NONE',  ( -64.99999999999909051, 16.00000000000000000, -24.99999999999999289 ) ) ;
#41334=AXIS2_PLACEMENT_3D ( 'NONE', #25284, #32502, #25538 ) ;
#41342=ORIENTED_EDGE ( 'NONE', *, *, #43707, .F. ) ;
#41347=CARTESIAN_POINT ( 'NONE',  ( -19.99999999999846523, 17.00000000000000000, 35.00000000000000000 ) ) ;
#41352=CARTESIAN_POINT ( 'NONE',  ( -19.99999999999815969, 17.00000000000000000, 65.00000000000000000 ) ) ;
#41361=CARTESIAN_POINT ( 'NONE',  ( 130.0000000000008811, 17.00000000000000000, -24.99999999999999289 ) ) ;
#41363=PLANE ( 'NONE',  #40666 ) ;
#41367=ORIENTED_EDGE ( 'NONE', *, *, #24874, .T. ) ;
#41374=CARTESIAN_POINT ( 'NONE',  ( -114.9999999999978542, 17.00000000000000000, 95.00000000000000000 ) ) ;
#41388=DIRECTION ( 'NONE',  ( -0.000000000000000000, -0.000000000000000000, -1.000000000000000000 ) ) ;
#41394=ORIENTED_EDGE ( 'NONE', *, *, #35375, .F. ) ;
#41397=DIRECTION ( 'NONE',  ( 0.000000000000000000, 0.000000000000000000, 1.000000000000000000 ) ) ;
#41403=VECTOR ( 'NONE', #47033, 1000.000000000000000 ) ;
#41410=DIRECTION ( 'NONE',  ( 1.000000000000000000, 0.000000000000000000, 0.000000000000000000 ) ) ;
#41411=VERTEX_POINT ( 'NONE', #2181 ) ;
#41412=VECTOR ( 'NONE', #21110, 1000.000000000000000 ) ;
#41414=CARTESIAN_POINT ( 'NONE',  ( -164.9999999999997442, 17.00000000000000000, -84.99999999999998579 ) ) ;
#41417=VERTEX_POINT ( 'NONE', #45496 ) ;
#41422=CARTESIAN_POINT ( 'NONE',  ( 135.0000000000019043, 16.00000000000000000, 65.00000000000000000 ) ) ;
#41424=LINE ( 'NONE', #45738, #19033 ) ;
#41435=CARTESIAN_POINT ( 'NONE',  ( -164.9999999999990905, 17.00000000000000000, -24.99999999999999289 ) ) ;
#41437=DIRECTION ( 'NONE',  ( 0.000000000000000000, -1.000000000000000000, 0.000000000000000000 ) ) ;
#41450=AXIS2_PLACEMENT_3D ( 'NONE', #29482, #29994, #10991 ) ;
#41452=VECTOR ( 'NONE', #27739, 1000.000000000000000 ) ;
#41455=PLANE ( 'NONE',  #33223 ) ;
#41457=ORIENTED_EDGE ( 'NONE', *, *, #3926, .T. ) ;
#41467=ORIENTED_EDGE ( 'NONE', *, *, #7095, .F. ) ;
#41479=EDGE_LOOP ( 'NONE', ( #3348, #22904, #393, #5794 ) ) ;
#41495=CARTESIAN_POINT ( 'NONE',  ( 164.9999999999999716, 17.00000000000000000, -1.387778780781445676E-14 ) ) ;
#41496=ADVANCED_FACE ( 'NONE', ( #45240 ), #2425, .F. ) ;
#41499=CARTESIAN_POINT ( 'NONE',  ( -69.99999999999847944, 16.00000000000000000, 35.00000000000000000 ) ) ;
#41509=LINE ( 'NONE', #30465, #10909 ) ;
#41514=CARTESIAN_POINT ( 'NONE',  ( 135.0000000000000000, 17.00000000000000000, -90.00000000000000000 ) ) ;
#41515=LINE ( 'NONE', #2753, #47547 ) ;
#41520=DIRECTION ( 'NONE',  ( -0.000000000000000000, -1.000000000000000000, -0.000000000000000000 ) ) ;
#41524=DIRECTION ( 'NONE',  ( -1.000000000000000000, 0.000000000000000000, -0.000000000000000000 ) ) ;
#41527=CARTESIAN_POINT ( 'NONE',  ( 80.00000000000028422, 16.00000000000000000, -84.99999999999998579 ) ) ;
#41529=ADVANCED_FACE ( 'NONE', ( #34499 ), #7550, .F. ) ;
#41537=ADVANCED_FACE ( 'NONE', ( #19341 ), #8065, .F. ) ;
#41538=CARTESIAN_POINT ( 'NONE',  ( 80.00000000000092371, 17.00000000000000000, -24.99999999999999289 ) ) ;
#41542=CARTESIAN_POINT ( 'NONE',  ( 135.0000000000006253, 17.00000000000000000, -54.99999999999999289 ) ) ;
#41548=DIRECTION ( 'NONE',  ( -0.000000000000000000, -1.000000000000000000, -0.000000000000000000 ) ) ;
#41553=CARTESIAN_POINT ( 'NONE',  ( -114.9999999999997158, 16.00000000000000000, -84.99999999999998579 ) ) ;
#41555=CARTESIAN_POINT ( 'NONE',  ( -64.99999999999909051, 16.00000000000000000, -24.99999999999999289 ) ) ;
#41569=EDGE_CURVE ( 'NONE', #325, #26536, #31413, .T. ) ;
#41577=CARTESIAN_POINT ( 'NONE',  ( -119.9999999999984652, 17.00000000000000000, 35.00000000000000000 ) ) ;
#41584=VECTOR ( 'NONE', #6018, 1000.000000000000000 ) ;
#41585=VERTEX_POINT ( 'NONE', #4207 ) ;
#41589=CARTESIAN_POINT ( 'NONE',  ( -69.99999999999940314, 17.00000000000000000, -54.99999999999999289 ) ) ;
#41596=EDGE_CURVE ( 'NONE', #25400, #13070, #13155, .T. ) ;
#41597=FACE_OUTER_BOUND ( 'NONE', #37184, .T. ) ;
#41604=EDGE_LOOP ( 'NONE', ( #9764, #48430, #26220, #6564 ) ) ;
#41611=LINE ( 'NONE', #41361, #27753 ) ;
#41619=ORIENTED_EDGE ( 'NONE', *, *, #4340, .F. ) ;
#41638=CARTESIAN_POINT ( 'NONE',  ( 130.0000000000015064, 16.00000000000000000, 35.00000000000000000 ) ) ;
#41643=EDGE_CURVE ( 'NONE', #15451, #17054, #4710, .T. ) ;
#41646=ORIENTED_EDGE ( 'NONE', *, *, #43112, .T. ) ;
#41653=CARTESIAN_POINT ( 'NONE',  ( 80.00000000000122213, 16.00000000000000000, 5.000000000000004441 ) ) ;
#41659=DIRECTION ( 'NONE',  ( 1.000000000000000000, 0.000000000000000000, -0.000000000000000000 ) ) ;
#41684=FACE_OUTER_BOUND ( 'NONE', #10783, .T. ) ;
#41687=LINE ( 'NONE', #3176, #27426 ) ;
#41694=CARTESIAN_POINT ( 'NONE',  ( -64.99999999999846523, 17.00000000000000000, 60.00000000000000000 ) ) ;
#41712=ORIENTED_EDGE ( 'NONE', *, *, #766, .F. ) ;
#41715=ORIENTED_EDGE ( 'NONE', *, *, #3888, .F. ) ;
#41720=ORIENTED_EDGE ( 'NONE', *, *, #21834, .T. ) ;
#41727=FACE_OUTER_BOUND ( 'NONE', #22679, .T. ) ;
#41729=ORIENTED_EDGE ( 'NONE', *, *, #5130, .T. ) ;
#41745=DIRECTION ( 'NONE',  ( 0.000000000000000000, 0.000000000000000000, 1.000000000000000000 ) ) ;
#41758=CARTESIAN_POINT ( 'NONE',  ( 129.9999999999999432, 17.00000000000000000, -90.00000000000000000 ) ) ;
#41765=ORIENTED_EDGE ( 'NONE', *, *, #48093, .T. ) ;
#41776=LINE ( 'NONE', #26641, #28908 ) ;
#41779=ORIENTED_EDGE ( 'NONE', *, *, #26240, .T. ) ;
#41784=ORIENTED_EDGE ( 'NONE', *, *, #36641, .T. ) ;
#41787=ADVANCED_FACE ( 'NONE', ( #9565 ), #22118, .F. ) ;
#41790=VECTOR ( 'NONE', #3389, 1000.000000000000000 ) ;
#41800=LINE ( 'NONE', #3550, #530 ) ;
#41801=VECTOR ( 'NONE', #3807, 1000.000000000000000 ) ;
#41804=VERTEX_POINT ( 'NONE', #21610 ) ;
#41807=CARTESIAN_POINT ( 'NONE',  ( -164.9999999999978400, 17.00000000000000000, 95.00000000000000000 ) ) ;
#41814=LINE ( 'NONE', #26679, #13834 ) ;
#41816=EDGE_CURVE ( 'NONE', #25407, #24059, #2123, .T. ) ;
#41822=EDGE_CURVE ( 'NONE', #39034, #13738, #2603, .T. ) ;
#41830=ORIENTED_EDGE ( 'NONE', *, *, #4593, .F. ) ;
#41831=EDGE_CURVE ( 'NONE', #6173, #1878, #27680, .T. ) ;
#41840=CARTESIAN_POINT ( 'NONE',  ( 130.0000000000005684, 17.00000000000000000, -30.00000000000000000 ) ) ;
#41844=AXIS2_PLACEMENT_3D ( 'NONE', #31561, #46641, #43585 ) ;
#41858=CARTESIAN_POINT ( 'NONE',  ( 30.00000000000029132, 17.00000000000000000, -84.99999999999998579 ) ) ;
#41859=LINE ( 'NONE', #7222, #17361 ) ;
#41862=VERTEX_POINT ( 'NONE', #23835 ) ;
#41868=VERTEX_POINT ( 'NONE', #11777 ) ;
#41869=EDGE_LOOP ( 'NONE', ( #32820, #33837, #25413, #4187 ) ) ;
#41871=LINE ( 'NONE', #2852, #49041 ) ;
#41879=LINE ( 'NONE', #22884, #26114 ) ;
#41880=VECTOR ( 'NONE', #17591, 1000.000000000000000 ) ;
#41884=CARTESIAN_POINT ( 'NONE',  ( -69.99999999999847944, 17.00000000000000000, 35.00000000000000000 ) ) ;
#41885=VERTEX_POINT ( 'NONE', #19971 ) ;
#41895=VERTEX_POINT ( 'NONE', #50469 ) ;
#41899=ADVANCED_FACE ( 'NONE', ( #4077 ), #38730, .F. ) ;
#41904=DIRECTION ( 'NONE',  ( -1.000000000000000000, -0.000000000000000000, -0.000000000000000000 ) ) ;
#41909=LINE ( 'NONE', #6756, #15939 ) ;
#41913=VERTEX_POINT ( 'NONE', #27177 ) ;
#41914=DIRECTION ( 'NONE',  ( 1.000000000000000000, 0.000000000000000000, -0.000000000000000000 ) ) ;
#41919=ADVANCED_FACE ( 'NONE', ( #46880 ), #32553, .F. ) ;
#41923=ORIENTED_EDGE ( 'NONE', *, *, #16757, .F. ) ;
#41934=EDGE_CURVE ( 'NONE', #26648, #7228, #40747, .T. ) ;
#41938=FACE_OUTER_BOUND ( 'NONE', #33530, .T. ) ;
#41943=CARTESIAN_POINT ( 'NONE',  ( -69.99999999999909051, 16.00000000000000000, 0.000000000000000000 ) ) ;
#41952=VERTEX_POINT ( 'NONE', #24843 ) ;
#41960=ORIENTED_EDGE ( 'NONE', *, *, #44584, .T. ) ;
#41969=ORIENTED_EDGE ( 'NONE', *, *, #41831, .T. ) ;
#41971=ORIENTED_EDGE ( 'NONE', *, *, #49451, .T. ) ;
#41973=LINE ( 'NONE', #3988, #23435 ) ;
#41976=ADVANCED_FACE ( 'NONE', ( #20731 ), #36150, .F. ) ;
#41978=ADVANCED_FACE ( 'NONE', ( #44067 ), #32299, .F. ) ;
#41983=ORIENTED_EDGE ( 'NONE', *, *, #47852, .T. ) ;
#41984=CARTESIAN_POINT ( 'NONE',  ( 0.000000000000000000, 17.00000000000000000, 0.000000000000000000 ) ) ;
#41999=ADVANCED_FACE ( 'NONE', ( #21480 ), #17138, .F. ) ;
#42000=FACE_OUTER_BOUND ( 'NONE', #15589, .T. ) ;
#42002=DIRECTION ( 'NONE',  ( -1.000000000000000000, -0.000000000000000000, -0.000000000000000000 ) ) ;
#42008=LINE ( 'NONE', #9949, #36528 ) ;
#42017=EDGE_CURVE ( 'NONE', #24878, #32976, #44816, .T. ) ;
#42026=CARTESIAN_POINT ( 'NONE',  ( -14.99999999999970868, 17.00000000000000000, -84.99999999999998579 ) ) ;
#42030=CARTESIAN_POINT ( 'NONE',  ( 135.0000000000021600, 17.00000000000000000, 95.00000000000000000 ) ) ;
#42031=ORIENTED_EDGE ( 'NONE', *, *, #11182, .T. ) ;
#42034=CARTESIAN_POINT ( 'NONE',  ( 29.99999999999998579, 16.00000000000000000, -90.00000000000000000 ) ) ;
#42041=ORIENTED_EDGE ( 'NONE', *, *, #27062, .T. ) ;
#42047=FACE_BOUND ( 'NONE', #45492, .T. ) ;
#42048=PLANE ( 'NONE',  #37475 ) ;
#42052=DIRECTION ( 'NONE',  ( -1.000000000000000000, -0.000000000000000000, -0.000000000000000000 ) ) ;
#42055=CARTESIAN_POINT ( 'NONE',  ( -164.9999999999984936, 17.00000000000000000, 60.00000000000000000 ) ) ;
#42059=CARTESIAN_POINT ( 'NONE',  ( 85.00000000000184741, 17.00000000000000000, 65.00000000000000000 ) ) ;
#42065=PLANE ( 'NONE',  #17596 ) ;
#42069=ORIENTED_EDGE ( 'NONE', *, *, #12300, .T. ) ;
#42083=DIRECTION ( 'NONE',  ( -1.000000000000000000, -0.000000000000000000, -0.000000000000000000 ) ) ;
#42092=VERTEX_POINT ( 'NONE', #41495 ) ;
#42100=ORIENTED_EDGE ( 'NONE', *, *, #10879, .F. ) ;
#42106=ORIENTED_EDGE ( 'NONE', *, *, #47342, .F. ) ;
#42109=ORIENTED_EDGE ( 'NONE', *, *, #35720, .F. ) ;
#42113=LINE ( 'NONE', #26474, #11935 ) ;
#42128=DIRECTION ( 'NONE',  ( 1.000000000000000000, 0.000000000000000000, 0.000000000000000000 ) ) ;
#42129=EDGE_CURVE ( 'NONE', #24997, #42678, #29689, .T. ) ;
#42130=LINE ( 'NONE', #22641, #6673 ) ;
#42133=EDGE_CURVE ( 'NONE', #19097, #26042, #14285, .T. ) ;
#42140=ADVANCED_FACE ( 'NONE', ( #42000 ), #10443, .F. ) ;
#42142=VECTOR ( 'NONE', #22640, 1000.000000000000000 ) ;
#42145=ORIENTED_EDGE ( 'NONE', *, *, #5791, .F. ) ;
#42146=FACE_OUTER_BOUND ( 'NONE', #39486, .T. ) ;
#42151=DIRECTION ( 'NONE',  ( -0.000000000000000000, -0.000000000000000000, 1.000000000000000000 ) ) ;
#42152=DIRECTION ( 'NONE',  ( 0.000000000000000000, 0.000000000000000000, 1.000000000000000000 ) ) ;
#42153=LINE ( 'NONE', #11631, #1828 ) ;
#42156=EDGE_LOOP ( 'NONE', ( #49600, #15230, #23211, #35574 ) ) ;
#42157=LINE ( 'NONE', #42407, #4199 ) ;
#42166=VERTEX_POINT ( 'NONE', #47329 ) ;
#42173=EDGE_CURVE ( 'NONE', #39178, #9900, #34563, .T. ) ;
#42175=VERTEX_POINT ( 'NONE', #50664 ) ;
#42177=DIRECTION ( 'NONE',  ( 0.000000000000000000, 0.000000000000000000, 1.000000000000000000 ) ) ;
#42180=VECTOR ( 'NONE', #29925, 1000.000000000000000 ) ;
#42183=DIRECTION ( 'NONE',  ( -0.000000000000000000, -1.000000000000000000, -0.000000000000000000 ) ) ;
#42185=CARTESIAN_POINT ( 'NONE',  ( 85.00000000000184741, 17.00000000000000000, 65.00000000000000000 ) ) ;
#42191=DIRECTION ( 'NONE',  ( 1.000000000000000000, 0.000000000000000000, 0.000000000000000000 ) ) ;
#42193=CARTESIAN_POINT ( 'NONE',  ( 129.9999999999999432, 17.00000000000000000, -114.9999999999999858 ) ) ;
#42194=CARTESIAN_POINT ( 'NONE',  ( 130.0000000000002842, 16.00000000000000000, -84.99999999999998579 ) ) ;
#42198=EDGE_CURVE ( 'NONE', #33858, #7870, #23775, .T. ) ;
#42221=VECTOR ( 'NONE', #17690, 1000.000000000000000 ) ;
#42230=ORIENTED_EDGE ( 'NONE', *, *, #10486, .F. ) ;
#42245=DIRECTION ( 'NONE',  ( 1.000000000000000000, 0.000000000000000000, 0.000000000000000000 ) ) ;
#42250=FACE_OUTER_BOUND ( 'NONE', #48858, .T. ) ;
#42273=ORIENTED_EDGE ( 'NONE', *, *, #12631, .F. ) ;
#42281=CARTESIAN_POINT ( 'NONE',  ( -165.0000000000000284, 17.00000000000000000, -114.9999999999999858 ) ) ;
#42292=ORIENTED_EDGE ( 'NONE', *, *, #46571, .F. ) ;
#42296=AXIS2_PLACEMENT_3D ( 'NONE', #24351, #4585, #27176 ) ;
#42297=ORIENTED_EDGE ( 'NONE', *, *, #29353, .F. ) ;
#42302=VECTOR ( 'NONE', #34671, 1000.000000000000000 ) ;
#42303=DIRECTION ( 'NONE',  ( 1.000000000000000000, 0.000000000000000000, 0.000000000000000000 ) ) ;
#42308=PLANE ( 'NONE',  #13417 ) ;
#42311=ADVANCED_FACE ( 'NONE', ( #48332 ), #43764, .F. ) ;
#42320=CARTESIAN_POINT ( 'NONE',  ( 135.0000000000015632, 17.00000000000000000, 35.00000000000000000 ) ) ;
#42324=ORIENTED_EDGE ( 'NONE', *, *, #40442, .F. ) ;
#42330=DIRECTION ( 'NONE',  ( 1.000000000000000000, 0.000000000000000000, 0.000000000000000000 ) ) ;
#42337=DIRECTION ( 'NONE',  ( -0.000000000000000000, -1.000000000000000000, -0.000000000000000000 ) ) ;
#42338=VERTEX_POINT ( 'NONE', #20166 ) ;
#42343=ORIENTED_EDGE ( 'NONE', *, *, #48382, .F. ) ;
#42345=CARTESIAN_POINT ( 'NONE',  ( 164.9999999999999716, 16.00000000000000000, 115.0000000000000142 ) ) ;
#42354=CARTESIAN_POINT ( 'NONE',  ( 135.0000000000009663, 16.00000000000000000, -24.99999999999999289 ) ) ;
#42362=CARTESIAN_POINT ( 'NONE',  ( -19.99999999999878142, 17.00000000000000000, 30.00000000000000000 ) ) ;
#42371=CARTESIAN_POINT ( 'NONE',  ( 30.00000000000153833, 17.00000000000000000, 60.00000000000000000 ) ) ;
#42373=DIRECTION ( 'NONE',  ( -0.000000000000000000, -1.000000000000000000, -0.000000000000000000 ) ) ;
#42375=CARTESIAN_POINT ( 'NONE',  ( -14.99999999999937472, 16.00000000000000000, -54.99999999999999289 ) ) ;
#42384=LINE ( 'NONE', #46457, #33957 ) ;
#42385=CARTESIAN_POINT ( 'NONE',  ( -14.99999999999812594, 16.00000000000000000, 90.00000000000000000 ) ) ;
#42390=DIRECTION ( 'NONE',  ( 1.000000000000000000, 0.000000000000000000, 0.000000000000000000 ) ) ;
#42392=ADVANCED_FACE ( 'NONE', ( #9379 ), #32498, .F. ) ;
#42397=ORIENTED_EDGE ( 'NONE', *, *, #6251, .F. ) ;
#42400=CARTESIAN_POINT ( 'NONE',  ( -64.99999999999783995, 17.00000000000000000, 95.00000000000000000 ) ) ;
#42403=DIRECTION ( 'NONE',  ( 0.000000000000000000, 0.000000000000000000, -1.000000000000000000 ) ) ;
#42407=CARTESIAN_POINT ( 'NONE',  ( -64.99999999999877787, 17.00000000000000000, 30.00000000000000000 ) ) ;
#42413=VERTEX_POINT ( 'NONE', #35850 ) ;
#42416=CARTESIAN_POINT ( 'NONE',  ( -64.99999999999783995, 16.00000000000000000, 95.00000000000000000 ) ) ;
#42419=ADVANCED_FACE ( 'NONE', ( #28127 ), #24290, .F. ) ;
#42420=ADVANCED_FACE ( 'NONE', ( #8633 ), #12719, .T. ) ;
#42428=DIRECTION ( 'NONE',  ( 1.000000000000000000, 0.000000000000000000, -0.000000000000000000 ) ) ;
#42432=VERTEX_POINT ( 'NONE', #6534 ) ;
#42440=CARTESIAN_POINT ( 'NONE',  ( -114.9999999999981526, 16.00000000000000000, 65.00000000000000000 ) ) ;
#42457=DIRECTION ( 'NONE',  ( -0.000000000000000000, -0.000000000000000000, -1.000000000000000000 ) ) ;
#42463=EDGE_LOOP ( 'NONE', ( #45698, #17920, #19497, #46452 ) ) ;
#42467=DIRECTION ( 'NONE',  ( 0.000000000000000000, -0.000000000000000000, -1.000000000000000000 ) ) ;
#42468=ORIENTED_EDGE ( 'NONE', *, *, #7538, .F. ) ;
#42470=LINE ( 'NONE', #7091, #20038 ) ;
#42474=VERTEX_POINT ( 'NONE', #30142 ) ;
#42476=CARTESIAN_POINT ( 'NONE',  ( 175.0000000000000000, 15.00000000000000000, -122.5000000000000000 ) ) ;
#42479=ADVANCED_FACE ( 'NONE', ( #33255 ), #30398, .F. ) ;
#42486=CARTESIAN_POINT ( 'NONE',  ( -69.99999999999972999, 16.00000000000000000, -60.00000000000000000 ) ) ;
#42488=AXIS2_PLACEMENT_3D ( 'NONE', #22943, #14744, #4218 ) ;
#42495=ADVANCED_FACE ( 'NONE', ( #41684 ), #46504, .F. ) ;
#42522=DIRECTION ( 'NONE',  ( -0.000000000000000000, -0.000000000000000000, -1.000000000000000000 ) ) ;
#42527=CARTESIAN_POINT ( 'NONE',  ( 30.00000000000187228, 17.00000000000000000, 65.00000000000000000 ) ) ;
#42530=LINE ( 'NONE', #23034, #5370 ) ;
#42542=PLANE ( 'NONE',  #45868 ) ;
#42550=EDGE_CURVE ( 'NONE', #30097, #27796, #34774, .T. ) ;
#42551=DIRECTION ( 'NONE',  ( 1.000000000000000000, 0.000000000000000000, 0.000000000000000000 ) ) ;
#42552=AXIS2_PLACEMENT_3D ( 'NONE', #12921, #1400, #9091 ) ;
#42567=DIRECTION ( 'NONE',  ( -0.000000000000000000, -1.000000000000000000, -0.000000000000000000 ) ) ;
#42569=ORIENTED_EDGE ( 'NONE', *, *, #12383, .T. ) ;
#42583=CARTESIAN_POINT ( 'NONE',  ( 164.9999999999999716, 16.00000000000000000, 35.00000000000000000 ) ) ;
#42590=CARTESIAN_POINT ( 'NONE',  ( -114.9999999999987779, 17.00000000000000000, 5.000000000000004441 ) ) ;
#42594=DIRECTION ( 'NONE',  ( -0.000000000000000000, -1.000000000000000000, -0.000000000000000000 ) ) ;
#42595=CARTESIAN_POINT ( 'NONE',  ( -115.0000000000000284, 16.00000000000000000, -90.00000000000000000 ) ) ;
#42598=VECTOR ( 'NONE', #13259, 1000.000000000000000 ) ;
#42612=ORIENTED_EDGE ( 'NONE', *, *, #31926, .F. ) ;
#42613=ORIENTED_EDGE ( 'NONE', *, *, #44807, .F. ) ;
#42614=ADVANCED_FACE ( 'NONE', ( #27048 ), #42686, .F. ) ;
#42619=CARTESIAN_POINT ( 'NONE',  ( -19.99999999999846523, 17.00000000000000000, 60.00000000000000000 ) ) ;
#42621=DIRECTION ( 'NONE',  ( -1.000000000000000000, -0.000000000000000000, -0.000000000000000000 ) ) ;
#42631=VERTEX_POINT ( 'NONE', #880 ) ;
#42635=VECTOR ( 'NONE', #30763, 1000.000000000000000 ) ;
#42636=CARTESIAN_POINT ( 'NONE',  ( -14.99999999999812594, 16.00000000000000000, 65.00000000000000000 ) ) ;
#42638=VECTOR ( 'NONE', #24510, 1000.000000000000000 ) ;
#42642=CARTESIAN_POINT ( 'NONE',  ( -14.99999999999876366, 16.00000000000000000, 30.00000000000000000 ) ) ;
#42643=DIRECTION ( 'NONE',  ( 0.000000000000000000, 0.000000000000000000, -1.000000000000000000 ) ) ;
#42661=VERTEX_POINT ( 'NONE', #47274 ) ;
#42668=EDGE_LOOP ( 'NONE', ( #19329, #42297, #42343, #37367 ) ) ;
#42669=VERTEX_POINT ( 'NONE', #20110 ) ;
#42674=VECTOR ( 'NONE', #3772, 1000.000000000000000 ) ;
#42678=VERTEX_POINT ( 'NONE', #24730 ) ;
#42686=PLANE ( 'NONE',  #32104 ) ;
#42688=FACE_OUTER_BOUND ( 'NONE', #43659, .T. ) ;
#42691=FACE_OUTER_BOUND ( 'NONE', #32463, .T. ) ;
#42695=AXIS2_PLACEMENT_3D ( 'NONE', #4197, #19833, #27030 ) ;
#42699=DIRECTION ( 'NONE',  ( -1.000000000000000000, -0.000000000000000000, -0.000000000000000000 ) ) ;
#42715=FACE_OUTER_BOUND ( 'NONE', #8373, .T. ) ;
#42717=CARTESIAN_POINT ( 'NONE',  ( -119.9999999999990905, 17.00000000000000000, 0.000000000000000000 ) ) ;
#42719=CARTESIAN_POINT ( 'NONE',  ( -164.9999999999981526, 17.00000000000000000, 65.00000000000000000 ) ) ;
#42722=ORIENTED_EDGE ( 'NONE', *, *, #30594, .F. ) ;
#42735=VECTOR ( 'NONE', #12106, 1000.000000000000000 ) ;
#42737=ORIENTED_EDGE ( 'NONE', *, *, #8791, .F. ) ;
#42745=EDGE_LOOP ( 'NONE', ( #21909, #17849, #29941, #5006 ) ) ;
#42753=DIRECTION ( 'NONE',  ( 0.000000000000000000, 0.000000000000000000, -1.000000000000000000 ) ) ;
#42778=CARTESIAN_POINT ( 'NONE',  ( 135.0000000000000000, 17.00000000000000000, -90.00000000000000000 ) ) ;
#42784=ORIENTED_EDGE ( 'NONE', *, *, #28015, .F. ) ;
#42786=DIRECTION ( 'NONE',  ( -4.625929269271542120E-16, 0.000000000000000000, -1.000000000000000000 ) ) ;
#42801=VECTOR ( 'NONE', #35584, 1000.000000000000000 ) ;
#42812=DIRECTION ( 'NONE',  ( -1.000000000000000000, -0.000000000000000000, -0.000000000000000000 ) ) ;
#42828=ORIENTED_EDGE ( 'NONE', *, *, #27735, .T. ) ;
#42829=VERTEX_POINT ( 'NONE', #32945 ) ;
#42833=CARTESIAN_POINT ( 'NONE',  ( 85.00000000000029843, 17.00000000000000000, -84.99999999999998579 ) ) ;
#42840=ORIENTED_EDGE ( 'NONE', *, *, #39405, .F. ) ;
#42846=ORIENTED_EDGE ( 'NONE', *, *, #46483, .F. ) ;
#42851=PLANE ( 'NONE',  #7350 ) ;
#42855=ORIENTED_EDGE ( 'NONE', *, *, #50050, .F. ) ;
#42886=CARTESIAN_POINT ( 'NONE',  ( 30.00000000000123279, 16.00000000000000000, 30.00000000000000000 ) ) ;
#42889=DIRECTION ( 'NONE',  ( -0.000000000000000000, -0.000000000000000000, -1.000000000000000000 ) ) ;
#42896=EDGE_LOOP ( 'NONE', ( #23815, #35886, #28580, #31524 ) ) ;
#42902=VERTEX_POINT ( 'NONE', #50025 ) ;
#42904=ORIENTED_EDGE ( 'NONE', *, *, #7899, .T. ) ;
#42907=EDGE_CURVE ( 'NONE', #15777, #23917, #38805, .T. ) ;
#42913=ORIENTED_EDGE ( 'NONE', *, *, #9010, .F. ) ;
#42918=LINE ( 'NONE', #23689, #23868 ) ;
#42932=EDGE_LOOP ( 'NONE', ( #31654, #17394, #38352, #33657 ) ) ;
#42939=EDGE_LOOP ( 'NONE', ( #40450, #27615, #28411, #49053 ) ) ;
#42940=ORIENTED_EDGE ( 'NONE', *, *, #12797, .T. ) ;
#42943=CARTESIAN_POINT ( 'NONE',  ( -14.99999999999876366, 16.00000000000000000, 30.00000000000000000 ) ) ;
#42951=DIRECTION ( 'NONE',  ( 0.000000000000000000, 0.000000000000000000, 1.000000000000000000 ) ) ;
#42959=ORIENTED_EDGE ( 'NONE', *, *, #46280, .F. ) ;
#42973=EDGE_LOOP ( 'NONE', ( #9168, #48731, #26481, #25712 ) ) ;
#42975=ORIENTED_EDGE ( 'NONE', *, *, #46513, .T. ) ;
#42978=CARTESIAN_POINT ( 'NONE',  ( 0.000000000000000000, 17.00000000000000000, 0.000000000000000000 ) ) ;
#42979=ORIENTED_EDGE ( 'NONE', *, *, #33053, .T. ) ;
#42981=DIRECTION ( 'NONE',  ( 1.000000000000000000, 0.000000000000000000, 0.000000000000000000 ) ) ;
#42991=VERTEX_POINT ( 'NONE', #23395 ) ;
#43000=ORIENTED_EDGE ( 'NONE', *, *, #11177, .F. ) ;
#43003=DIRECTION ( 'NONE',  ( -0.000000000000000000, -0.000000000000000000, -1.000000000000000000 ) ) ;
#43008=ORIENTED_EDGE ( 'NONE', *, *, #40185, .F. ) ;
#43014=AXIS2_PLACEMENT_3D ( 'NONE', #41374, #1626, #6468 ) ;
#43018=CARTESIAN_POINT ( 'NONE',  ( -114.9999999999991047, 17.00000000000000000, 0.000000000000000000 ) ) ;
#43039=DIRECTION ( 'NONE',  ( 1.000000000000000000, 0.000000000000000000, 0.000000000000000000 ) ) ;
#43045=LINE ( 'NONE', #11510, #6569 ) ;
#43050=ORIENTED_EDGE ( 'NONE', *, *, #13329, .F. ) ;
#43052=DIRECTION ( 'NONE',  ( 0.000000000000000000, 0.000000000000000000, 1.000000000000000000 ) ) ;
#43056=PLANE ( 'NONE',  #48893 ) ;
#43058=CARTESIAN_POINT ( 'NONE',  ( -64.99999999999846523, 16.00000000000000000, 35.00000000000000000 ) ) ;
#43060=VECTOR ( 'NONE', #11262, 1000.000000000000000 ) ;
#43063=DIRECTION ( 'NONE',  ( -1.000000000000000000, 0.000000000000000000, -0.000000000000000000 ) ) ;
#43065=EDGE_CURVE ( 'NONE', #20271, #11044, #44383, .T. ) ;
#43066=EDGE_CURVE ( 'NONE', #3216, #7644, #28261, .T. ) ;
#43074=FACE_OUTER_BOUND ( 'NONE', #2848, .T. ) ;
#43075=CARTESIAN_POINT ( 'NONE',  ( 80.00000000000216005, 17.00000000000000000, 95.00000000000000000 ) ) ;
#43076=VERTEX_POINT ( 'NONE', #9258 ) ;
#43078=EDGE_CURVE ( 'NONE', #22969, #27259, #44137, .T. ) ;
#43079=LINE ( 'NONE', #43324, #13003 ) ;
#43080=DIRECTION ( 'NONE',  ( -0.000000000000000000, -1.000000000000000000, -0.000000000000000000 ) ) ;
#43085=VERTEX_POINT ( 'NONE', #40313 ) ;
#43092=ORIENTED_EDGE ( 'NONE', *, *, #41569, .T. ) ;
#43094=EDGE_CURVE ( 'NONE', #24059, #14851, #16695, .T. ) ;
#43097=VECTOR ( 'NONE', #36130, 1000.000000000000000 ) ;
#43101=LINE ( 'NONE', #4107, #38523 ) ;
#43110=VERTEX_POINT ( 'NONE', #19790 ) ;
#43112=EDGE_CURVE ( 'NONE', #33150, #27796, #31620, .T. ) ;
#43115=VERTEX_POINT ( 'NONE', #27750 ) ;
#43122=DIRECTION ( 'NONE',  ( -0.000000000000000000, -1.000000000000000000, -0.000000000000000000 ) ) ;
#43140=ADVANCED_FACE ( 'NONE', ( #47458 ), #8770, .F. ) ;
#43161=DIRECTION ( 'NONE',  ( 0.000000000000000000, 0.000000000000000000, -1.000000000000000000 ) ) ;
#43162=CARTESIAN_POINT ( 'NONE',  ( -175.0000000000000000, 15.00000000000000000, -122.5000000000000000 ) ) ;
#43163=ORIENTED_EDGE ( 'NONE', *, *, #6538, .F. ) ;
#43168=ORIENTED_EDGE ( 'NONE', *, *, #10829, .T. ) ;
#43171=DIRECTION ( 'NONE',  ( 0.000000000000000000, 0.000000000000000000, -1.000000000000000000 ) ) ;
#43172=DIRECTION ( 'NONE',  ( 1.000000000000000000, 0.000000000000000000, -0.000000000000000000 ) ) ;
#43174=ORIENTED_EDGE ( 'NONE', *, *, #39187, .F. ) ;
#43179=CARTESIAN_POINT ( 'NONE',  ( 130.0000000000012221, 16.00000000000000000, 5.000000000000004441 ) ) ;
#43180=ORIENTED_EDGE ( 'NONE', *, *, #338, .T. ) ;
#43185=VECTOR ( 'NONE', #33725, 1000.000000000000000 ) ;
#43186=LINE ( 'NONE', #23691, #25114 ) ;
#43193=DIRECTION ( 'NONE',  ( 0.000000000000000000, 0.000000000000000000, 1.000000000000000000 ) ) ;
#43198=DIRECTION ( 'NONE',  ( -1.000000000000000000, 0.000000000000000000, -0.000000000000000000 ) ) ;
#43199=ORIENTED_EDGE ( 'NONE', *, *, #49422, .T. ) ;
#43217=LINE ( 'NONE', #892, #38527 ) ;
#43228=AXIS2_PLACEMENT_3D ( 'NONE', #23957, #16259, #48016 ) ;
#43229=ORIENTED_EDGE ( 'NONE', *, *, #24434, .T. ) ;
#43240=ORIENTED_EDGE ( 'NONE', *, *, #39361, .T. ) ;
#43257=ADVANCED_FACE ( 'NONE', ( #48709 ), #25165, .F. ) ;
#43264=EDGE_CURVE ( 'NONE', #37192, #31020, #48461, .T. ) ;
#43283=ORIENTED_EDGE ( 'NONE', *, *, #13028, .T. ) ;
#43289=LINE ( 'NONE', #15352, #4664 ) ;
#43303=CARTESIAN_POINT ( 'NONE',  ( 34.99999999999997868, 16.00000000000000000, -114.9999999999999858 ) ) ;
#43308=CARTESIAN_POINT ( 'NONE',  ( 30.00000000000092726, 16.00000000000000000, 0.000000000000000000 ) ) ;
#43319=CARTESIAN_POINT ( 'NONE',  ( -69.99999999999879208, 17.00000000000000000, 5.000000000000004441 ) ) ;
#43324=CARTESIAN_POINT ( 'NONE',  ( -164.9999999999990905, 17.00000000000000000, 0.000000000000000000 ) ) ;
#43340=ORIENTED_EDGE ( 'NONE', *, *, #4381, .T. ) ;
#43342=VERTEX_POINT ( 'NONE', #50480 ) ;
#43343=CARTESIAN_POINT ( 'NONE',  ( -165.0000000000000284, 16.00000000000000000, 115.0000000000000142 ) ) ;
#43358=PLANE ( 'NONE',  #8700 ) ;
#43363=LINE ( 'NONE', #4383, #12630 ) ;
#43364=CARTESIAN_POINT ( 'NONE',  ( -114.9999999999981526, 17.00000000000000000, 90.00000000000000000 ) ) ;
#43373=ORIENTED_EDGE ( 'NONE', *, *, #35781, .F. ) ;
#43380=VERTEX_POINT ( 'NONE', #46635 ) ;
#43390=ORIENTED_EDGE ( 'NONE', *, *, #49692, .F. ) ;
#43396=PLANE ( 'NONE',  #10183 ) ;
#43399=LINE ( 'NONE', #28014, #12426 ) ;
#43416=VECTOR ( 'NONE', #42390, 1000.000000000000000 ) ;
#43418=ADVANCED_FACE ( 'NONE', ( #33535 ), #41217, .F. ) ;
#43427=ADVANCED_FACE ( 'NONE', ( #41727 ), #37905, .F. ) ;
#43451=EDGE_CURVE ( 'NONE', #950, #24182, #29422, .T. ) ;
#43459=FACE_OUTER_BOUND ( 'NONE', #6743, .T. ) ;
#43467=ORIENTED_EDGE ( 'NONE', *, *, #27154, .F. ) ;
#43488=ORIENTED_EDGE ( 'NONE', *, *, #40671, .T. ) ;
#43493=EDGE_CURVE ( 'NONE', #1405, #17026, #3154, .T. ) ;
#43496=VERTEX_POINT ( 'NONE', #19325 ) ;
#43501=VERTEX_POINT ( 'NONE', #3673 ) ;
#43505=ORIENTED_EDGE ( 'NONE', *, *, #25812, .F. ) ;
#43508=CARTESIAN_POINT ( 'NONE',  ( 30.00000000000219202, 16.00000000000000000, 115.0000000000000142 ) ) ;
#43534=LINE ( 'NONE', #22585, #9484 ) ;
#43537=EDGE_CURVE ( 'NONE', #24564, #3086, #11129, .T. ) ;
#43540=DIRECTION ( 'NONE',  ( -0.000000000000000000, -1.000000000000000000, -0.000000000000000000 ) ) ;
#43562=CARTESIAN_POINT ( 'NONE',  ( -65.00000000000002842, 17.00000000000000000, -114.9999999999999858 ) ) ;
#43563=VECTOR ( 'NONE', #15450, 1000.000000000000000 ) ;
#43582=VECTOR ( 'NONE', #1359, 1000.000000000000000 ) ;
#43585=DIRECTION ( 'NONE',  ( 0.000000000000000000, -0.000000000000000000, -1.000000000000000000 ) ) ;
#43586=EDGE_CURVE ( 'NONE', #33538, #23358, #23443, .T. ) ;
#43590=ORIENTED_EDGE ( 'NONE', *, *, #7959, .T. ) ;
#43591=CARTESIAN_POINT ( 'NONE',  ( -19.99999999999815969, 17.00000000000000000, 65.00000000000000000 ) ) ;
#43596=ORIENTED_EDGE ( 'NONE', *, *, #14357, .T. ) ;
#43604=VECTOR ( 'NONE', #37834, 1000.000000000000000 ) ;
#43613=DIRECTION ( 'NONE',  ( 0.000000000000000000, -0.000000000000000000, -1.000000000000000000 ) ) ;
#43617=ORIENTED_EDGE ( 'NONE', *, *, #15059, .T. ) ;
#43618=DIRECTION ( 'NONE',  ( -1.000000000000000000, -0.000000000000000000, -0.000000000000000000 ) ) ;
#43643=ORIENTED_EDGE ( 'NONE', *, *, #48063, .F. ) ;
#43645=VECTOR ( 'NONE', #6853, 1000.000000000000000 ) ;
#43646=DIRECTION ( 'NONE',  ( 1.000000000000000000, 0.000000000000000000, 0.000000000000000000 ) ) ;
#43659=EDGE_LOOP ( 'NONE', ( #42031, #13885, #42975, #50652 ) ) ;
#43660=VERTEX_POINT ( 'NONE', #14467 ) ;
#43663=CARTESIAN_POINT ( 'NONE',  ( 85.00000000000123634, 17.00000000000000000, 30.00000000000000000 ) ) ;
#43673=EDGE_LOOP ( 'NONE', ( #1718, #36446, #48003, #24568 ) ) ;
#43684=CARTESIAN_POINT ( 'NONE',  ( 0.000000000000000000, 17.00000000000000000, 0.000000000000000000 ) ) ;
#43707=EDGE_CURVE ( 'NONE', #30294, #48563, #4936, .T. ) ;
#43709=CARTESIAN_POINT ( 'NONE',  ( -19.99999999999940670, 17.00000000000000000, -54.99999999999999289 ) ) ;
#43710=CARTESIAN_POINT ( 'NONE',  ( -164.9999999999997442, 17.00000000000000000, -60.00000000000000000 ) ) ;
#43721=CARTESIAN_POINT ( 'NONE',  ( -114.9999999999987779, 17.00000000000000000, 5.000000000000004441 ) ) ;
#43726=VECTOR ( 'NONE', #21504, 1000.000000000000000 ) ;
#43728=ADVANCED_FACE ( 'NONE', ( #36776 ), #29810, .F. ) ;
#43731=ORIENTED_EDGE ( 'NONE', *, *, #27508, .T. ) ;
#43749=ORIENTED_EDGE ( 'NONE', *, *, #46269, .T. ) ;
#43751=EDGE_CURVE ( 'NONE', #41868, #37688, #44426, .T. ) ;
#43759=VECTOR ( 'NONE', #44787, 1000.000000000000000 ) ;
#43763=VECTOR ( 'NONE', #33639, 1000.000000000000000 ) ;
#43764=PLANE ( 'NONE',  #32435 ) ;
#43774=LINE ( 'NONE', #8881, #28300 ) ;
#43779=ORIENTED_EDGE ( 'NONE', *, *, #18370, .F. ) ;
#43792=DIRECTION ( 'NONE',  ( 0.000000000000000000, 0.000000000000000000, 1.000000000000000000 ) ) ;
#43793=VECTOR ( 'NONE', #45348, 1000.000000000000000 ) ;
#43795=CARTESIAN_POINT ( 'NONE',  ( -69.99999999999816680, 17.00000000000000000, 65.00000000000000000 ) ) ;
#43797=AXIS2_PLACEMENT_3D ( 'NONE', #3610, #23625, #39041 ) ;
#43810=ORIENTED_EDGE ( 'NONE', *, *, #12788, .T. ) ;
#43821=DIRECTION ( 'NONE',  ( 0.000000000000000000, -0.000000000000000000, -1.000000000000000000 ) ) ;
#43825=EDGE_CURVE ( 'NONE', #27084, #15777, #37291, .T. ) ;
#43831=CARTESIAN_POINT ( 'NONE',  ( 135.0000000000012790, 17.00000000000000000, 30.00000000000000000 ) ) ;
#43840=CARTESIAN_POINT ( 'NONE',  ( 85.00000000000090949, 17.00000000000000000, -24.99999999999999289 ) ) ;
#43842=CARTESIAN_POINT ( 'NONE',  ( 130.0000000000015064, 17.00000000000000000, 60.00000000000000000 ) ) ;
#43850=ORIENTED_EDGE ( 'NONE', *, *, #16717, .T. ) ;
#43852=CARTESIAN_POINT ( 'NONE',  ( 175.0000000000000000, 0.000000000000000000, -122.5000000000000000 ) ) ;
#43856=CARTESIAN_POINT ( 'NONE',  ( -119.9999999999987921, 17.00000000000000000, 5.000000000000004441 ) ) ;
#43865=AXIS2_PLACEMENT_3D ( 'NONE', #45242, #6525, #10387 ) ;
#43874=EDGE_CURVE ( 'NONE', #32522, #20901, #41859, .T. ) ;
#43879=ORIENTED_EDGE ( 'NONE', *, *, #26579, .F. ) ;
#43888=CARTESIAN_POINT ( 'NONE',  ( -165.0000000000000284, 16.00000000000000000, -114.9999999999999858 ) ) ;
#43891=CARTESIAN_POINT ( 'NONE',  ( -14.99999999999970868, 16.00000000000000000, -60.00000000000000000 ) ) ;
#43934=VECTOR ( 'NONE', #28422, 1000.000000000000000 ) ;
#43948=DIRECTION ( 'NONE',  ( 0.000000000000000000, 0.000000000000000000, -1.000000000000000000 ) ) ;
#43950=LINE ( 'NONE', #17268, #32413 ) ;
#43951=DIRECTION ( 'NONE',  ( -0.000000000000000000, -1.000000000000000000, -0.000000000000000000 ) ) ;
#43953=CARTESIAN_POINT ( 'NONE',  ( 85.00000000000184741, 16.00000000000000000, 65.00000000000000000 ) ) ;
#43955=DIRECTION ( 'NONE',  ( 4.625929269271687073E-16, -0.000000000000000000, 1.000000000000000000 ) ) ;
#43956=CARTESIAN_POINT ( 'NONE',  ( 80.00000000000061107, 16.00000000000000000, -30.00000000000000000 ) ) ;
#43978=ORIENTED_EDGE ( 'NONE', *, *, #24902, .T. ) ;
#43985=ORIENTED_EDGE ( 'NONE', *, *, #15969, .F. ) ;
#43993=ORIENTED_EDGE ( 'NONE', *, *, #6089, .T. ) ;
#44012=LINE ( 'NONE', #19914, #45947 ) ;
#44024=LINE ( 'NONE', #17094, #2443 ) ;
#44033=ORIENTED_EDGE ( 'NONE', *, *, #36688, .F. ) ;
#44047=EDGE_LOOP ( 'NONE', ( #50673, #32540, #22112, #29562 ) ) ;
#44064=AXIS2_PLACEMENT_3D ( 'NONE', #19416, #31744, #34835 ) ;
#44067=FACE_OUTER_BOUND ( 'NONE', #49571, .T. ) ;
#44082=FACE_OUTER_BOUND ( 'NONE', #38565, .T. ) ;
#44087=DIRECTION ( 'NONE',  ( 0.000000000000000000, 0.000000000000000000, 1.000000000000000000 ) ) ;
#44088=EDGE_LOOP ( 'NONE', ( #23194, #36835, #18605, #3010 ) ) ;
#44092=AXIS2_PLACEMENT_3D ( 'NONE', #44940, #44698, #40870 ) ;
#44101=ORIENTED_EDGE ( 'NONE', *, *, #19397, .F. ) ;
#44107=FACE_OUTER_BOUND ( 'NONE', #35542, .T. ) ;
#44109=LINE ( 'NONE', #21281, #5725 ) ;
#44136=ORIENTED_EDGE ( 'NONE', *, *, #47320, .F. ) ;
#44137=LINE ( 'NONE', #27996, #23076 ) ;
#44145=ORIENTED_EDGE ( 'NONE', *, *, #38656, .T. ) ;
#44159=LINE ( 'NONE', #4917, #40974 ) ;
#44160=CARTESIAN_POINT ( 'NONE',  ( -115.0000000000000284, 17.00000000000000000, -90.00000000000000000 ) ) ;
#44178=EDGE_CURVE ( 'NONE', #14334, #907, #41048, .T. ) ;
#44187=CARTESIAN_POINT ( 'NONE',  ( -14.99999999999906919, 16.00000000000000000, 0.000000000000000000 ) ) ;
#44191=EDGE_LOOP ( 'NONE', ( #7695, #1152, #26749, #11936 ) ) ;
#44193=DIRECTION ( 'NONE',  ( -1.000000000000000000, -0.000000000000000000, -0.000000000000000000 ) ) ;
#44198=ORIENTED_EDGE ( 'NONE', *, *, #36560, .F. ) ;
#44207=CARTESIAN_POINT ( 'NONE',  ( 84.99999999999997158, 17.00000000000000000, -90.00000000000000000 ) ) ;
#44217=DIRECTION ( 'NONE',  ( -0.000000000000000000, -1.000000000000000000, -0.000000000000000000 ) ) ;
#44224=ORIENTED_EDGE ( 'NONE', *, *, #11386, .T. ) ;
#44238=ORIENTED_EDGE ( 'NONE', *, *, #40565, .T. ) ;
#44240=ADVANCED_FACE ( 'NONE', ( #22800, #14595, #26660, #14085, #46110, #22297, #49201, #42047, #7423, #45363, #2544, #22546, #38723, #30013, #49453, #6395, #33609, #15108, #49951, #18186, #38482, #18439, #50196, #34617, #14855, #10253, #38233, #25911, #46380, #29749, #10499 ), #14341, .F. ) ;
#44251=CARTESIAN_POINT ( 'NONE',  ( -165.0000000000000284, 16.00000000000000000, -24.99999999999999289 ) ) ;
#44252=DIRECTION ( 'NONE',  ( -1.000000000000000000, -0.000000000000000000, -0.000000000000000000 ) ) ;
#44263=LINE ( 'NONE', #681, #15188 ) ;
#44264=CARTESIAN_POINT ( 'NONE',  ( 84.99999999999997158, 17.00000000000000000, -90.00000000000000000 ) ) ;
#44268=VECTOR ( 'NONE', #3381, 1000.000000000000000 ) ;
#44272=CARTESIAN_POINT ( 'NONE',  ( 0.000000000000000000, 17.00000000000000000, 0.000000000000000000 ) ) ;
#44273=LINE ( 'NONE', #39707, #11894 ) ;
#44285=PLANE ( 'NONE',  #5455 ) ;
#44289=LINE ( 'NONE', #36655, #43097 ) ;
#44292=DIRECTION ( 'NONE',  ( 0.000000000000000000, -0.000000000000000000, -1.000000000000000000 ) ) ;
#44295=ORIENTED_EDGE ( 'NONE', *, *, #30614, .T. ) ;
#44298=EDGE_CURVE ( 'NONE', #27596, #5585, #37975, .T. ) ;
#44306=VECTOR ( 'NONE', #12872, 1000.000000000000000 ) ;
#44311=DIRECTION ( 'NONE',  ( 1.000000000000000000, 0.000000000000000000, -0.000000000000000000 ) ) ;
#44316=DIRECTION ( 'NONE',  ( 0.000000000000000000, 0.000000000000000000, 1.000000000000000000 ) ) ;
#44322=EDGE_CURVE ( 'NONE', #19392, #7505, #16372, .T. ) ;
#44324=CARTESIAN_POINT ( 'NONE',  ( -115.0000000000000284, 17.00000000000000000, -90.00000000000000000 ) ) ;
#44328=ADVANCED_FACE ( 'NONE', ( #31790 ), #46618, .F. ) ;
#44331=EDGE_CURVE ( 'NONE', #35777, #32189, #24347, .T. ) ;
#44332=DIRECTION ( 'NONE',  ( -0.000000000000000000, -1.000000000000000000, -0.000000000000000000 ) ) ;
#44334=CARTESIAN_POINT ( 'NONE',  ( 164.9999999999999716, 17.00000000000000000, -60.00000000000001421 ) ) ;
#44336=ADVANCED_FACE ( 'NONE', ( #20225 ), #3813, .F. ) ;
#44339=VERTEX_POINT ( 'NONE', #43308 ) ;
#44346=LINE ( 'NONE', #1778, #11159 ) ;
#44358=EDGE_LOOP ( 'NONE', ( #43749, #32446, #9377, #32085 ) ) ;
#44360=ORIENTED_EDGE ( 'NONE', *, *, #21238, .T. ) ;
#44361=LINE ( 'NONE', #21036, #27866 ) ;
#44362=LINE ( 'NONE', #20529, #42221 ) ;
#44383=LINE ( 'NONE', #24914, #3404 ) ;
#44385=FACE_OUTER_BOUND ( 'NONE', #42668, .T. ) ;
#44386=CARTESIAN_POINT ( 'NONE',  ( -14.99999999999845812, 17.00000000000000000, 60.00000000000000000 ) ) ;
#44397=CARTESIAN_POINT ( 'NONE',  ( 130.0000000000018474, 16.00000000000000000, 65.00000000000000000 ) ) ;
#44403=CARTESIAN_POINT ( 'NONE',  ( -164.9999999999994031, 17.00000000000000000, -54.99999999999999289 ) ) ;
#44422=CARTESIAN_POINT ( 'NONE',  ( 175.0000000000000000, 15.00000000000000000, 122.5000000000000142 ) ) ;
#44426=LINE ( 'NONE', #48252, #43582 ) ;
#44431=DIRECTION ( 'NONE',  ( -0.000000000000000000, -0.000000000000000000, -1.000000000000000000 ) ) ;
#44433=CARTESIAN_POINT ( 'NONE',  ( 135.0000000000015632, 17.00000000000000000, 60.00000000000000000 ) ) ;
#44445=VECTOR ( 'NONE', #18564, 1000.000000000000000 ) ;
#44452=VECTOR ( 'NONE', #9977, 1000.000000000000000 ) ;
#44456=DIRECTION ( 'NONE',  ( -0.000000000000000000, -1.000000000000000000, -0.000000000000000000 ) ) ;
#44457=EDGE_CURVE ( 'NONE', #22853, #25007, #41424, .T. ) ;
#44467=EDGE_LOOP ( 'NONE', ( #40065, #25968, #30167, #46311 ) ) ;
#44470=FACE_OUTER_BOUND ( 'NONE', #5977, .T. ) ;
#44477=FACE_OUTER_BOUND ( 'NONE', #20880, .T. ) ;
#44486=EDGE_LOOP ( 'NONE', ( #22329, #6496, #17750, #25257 ) ) ;
#44508=VECTOR ( 'NONE', #26857, 1000.000000000000000 ) ;
#44515=DIRECTION ( 'NONE',  ( 0.000000000000000000, 0.000000000000000000, 1.000000000000000000 ) ) ;
#44522=ORIENTED_EDGE ( 'NONE', *, *, #22506, .T. ) ;
#44524=PLANE ( 'NONE',  #49986 ) ;
#44525=ORIENTED_EDGE ( 'NONE', *, *, #40619, .F. ) ;
#44529=ORIENTED_EDGE ( 'NONE', *, *, #45267, .F. ) ;
#44540=ORIENTED_EDGE ( 'NONE', *, *, #46790, .T. ) ;
#44545=CARTESIAN_POINT ( 'NONE',  ( -164.9999999999987779, 17.00000000000000000, 30.00000000000000000 ) ) ;
#44556=VERTEX_POINT ( 'NONE', #17132 ) ;
#44567=LINE ( 'NONE', #43591, #18890 ) ;
#44571=DIRECTION ( 'NONE',  ( -1.000000000000000000, 0.000000000000000000, 0.000000000000000000 ) ) ;
#44584=EDGE_CURVE ( 'NONE', #21400, #46071, #19586, .T. ) ;
#44590=ADVANCED_FACE ( 'NONE', ( #27300 ), #38351, .F. ) ;
#44592=EDGE_LOOP ( 'NONE', ( #4700, #4063, #2874, #50381 ) ) ;
#44599=DIRECTION ( 'NONE',  ( 0.000000000000000000, 0.000000000000000000, -1.000000000000000000 ) ) ;
#44608=EDGE_CURVE ( 'NONE', #21378, #22127, #14984, .T. ) ;
#44625=CARTESIAN_POINT ( 'NONE',  ( 0.000000000000000000, 17.00000000000000000, 0.000000000000000000 ) ) ;
#44645=DIRECTION ( 'NONE',  ( 0.000000000000000000, 0.000000000000000000, 1.000000000000000000 ) ) ;
#44650=AXIS2_PLACEMENT_3D ( 'NONE', #16367, #31785, #46868 ) ;
#44651=CARTESIAN_POINT ( 'NONE',  ( 135.0000000000009663, 17.00000000000000000, -24.99999999999999289 ) ) ;
#44656=AXIS2_PLACEMENT_3D ( 'NONE', #33051, #8936, #44311 ) ;
#44675=ORIENTED_EDGE ( 'NONE', *, *, #9663, .F. ) ;
#44686=ADVANCED_FACE ( 'NONE', ( #364 ), #31674, .F. ) ;
#44695=CARTESIAN_POINT ( 'NONE',  ( 130.0000000000018474, 17.00000000000000000, 65.00000000000000000 ) ) ;
#44698=DIRECTION ( 'NONE',  ( 1.000000000000000000, 0.000000000000000000, 0.000000000000000000 ) ) ;
#44700=AXIS2_PLACEMENT_3D ( 'NONE', #30193, #6594, #21992 ) ;
#44701=VECTOR ( 'NONE', #10412, 1000.000000000000000 ) ;
#44725=VERTEX_POINT ( 'NONE', #12395 ) ;
#44727=LINE ( 'NONE', #1658, #20874 ) ;
#44729=CARTESIAN_POINT ( 'NONE',  ( 80.00000000000216005, 17.00000000000000000, 95.00000000000000000 ) ) ;
#44735=VECTOR ( 'NONE', #11566, 1000.000000000000000 ) ;
#44736=DIRECTION ( 'NONE',  ( 0.000000000000000000, 0.000000000000000000, 1.000000000000000000 ) ) ;
#44746=ORIENTED_EDGE ( 'NONE', *, *, #43451, .F. ) ;
#44756=VECTOR ( 'NONE', #32392, 1000.000000000000000 ) ;
#44758=VECTOR ( 'NONE', #43122, 1000.000000000000000 ) ;
#44765=VECTOR ( 'NONE', #3096, 1000.000000000000000 ) ;
#44769=LINE ( 'NONE', #28394, #23870 ) ;
#44777=ORIENTED_EDGE ( 'NONE', *, *, #19260, .T. ) ;
#44787=DIRECTION ( 'NONE',  ( 0.000000000000000000, 0.000000000000000000, -1.000000000000000000 ) ) ;
#44807=EDGE_CURVE ( 'NONE', #30535, #15604, #37539, .T. ) ;
#44816=LINE ( 'NONE', #48390, #5381 ) ;
#44821=ORIENTED_EDGE ( 'NONE', *, *, #43078, .F. ) ;
#44824=CARTESIAN_POINT ( 'NONE',  ( 30.00000000000062172, 16.00000000000000000, -54.99999999999999289 ) ) ;
#44827=DIRECTION ( 'NONE',  ( -1.000000000000000000, 0.000000000000000000, 0.000000000000000000 ) ) ;
#44828=ORIENTED_EDGE ( 'NONE', *, *, #8935, .F. ) ;
#44836=EDGE_CURVE ( 'NONE', #19934, #50192, #6223, .T. ) ;
#44837=LINE ( 'NONE', #23420, #37713 ) ;
#44838=ORIENTED_EDGE ( 'NONE', *, *, #3049, .F. ) ;
#44839=CARTESIAN_POINT ( 'NONE',  ( -70.00000000000002842, 17.00000000000000000, -90.00000000000000000 ) ) ;
#44862=ORIENTED_EDGE ( 'NONE', *, *, #49313, .T. ) ;
#44864=LINE ( 'NONE', #5894, #5445 ) ;
#44869=ORIENTED_EDGE ( 'NONE', *, *, #30408, .T. ) ;
#44876=DIRECTION ( 'NONE',  ( 0.000000000000000000, -0.000000000000000000, -1.000000000000000000 ) ) ;
#44890=DIRECTION ( 'NONE',  ( 1.000000000000000000, 0.000000000000000000, -9.251858538542979716E-16 ) ) ;
#44899=CARTESIAN_POINT ( 'NONE',  ( 85.00000000000213163, 17.00000000000000000, 95.00000000000000000 ) ) ;
#44903=VERTEX_POINT ( 'NONE', #44433 ) ;
#44912=CARTESIAN_POINT ( 'NONE',  ( 35.00000000000152767, 17.00000000000000000, 60.00000000000000000 ) ) ;
#44915=VECTOR ( 'NONE', #32501, 1000.000000000000000 ) ;
#44917=ORIENTED_EDGE ( 'NONE', *, *, #1503, .T. ) ;
#44928=ORIENTED_EDGE ( 'NONE', *, *, #39938, .F. ) ;
#44935=DIRECTION ( 'NONE',  ( -1.000000000000000000, 0.000000000000000000, -0.000000000000000000 ) ) ;
#44940=CARTESIAN_POINT ( 'NONE',  ( -65.00000000000002842, 17.00000000000000000, -114.9999999999999858 ) ) ;
#44951=VECTOR ( 'NONE', #47581, 1000.000000000000000 ) ;
#44954=VECTOR ( 'NONE', #32056, 1000.000000000000000 ) ;
#44966=FACE_OUTER_BOUND ( 'NONE', #14393, .T. ) ;
#44971=DIRECTION ( 'NONE',  ( 1.000000000000000000, 0.000000000000000000, 0.000000000000000000 ) ) ;
#44978=EDGE_CURVE ( 'NONE', #50236, #25157, #14665, .T. ) ;
#44982=EDGE_CURVE ( 'NONE', #42338, #16052, #11068, .T. ) ;
#44985=DIRECTION ( 'NONE',  ( -1.000000000000000000, 0.000000000000000000, -0.000000000000000000 ) ) ;
#44987=ORIENTED_EDGE ( 'NONE', *, *, #30744, .F. ) ;
#44994=CARTESIAN_POINT ( 'NONE',  ( 164.9999999999999716, 17.00000000000000000, -25.00000000000000711 ) ) ;
#44995=CARTESIAN_POINT ( 'NONE',  ( -164.9999999999981526, 17.00000000000000000, 65.00000000000000000 ) ) ;
#45004=AXIS2_PLACEMENT_3D ( 'NONE', #27135, #34849, #42753 ) ;
#45009=LINE ( 'NONE', #17590, #40163 ) ;
#45014=ADVANCED_FACE ( 'NONE', ( #8757 ), #4140, .F. ) ;
#45018=FACE_OUTER_BOUND ( 'NONE', #13693, .T. ) ;
#45021=VERTEX_POINT ( 'NONE', #39553 ) ;
#45024=VECTOR ( 'NONE', #12551, 1000.000000000000000 ) ;
#45041=LINE ( 'NONE', #21713, #17720 ) ;
#45051=FACE_OUTER_BOUND ( 'NONE', #50171, .T. ) ;
#45052=ORIENTED_EDGE ( 'NONE', *, *, #49759, .F. ) ;
#45053=DIRECTION ( 'NONE',  ( 0.000000000000000000, -0.000000000000000000, -1.000000000000000000 ) ) ;
#45054=DIRECTION ( 'NONE',  ( 1.000000000000000000, 0.000000000000000000, 0.000000000000000000 ) ) ;
#45055=CARTESIAN_POINT ( 'NONE',  ( -14.99999999999782041, 17.00000000000000000, 115.0000000000000142 ) ) ;
#45062=VECTOR ( 'NONE', #45268, 1000.000000000000000 ) ;
#45064=AXIS2_PLACEMENT_3D ( 'NONE', #10087, #26494, #45702 ) ;
#45072=CARTESIAN_POINT ( 'NONE',  ( 164.9999999999999716, 17.00000000000000000, -90.00000000000002842 ) ) ;
#45073=ORIENTED_EDGE ( 'NONE', *, *, #30594, .T. ) ;
#45081=FACE_OUTER_BOUND ( 'NONE', #1236, .T. ) ;
#45086=ORIENTED_EDGE ( 'NONE', *, *, #7190, .F. ) ;
#45087=EDGE_CURVE ( 'NONE', #45549, #47156, #9243, .T. ) ;
#45091=CARTESIAN_POINT ( 'NONE',  ( 35.00000000000186162, 17.00000000000000000, 90.00000000000000000 ) ) ;
#45100=CARTESIAN_POINT ( 'NONE',  ( -114.9999999999984652, 17.00000000000000000, 35.00000000000000000 ) ) ;
#45101=VECTOR ( 'NONE', #45586, 1000.000000000000000 ) ;
#45110=VECTOR ( 'NONE', #39194, 1000.000000000000000 ) ;
#45117=CARTESIAN_POINT ( 'NONE',  ( -165.0000000000000284, 16.00000000000000000, 30.00000000000000000 ) ) ;
#45118=LINE ( 'NONE', #20784, #34156 ) ;
#45120=FACE_OUTER_BOUND ( 'NONE', #26693, .T. ) ;
#45126=CARTESIAN_POINT ( 'NONE',  ( -64.99999999999971578, 16.00000000000000000, -84.99999999999998579 ) ) ;
#45144=PLANE ( 'NONE',  #39268 ) ;
#45150=ADVANCED_FACE ( 'NONE', ( #45120 ), #28752, .F. ) ;
#45151=FACE_OUTER_BOUND ( 'NONE', #8743, .T. ) ;
#45157=LINE ( 'NONE', #14131, #25923 ) ;
#45160=CARTESIAN_POINT ( 'NONE',  ( -114.9999999999994031, 17.00000000000000000, -54.99999999999999289 ) ) ;
#45168=DIRECTION ( 'NONE',  ( 1.000000000000000000, 0.000000000000000000, -0.000000000000000000 ) ) ;
#45169=EDGE_LOOP ( 'NONE', ( #32321, #133, #32251, #5256 ) ) ;
#45178=ORIENTED_EDGE ( 'NONE', *, *, #6149, .T. ) ;
#45188=CARTESIAN_POINT ( 'NONE',  ( -114.9999999999997158, 17.00000000000000000, -84.99999999999998579 ) ) ;
#45205=CARTESIAN_POINT ( 'NONE',  ( -14.99999999999906919, 17.00000000000000000, -24.99999999999999289 ) ) ;
#45208=ORIENTED_EDGE ( 'NONE', *, *, #35505, .F. ) ;
#45212=CARTESIAN_POINT ( 'NONE',  ( 30.00000000000153833, 17.00000000000000000, 35.00000000000000000 ) ) ;
#45214=ORIENTED_EDGE ( 'NONE', *, *, #38656, .F. ) ;
#45216=DIRECTION ( 'NONE',  ( 0.000000000000000000, 0.000000000000000000, 1.000000000000000000 ) ) ;
#45225=DIRECTION ( 'NONE',  ( 0.000000000000000000, -1.000000000000000000, 0.000000000000000000 ) ) ;
#45232=VECTOR ( 'NONE', #33675, 1000.000000000000000 ) ;
#45238=ORIENTED_EDGE ( 'NONE', *, *, #14646, .T. ) ;
#45240=FACE_OUTER_BOUND ( 'NONE', #46467, .T. ) ;
#45242=CARTESIAN_POINT ( 'NONE',  ( -19.99999999999815969, 17.00000000000000000, 65.00000000000000000 ) ) ;
#45262=EDGE_CURVE ( 'NONE', #43085, #26536, #26668, .T. ) ;
#45265=CARTESIAN_POINT ( 'NONE',  ( -115.0000000000000284, 16.00000000000000000, -90.00000000000000000 ) ) ;
#45267=EDGE_CURVE ( 'NONE', #47621, #29419, #37726, .T. ) ;
#45268=DIRECTION ( 'NONE',  ( -0.000000000000000000, -0.000000000000000000, -1.000000000000000000 ) ) ;
#45285=ORIENTED_EDGE ( 'NONE', *, *, #37262, .F. ) ;
#45295=EDGE_CURVE ( 'NONE', #41417, #21137, #34372, .T. ) ;
#45296=ORIENTED_EDGE ( 'NONE', *, *, #15849, .F. ) ;
#45303=EDGE_CURVE ( 'NONE', #16866, #35257, #18947, .T. ) ;
#45305=EDGE_CURVE ( 'NONE', #27903, #8207, #7432, .T. ) ;
#45306=CARTESIAN_POINT ( 'NONE',  ( -14.99999999999970868, 16.00000000000000000, -60.00000000000000000 ) ) ;
#45311=ADVANCED_FACE ( 'NONE', ( #7679 ), #16379, .F. ) ;
#45312=DIRECTION ( 'NONE',  ( -1.000000000000000000, -0.000000000000000000, -0.000000000000000000 ) ) ;
#45317=FACE_OUTER_BOUND ( 'NONE', #33577, .T. ) ;
#45322=LINE ( 'NONE', #7119, #9902 ) ;
#45326=VERTEX_POINT ( 'NONE', #32047 ) ;
#45341=DIRECTION ( 'NONE',  ( 0.000000000000000000, 0.000000000000000000, -1.000000000000000000 ) ) ;
#45343=ADVANCED_FACE ( 'NONE', ( #39748 ), #35904, .F. ) ;
#45348=DIRECTION ( 'NONE',  ( 0.000000000000000000, 0.000000000000000000, -1.000000000000000000 ) ) ;
#45351=VERTEX_POINT ( 'NONE', #47890 ) ;
#45353=CARTESIAN_POINT ( 'NONE',  ( -64.99999999999971578, 16.00000000000000000, -84.99999999999998579 ) ) ;
#45354=ORIENTED_EDGE ( 'NONE', *, *, #16913, .T. ) ;
#45357=CARTESIAN_POINT ( 'NONE',  ( 135.0000000000019043, 16.00000000000000000, 90.00000000000000000 ) ) ;
#45358=CARTESIAN_POINT ( 'NONE',  ( -19.99999999999971223, 17.00000000000000000, -84.99999999999998579 ) ) ;
#45363=FACE_BOUND ( 'NONE', #27332, .T. ) ;
#45373=EDGE_LOOP ( 'NONE', ( #6471, #28106, #45086, #27658 ) ) ;
#45374=EDGE_CURVE ( 'NONE', #11508, #37527, #4335, .T. ) ;
#45382=DIRECTION ( 'NONE',  ( 0.000000000000000000, -1.000000000000000000, 0.000000000000000000 ) ) ;
#45387=LINE ( 'NONE', #6661, #4494 ) ;
#45399=VECTOR ( 'NONE', #46948, 1000.000000000000000 ) ;
#45406=DIRECTION ( 'NONE',  ( -0.000000000000000000, -0.000000000000000000, -1.000000000000000000 ) ) ;
#45413=VECTOR ( 'NONE', #15984, 1000.000000000000000 ) ;
#45422=CARTESIAN_POINT ( 'NONE',  ( 35.00000000000061107, 17.00000000000000000, -54.99999999999999289 ) ) ;
#45426=FACE_OUTER_BOUND ( 'NONE', #39093, .T. ) ;
#45476=VECTOR ( 'NONE', #43080, 1000.000000000000000 ) ;
#45478=PLANE ( 'NONE',  #17767 ) ;
#45482=CARTESIAN_POINT ( 'NONE',  ( 164.9999999999999716, 15.00000000000000000, -114.9999999999999858 ) ) ;
#45483=CARTESIAN_POINT ( 'NONE',  ( 80.00000000000092371, 17.00000000000000000, -24.99999999999999289 ) ) ;
#45486=AXIS2_PLACEMENT_3D ( 'NONE', #31923, #7813, #35026 ) ;
#45492=EDGE_LOOP ( 'NONE', ( #13452, #42855, #44136, #8861 ) ) ;
#45495=AXIS2_PLACEMENT_3D ( 'NONE', #32799, #29199, #43821 ) ;
#45496=CARTESIAN_POINT ( 'NONE',  ( 35.00000000000061107, 16.00000000000000000, -54.99999999999999289 ) ) ;
#45501=LINE ( 'NONE', #18073, #49735 ) ;
#45511=VECTOR ( 'NONE', #18484, 1000.000000000000000 ) ;
#45512=DIRECTION ( 'NONE',  ( 1.000000000000000000, 0.000000000000000000, 0.000000000000000000 ) ) ;
#45520=LINE ( 'NONE', #10402, #31239 ) ;
#45538=VERTEX_POINT ( 'NONE', #9435 ) ;
#45544=VECTOR ( 'NONE', #45723, 1000.000000000000000 ) ;
#45547=AXIS2_PLACEMENT_3D ( 'NONE', #1597, #40597, #37279 ) ;
#45549=VERTEX_POINT ( 'NONE', #24589 ) ;
#45552=CARTESIAN_POINT ( 'NONE',  ( 84.99999999999997158, 17.00000000000000000, -114.9999999999999858 ) ) ;
#45555=VERTEX_POINT ( 'NONE', #5070 ) ;
#45561=DIRECTION ( 'NONE',  ( -0.000000000000000000, -1.000000000000000000, -0.000000000000000000 ) ) ;
#45570=CARTESIAN_POINT ( 'NONE',  ( -14.99999999999970868, 17.00000000000000000, -84.99999999999998579 ) ) ;
#45572=EDGE_CURVE ( 'NONE', #25937, #13970, #19145, .T. ) ;
#45574=DIRECTION ( 'NONE',  ( 0.000000000000000000, 0.000000000000000000, -1.000000000000000000 ) ) ;
#45577=DIRECTION ( 'NONE',  ( 0.000000000000000000, -1.000000000000000000, 0.000000000000000000 ) ) ;
#45581=DIRECTION ( 'NONE',  ( -1.000000000000000000, -0.000000000000000000, -0.000000000000000000 ) ) ;
#45583=CARTESIAN_POINT ( 'NONE',  ( 85.00000000000213163, 17.00000000000000000, 95.00000000000000000 ) ) ;
#45585=DIRECTION ( 'NONE',  ( 1.000000000000000000, 0.000000000000000000, -9.251858538542979716E-16 ) ) ;
#45586=DIRECTION ( 'NONE',  ( 0.000000000000000000, 0.000000000000000000, 1.000000000000000000 ) ) ;
#45593=VERTEX_POINT ( 'NONE', #37665 ) ;
#45598=VERTEX_POINT ( 'NONE', #46059 ) ;
#45603=PLANE ( 'NONE',  #9218 ) ;
#45604=EDGE_CURVE ( 'NONE', #41095, #22082, #18883, .T. ) ;
#45606=VERTEX_POINT ( 'NONE', #3236 ) ;
#45609=DIRECTION ( 'NONE',  ( 0.000000000000000000, 0.000000000000000000, -1.000000000000000000 ) ) ;
#45611=DIRECTION ( 'NONE',  ( 0.000000000000000000, -1.000000000000000000, 0.000000000000000000 ) ) ;
#45615=VERTEX_POINT ( 'NONE', #10951 ) ;
#45616=PLANE ( 'NONE',  #9827 ) ;
#45619=ADVANCED_FACE ( 'NONE', ( #42250 ), #26606, .F. ) ;
#45622=EDGE_CURVE ( 'NONE', #18731, #302, #30719, .T. ) ;
#45625=EDGE_CURVE ( 'NONE', #42991, #27084, #26092, .T. ) ;
#45641=FACE_OUTER_BOUND ( 'NONE', #47283, .T. ) ;
#45649=FACE_OUTER_BOUND ( 'NONE', #15226, .T. ) ;
#45656=CARTESIAN_POINT ( 'NONE',  ( 135.0000000000015632, 16.00000000000000000, 35.00000000000000000 ) ) ;
#45680=EDGE_LOOP ( 'NONE', ( #16403, #38276, #30687, #6062 ) ) ;
#45698=ORIENTED_EDGE ( 'NONE', *, *, #49060, .T. ) ;
#45702=DIRECTION ( 'NONE',  ( 0.000000000000000000, -0.000000000000000000, -1.000000000000000000 ) ) ;
#45703=DIRECTION ( 'NONE',  ( -0.000000000000000000, -0.000000000000000000, -1.000000000000000000 ) ) ;
#45713=ORIENTED_EDGE ( 'NONE', *, *, #39100, .T. ) ;
#45723=DIRECTION ( 'NONE',  ( -0.000000000000000000, -1.000000000000000000, -0.000000000000000000 ) ) ;
#45724=CARTESIAN_POINT ( 'NONE',  ( -165.0000000000000284, 17.00000000000000000, -90.00000000000000000 ) ) ;
#45726=DIRECTION ( 'NONE',  ( 1.000000000000000000, 0.000000000000000000, 0.000000000000000000 ) ) ;
#45728=ORIENTED_EDGE ( 'NONE', *, *, #39396, .F. ) ;
#45729=CLOSED_SHELL ( 'NONE', ( #44240, #31802, #22064, #35000, #9328, #9934, #42420, #32460, #22620, #15668, #10745, #34633, #43427, #774, #22845, #11394, #41899, #32137, #41999, #235, #31906, #25404, #47925, #41187, #1986, #4861, #11327, #26242, #10228, #11127, #20619, #8879, #34027, #21534, #35699, #45619, #32134, #2156, #17349, #22808, #5832, #15596, #37283, #46428, #37333, #5089, #11296, #44328, #40328, #22395, #26483, #22182, #5969, #41919, #9535, #18753, #30010, #1386, #22302, #30530, #25031, #2934, #14509, #48088, #42479, #26201, #9384, #33771, #27440, #24331, #15136, #39449, #180, #28718, #17038, #3705, #20267, #15923, #7657, #42392, #40132, #37815, #19096, #12021, #36823, #44336, #34768, #25035, #50663, #31885, #31927, #42419, #49655, #5149, #29175, #11375, #26294, #46398, #7668, #41496, #2340, #26153, #9323, #30242, #21470, #44590, #13344, #31647, #49477, #41256, #40444, #35309, #941, #16912, #14365, #31328, #45311, #31487, #28442, #26852, #11979, #28282, #27126, #19826, #10935, #43257, #7655, #49051, #41978, #46867, #36481, #12444, #12142, #34776, #13367, #40627, #14197, #28080, #24930, #48955, #50692, #17296, #6184, #34997, #4053, #47509, #43140, #10576, #36049, #14592, #42614, #12022, #18967, #10007, #43728, #29354, #21243, #47081, #38833, #30926, #30854, #35838, #42311, #45150, #41976, #20958, #29057, #553, #21285, #18284, #43418, #41529, #32115, #29490, #47725, #22520, #28969, #29923, #46510, #21757, #10173, #1691, #37495, #8315, #47157, #4859, #48385, #42495, #49220, #30198, #8939, #24027, #11517, #20514, #8870, #45343, #42140, #33682, #29706, #12197, #35117, #44686, #11866, #17133, #16279, #31057, #32694, #1697, #18265, #41537, #4689, #10971, #34714, #2756, #12398, #45014, #34616, #7692, #34402, #4649, #22138, #465, #4798, #22872, #20028, #23356, #6900, #33148, #21544, #6039, #32139, #39747, #22274, #46832, #32171, #8339, #46550, #41101, #47059, #10403, #24950, #17773, #41787, #26475, #31567, #32270, #30871, #33071, #5125, #12685, #34335, #39240, #22811, #11010, #24111, #437, #3141, #17730, #32779, #20680, #36836 ) ) ;
#45730=LINE ( 'NONE', #10611, #17670 ) ;
#45738=CARTESIAN_POINT ( 'NONE',  ( -14.99999999999906919, 16.00000000000000000, -24.99999999999999289 ) ) ;
#45739=ORIENTED_EDGE ( 'NONE', *, *, #49313, .F. ) ;
#45756=AXIS2_PLACEMENT_3D ( 'NONE', #18015, #25224, #21887 ) ;
#45768=VECTOR ( 'NONE', #22081, 1000.000000000000000 ) ;
#45775=EDGE_LOOP ( 'NONE', ( #10205, #23101, #15105, #4437, #31308, #48707, #4702, #49068, #13995, #6755, #37676, #29744, #23073, #40771, #41342, #47756, #36819, #20664, #4454, #7528, #30903, #48281, #45739, #6506, #10410, #16288, #33879, #23105 ) ) ;
#45777=DIRECTION ( 'NONE',  ( 0.000000000000000000, 0.000000000000000000, -1.000000000000000000 ) ) ;
#45778=ORIENTED_EDGE ( 'NONE', *, *, #15005, .T. ) ;
#45786=DIRECTION ( 'NONE',  ( 0.000000000000000000, 0.000000000000000000, -1.000000000000000000 ) ) ;
#45809=DIRECTION ( 'NONE',  ( 0.000000000000000000, 0.000000000000000000, -1.000000000000000000 ) ) ;
#45811=CARTESIAN_POINT ( 'NONE',  ( -14.99999999999876366, 17.00000000000000000, 5.000000000000004441 ) ) ;
#45816=AXIS2_PLACEMENT_3D ( 'NONE', #13788, #44827, #49161 ) ;
#45817=ORIENTED_EDGE ( 'NONE', *, *, #36613, .F. ) ;
#45825=DIRECTION ( 'NONE',  ( 0.000000000000000000, 0.000000000000000000, -1.000000000000000000 ) ) ;
#45830=DIRECTION ( 'NONE',  ( -0.000000000000000000, -1.000000000000000000, -0.000000000000000000 ) ) ;
#45845=ORIENTED_EDGE ( 'NONE', *, *, #94, .T. ) ;
#45864=VERTEX_POINT ( 'NONE', #5277 ) ;
#45865=CARTESIAN_POINT ( 'NONE',  ( 135.0000000000003411, 17.00000000000000000, -84.99999999999998579 ) ) ;
#45868=AXIS2_PLACEMENT_3D ( 'NONE', #34119, #23303, #18940 ) ;
#45882=DIRECTION ( 'NONE',  ( 1.000000000000000000, 0.000000000000000000, 0.000000000000000000 ) ) ;
#45899=VECTOR ( 'NONE', #9342, 1000.000000000000000 ) ;
#45905=ORIENTED_EDGE ( 'NONE', *, *, #3388, .T. ) ;
#45916=CARTESIAN_POINT ( 'NONE',  ( 34.99999999999997868, 17.00000000000000000, -90.00000000000000000 ) ) ;
#45934=ORIENTED_EDGE ( 'NONE', *, *, #50162, .T. ) ;
#45947=VECTOR ( 'NONE', #12468, 1000.000000000000000 ) ;
#45968=VERTEX_POINT ( 'NONE', #41943 ) ;
#45980=CARTESIAN_POINT ( 'NONE',  ( 0.000000000000000000, 17.00000000000000000, 0.000000000000000000 ) ) ;
#45984=ORIENTED_EDGE ( 'NONE', *, *, #49889, .T. ) ;
#45985=ORIENTED_EDGE ( 'NONE', *, *, #934, .F. ) ;
#45989=ORIENTED_EDGE ( 'NONE', *, *, #38192, .T. ) ;
#45991=ORIENTED_EDGE ( 'NONE', *, *, #16747, .F. ) ;
#46000=EDGE_CURVE ( 'NONE', #1528, #16006, #33753, .T. ) ;
#46004=DIRECTION ( 'NONE',  ( 1.000000000000000000, 0.000000000000000000, -0.000000000000000000 ) ) ;
#46023=CARTESIAN_POINT ( 'NONE',  ( -165.0000000000000284, 16.00000000000000000, 115.0000000000000142 ) ) ;
#46040=LINE ( 'NONE', #31208, #4472 ) ;
#46044=DIRECTION ( 'NONE',  ( 0.000000000000000000, 0.000000000000000000, 1.000000000000000000 ) ) ;
#46053=PLANE ( 'NONE',  #27780 ) ;
#46059=CARTESIAN_POINT ( 'NONE',  ( 85.00000000000152056, 17.00000000000000000, 60.00000000000000000 ) ) ;
#46071=VERTEX_POINT ( 'NONE', #24417 ) ;
#46076=DIRECTION ( 'NONE',  ( -1.000000000000000000, -0.000000000000000000, -0.000000000000000000 ) ) ;
#46083=ORIENTED_EDGE ( 'NONE', *, *, #19485, .T. ) ;
#46085=ORIENTED_EDGE ( 'NONE', *, *, #20229, .F. ) ;
#46092=LINE ( 'NONE', #18672, #44452 ) ;
#46096=DIRECTION ( 'NONE',  ( -1.000000000000000000, -0.000000000000000000, -0.000000000000000000 ) ) ;
#46100=VECTOR ( 'NONE', #10710, 1000.000000000000000 ) ;
#46110=FACE_BOUND ( 'NONE', #18334, .T. ) ;
#46124=EDGE_CURVE ( 'NONE', #15741, #44725, #13096, .T. ) ;
#46132=CARTESIAN_POINT ( 'NONE',  ( -119.9999999999997158, 17.00000000000000000, -60.00000000000000000 ) ) ;
#46139=DIRECTION ( 'NONE',  ( -0.000000000000000000, -0.000000000000000000, -1.000000000000000000 ) ) ;
#46140=ORIENTED_EDGE ( 'NONE', *, *, #6691, .T. ) ;
#46144=ORIENTED_EDGE ( 'NONE', *, *, #8929, .T. ) ;
#46146=LINE ( 'NONE', #2575, #24869 ) ;
#46152=EDGE_CURVE ( 'NONE', #16567, #593, #38618, .T. ) ;
#46168=CARTESIAN_POINT ( 'NONE',  ( -164.9999999999987779, 16.00000000000000000, 5.000000000000004441 ) ) ;
#46173=VECTOR ( 'NONE', #19440, 1000.000000000000000 ) ;
#46181=VERTEX_POINT ( 'NONE', #49467 ) ;
#46187=EDGE_CURVE ( 'NONE', #17726, #32522, #9498, .T. ) ;
#46190=DIRECTION ( 'NONE',  ( 0.000000000000000000, -1.000000000000000000, 0.000000000000000000 ) ) ;
#46191=ORIENTED_EDGE ( 'NONE', *, *, #34223, .T. ) ;
#46199=VECTOR ( 'NONE', #19661, 1000.000000000000000 ) ;
#46200=EDGE_LOOP ( 'NONE', ( #26249, #15283, #25965, #22424 ) ) ;
#46211=VECTOR ( 'NONE', #9105, 1000.000000000000000 ) ;
#46219=CARTESIAN_POINT ( 'NONE',  ( -164.9999999999994031, 16.00000000000000000, -54.99999999999999289 ) ) ;
#46223=EDGE_CURVE ( 'NONE', #46923, #11032, #40557, .T. ) ;
#46233=ORIENTED_EDGE ( 'NONE', *, *, #23647, .T. ) ;
#46234=EDGE_CURVE ( 'NONE', #17047, #1405, #6161, .T. ) ;
#46248=EDGE_LOOP ( 'NONE', ( #37938, #16074, #34354, #50712 ) ) ;
#46252=PLANE ( 'NONE',  #10548 ) ;
#46264=CARTESIAN_POINT ( 'NONE',  ( 130.0000000000008811, 17.00000000000000000, 0.000000000000000000 ) ) ;
#46269=EDGE_CURVE ( 'NONE', #9554, #33142, #18455, .T. ) ;
#46271=CARTESIAN_POINT ( 'NONE',  ( 35.00000000000028422, 16.00000000000000000, -84.99999999999998579 ) ) ;
#46280=EDGE_CURVE ( 'NONE', #25760, #31020, #7685, .T. ) ;
#46282=EDGE_LOOP ( 'NONE', ( #42904, #18721, #18477, #13817 ) ) ;
#46283=CARTESIAN_POINT ( 'NONE',  ( -119.9999999999981668, 17.00000000000000000, 90.00000000000000000 ) ) ;
#46295=LINE ( 'NONE', #10922, #12766 ) ;
#46297=CARTESIAN_POINT ( 'NONE',  ( 135.0000000000015632, 16.00000000000000000, 60.00000000000000000 ) ) ;
#46300=DIRECTION ( 'NONE',  ( -0.000000000000000000, -1.000000000000000000, -0.000000000000000000 ) ) ;
#46304=VERTEX_POINT ( 'NONE', #42059 ) ;
#46311=ORIENTED_EDGE ( 'NONE', *, *, #34964, .T. ) ;
#46319=ORIENTED_EDGE ( 'NONE', *, *, #42198, .F. ) ;
#46320=LINE ( 'NONE', #18880, #25129 ) ;
#46335=EDGE_CURVE ( 'NONE', #14478, #20370, #3056, .T. ) ;
#46341=DIRECTION ( 'NONE',  ( 0.000000000000000000, 0.000000000000000000, -1.000000000000000000 ) ) ;
#46345=ORIENTED_EDGE ( 'NONE', *, *, #7650, .T. ) ;
#46369=AXIS2_PLACEMENT_3D ( 'NONE', #17877, #21233, #36922 ) ;
#46372=LINE ( 'NONE', #3534, #34457 ) ;
#46380=FACE_BOUND ( 'NONE', #29735, .T. ) ;
#46388=PLANE ( 'NONE',  #23254 ) ;
#46397=DIRECTION ( 'NONE',  ( -1.000000000000000000, -0.000000000000000000, -0.000000000000000000 ) ) ;
#46398=ADVANCED_FACE ( 'NONE', ( #47641 ), #4594, .F. ) ;
#46399=VERTEX_POINT ( 'NONE', #43319 ) ;
#46405=CARTESIAN_POINT ( 'NONE',  ( -114.9999999999984652, 16.00000000000000000, 35.00000000000000000 ) ) ;
#46414=ORIENTED_EDGE ( 'NONE', *, *, #32192, .F. ) ;
#46422=VERTEX_POINT ( 'NONE', #32305 ) ;
#46428=ADVANCED_FACE ( 'NONE', ( #43074 ), #16383, .F. ) ;
#46439=ORIENTED_EDGE ( 'NONE', *, *, #35548, .T. ) ;
#46442=CARTESIAN_POINT ( 'NONE',  ( 0.000000000000000000, 17.00000000000000000, 0.000000000000000000 ) ) ;
#46444=PLANE ( 'NONE',  #1204 ) ;
#46446=ORIENTED_EDGE ( 'NONE', *, *, #7650, .F. ) ;
#46452=ORIENTED_EDGE ( 'NONE', *, *, #30355, .T. ) ;
#46457=CARTESIAN_POINT ( 'NONE',  ( -64.99999999999846523, 16.00000000000000000, 60.00000000000000000 ) ) ;
#46467=EDGE_LOOP ( 'NONE', ( #2884, #20331, #15421, #4970 ) ) ;
#46468=DIRECTION ( 'NONE',  ( -0.000000000000000000, -1.000000000000000000, -0.000000000000000000 ) ) ;
#46469=DIRECTION ( 'NONE',  ( -0.000000000000000000, -1.000000000000000000, -0.000000000000000000 ) ) ;
#46471=EDGE_CURVE ( 'NONE', #32541, #20108, #24596, .T. ) ;
#46482=DIRECTION ( 'NONE',  ( -0.000000000000000000, -1.000000000000000000, -0.000000000000000000 ) ) ;
#46483=EDGE_CURVE ( 'NONE', #3284, #25760, #4820, .T. ) ;
#46486=AXIS2_PLACEMENT_3D ( 'NONE', #46752, #10628, #26291 ) ;
#46487=ORIENTED_EDGE ( 'NONE', *, *, #43537, .F. ) ;
#46491=DIRECTION ( 'NONE',  ( -1.000000000000000000, -0.000000000000000000, -0.000000000000000000 ) ) ;
#46503=ORIENTED_EDGE ( 'NONE', *, *, #49346, .F. ) ;
#46504=PLANE ( 'NONE',  #17368 ) ;
#46510=ADVANCED_FACE ( 'NONE', ( #12789 ), #15886, .F. ) ;
#46513=EDGE_CURVE ( 'NONE', #21378, #21529, #32051, .T. ) ;
#46515=PLANE ( 'NONE',  #22093 ) ;
#46524=CARTESIAN_POINT ( 'NONE',  ( 29.99999999999997158, 16.00000000000000000, -114.9999999999999858 ) ) ;
#46526=DIRECTION ( 'NONE',  ( -0.000000000000000000, -0.000000000000000000, -1.000000000000000000 ) ) ;
#46529=EDGE_CURVE ( 'NONE', #21982, #2527, #8707, .T. ) ;
#46550=ADVANCED_FACE ( 'NONE', ( #45317 ), #48396, .F. ) ;
#46565=ORIENTED_EDGE ( 'NONE', *, *, #9010, .T. ) ;
#46571=EDGE_CURVE ( 'NONE', #23363, #30968, #48144, .T. ) ;
#46581=EDGE_LOOP ( 'NONE', ( #43596, #31684, #7593, #15130 ) ) ;
#46590=VERTEX_POINT ( 'NONE', #1751 ) ;
#46596=LINE ( 'NONE', #23025, #26239 ) ;
#46618=PLANE ( 'NONE',  #164 ) ;
#46622=CARTESIAN_POINT ( 'NONE',  ( -165.0000000000000284, 15.00000000000000000, 115.0000000000000142 ) ) ;
#46630=VECTOR ( 'NONE', #35290, 1000.000000000000000 ) ;
#46635=CARTESIAN_POINT ( 'NONE',  ( 30.00000000000062172, 16.00000000000000000, -54.99999999999999289 ) ) ;
#46641=DIRECTION ( 'NONE',  ( 0.000000000000000000, -1.000000000000000000, 0.000000000000000000 ) ) ;
#46646=DIRECTION ( 'NONE',  ( -0.000000000000000000, -1.000000000000000000, -0.000000000000000000 ) ) ;
#46654=VERTEX_POINT ( 'NONE', #49893 ) ;
#46661=ORIENTED_EDGE ( 'NONE', *, *, #12070, .T. ) ;
#46668=VECTOR ( 'NONE', #18916, 1000.000000000000000 ) ;
#46672=ORIENTED_EDGE ( 'NONE', *, *, #38813, .F. ) ;
#46677=VECTOR ( 'NONE', #32286, 1000.000000000000000 ) ;
#46680=VERTEX_POINT ( 'NONE', #45811 ) ;
#46684=CARTESIAN_POINT ( 'NONE',  ( 30.00000000000029132, 17.00000000000000000, -84.99999999999998579 ) ) ;
#46696=VERTEX_POINT ( 'NONE', #10451 ) ;
#46714=CARTESIAN_POINT ( 'NONE',  ( 30.00000000000187228, 17.00000000000000000, 90.00000000000000000 ) ) ;
#46716=LINE ( 'NONE', #23147, #6462 ) ;
#46719=DIRECTION ( 'NONE',  ( -4.625929269271584521E-16, 0.000000000000000000, -1.000000000000000000 ) ) ;
#46720=DIRECTION ( 'NONE',  ( -0.000000000000000000, -1.000000000000000000, -0.000000000000000000 ) ) ;
#46721=CARTESIAN_POINT ( 'NONE',  ( -114.9999999999997158, 17.00000000000000000, -60.00000000000000000 ) ) ;
#46724=ORIENTED_EDGE ( 'NONE', *, *, #21238, .F. ) ;
#46732=ORIENTED_EDGE ( 'NONE', *, *, #16792, .T. ) ;
#46736=CARTESIAN_POINT ( 'NONE',  ( 85.00000000000056843, 17.00000000000000000, -54.99999999999999289 ) ) ;
#46737=VECTOR ( 'NONE', #5351, 1000.000000000000000 ) ;
#46752=CARTESIAN_POINT ( 'NONE',  ( -115.0000000000000284, 17.00000000000000000, -114.9999999999999858 ) ) ;
#46762=VERTEX_POINT ( 'NONE', #14292 ) ;
#46786=DIRECTION ( 'NONE',  ( 0.000000000000000000, 0.000000000000000000, -1.000000000000000000 ) ) ;
#46790=EDGE_CURVE ( 'NONE', #32189, #19150, #21921, .T. ) ;
#46791=EDGE_CURVE ( 'NONE', #41868, #31669, #6511, .T. ) ;
#46808=LINE ( 'NONE', #15553, #27345 ) ;
#46814=PLANE ( 'NONE',  #1457 ) ;
#46826=EDGE_CURVE ( 'NONE', #9263, #12877, #13456, .T. ) ;
#46832=ADVANCED_FACE ( 'NONE', ( #10375 ), #13202, .F. ) ;
#46837=LINE ( 'NONE', #8397, #11452 ) ;
#46844=ORIENTED_EDGE ( 'NONE', *, *, #49025, .T. ) ;
#46846=DIRECTION ( 'NONE',  ( -0.000000000000000000, -1.000000000000000000, -0.000000000000000000 ) ) ;
#46849=AXIS2_PLACEMENT_3D ( 'NONE', #540, #31838, #12824 ) ;
#46853=CARTESIAN_POINT ( 'NONE',  ( -64.99999999999815259, 17.00000000000000000, 65.00000000000000000 ) ) ;
#46856=CARTESIAN_POINT ( 'NONE',  ( -165.0000000000000284, 16.00000000000000000, 95.00000000000000000 ) ) ;
#46865=CARTESIAN_POINT ( 'NONE',  ( -119.9999999999997158, 16.00000000000000000, -84.99999999999998579 ) ) ;
#46867=ADVANCED_FACE ( 'NONE', ( #38319 ), #15206, .F. ) ;
#46868=DIRECTION ( 'NONE',  ( 0.000000000000000000, 0.000000000000000000, 1.000000000000000000 ) ) ;
#46873=FACE_OUTER_BOUND ( 'NONE', #17273, .T. ) ;
#46880=FACE_OUTER_BOUND ( 'NONE', #28538, .T. ) ;
#46887=VECTOR ( 'NONE', #25221, 1000.000000000000000 ) ;
#46888=DIRECTION ( 'NONE',  ( 1.000000000000000000, 0.000000000000000000, 0.000000000000000000 ) ) ;
#46892=LINE ( 'NONE', #4599, #30224 ) ;
#46909=DIRECTION ( 'NONE',  ( -0.000000000000000000, -1.000000000000000000, -0.000000000000000000 ) ) ;
#46916=LINE ( 'NONE', #7976, #44735 ) ;
#46919=EDGE_CURVE ( 'NONE', #24059, #572, #30866, .T. ) ;
#46921=EDGE_CURVE ( 'NONE', #28202, #16567, #42384, .T. ) ;
#46923=VERTEX_POINT ( 'NONE', #37813 ) ;
#46925=EDGE_CURVE ( 'NONE', #9554, #31779, #3129, .T. ) ;
#46930=CARTESIAN_POINT ( 'NONE',  ( -14.99999999999937472, 16.00000000000000000, -54.99999999999999289 ) ) ;
#46932=CARTESIAN_POINT ( 'NONE',  ( 80.00000000000092371, 17.00000000000000000, -24.99999999999999289 ) ) ;
#46934=EDGE_CURVE ( 'NONE', #17054, #34874, #50037, .T. ) ;
#46948=DIRECTION ( 'NONE',  ( -1.000000000000000000, -0.000000000000000000, -0.000000000000000000 ) ) ;
#46955=VECTOR ( 'NONE', #5162, 1000.000000000000000 ) ;
#46971=DIRECTION ( 'NONE',  ( 1.000000000000000000, 0.000000000000000000, 0.000000000000000000 ) ) ;
#46975=DIRECTION ( 'NONE',  ( 0.000000000000000000, -0.000000000000000000, -1.000000000000000000 ) ) ;
#46977=DIRECTION ( 'NONE',  ( 0.000000000000000000, 0.000000000000000000, 1.000000000000000000 ) ) ;
#46987=FACE_OUTER_BOUND ( 'NONE', #41604, .T. ) ;
#46988=VECTOR ( 'NONE', #28453, 1000.000000000000000 ) ;
#47023=ORIENTED_EDGE ( 'NONE', *, *, #37870, .F. ) ;
#47033=DIRECTION ( 'NONE',  ( -1.000000000000000000, -0.000000000000000000, -0.000000000000000000 ) ) ;
#47034=ORIENTED_EDGE ( 'NONE', *, *, #34476, .F. ) ;
#47035=ORIENTED_EDGE ( 'NONE', *, *, #30806, .T. ) ;
#47040=ORIENTED_EDGE ( 'NONE', *, *, #34132, .F. ) ;
#47045=ORIENTED_EDGE ( 'NONE', *, *, #41934, .F. ) ;
#47046=VECTOR ( 'NONE', #11014, 1000.000000000000000 ) ;
#47050=DIRECTION ( 'NONE',  ( 0.000000000000000000, -1.000000000000000000, 0.000000000000000000 ) ) ;
#47054=CARTESIAN_POINT ( 'NONE',  ( 34.99999999999997868, 17.00000000000000000, -90.00000000000000000 ) ) ;
#47059=ADVANCED_FACE ( 'NONE', ( #8525 ), #43396, .F. ) ;
#47062=ORIENTED_EDGE ( 'NONE', *, *, #4222, .F. ) ;
#47065=CARTESIAN_POINT ( 'NONE',  ( 164.9999999999999716, 16.00000000000000000, -60.00000000000000000 ) ) ;
#47081=ADVANCED_FACE ( 'NONE', ( #23412 ), #4903, .F. ) ;
#47082=ORIENTED_EDGE ( 'NONE', *, *, #25874, .F. ) ;
#47085=PLANE ( 'NONE',  #6523 ) ;
#47094=ORIENTED_EDGE ( 'NONE', *, *, #9820, .F. ) ;
#47099=CARTESIAN_POINT ( 'NONE',  ( 29.99999999999998579, 16.00000000000000000, -114.9999999999999858 ) ) ;
#47110=EDGE_CURVE ( 'NONE', #25007, #44339, #16217, .T. ) ;
#47121=CARTESIAN_POINT ( 'NONE',  ( 135.0000000000021600, 17.00000000000000000, 95.00000000000000000 ) ) ;
#47125=DIRECTION ( 'NONE',  ( -1.000000000000000000, 0.000000000000000000, 0.000000000000000000 ) ) ;
#47132=DIRECTION ( 'NONE',  ( 0.000000000000000000, 0.000000000000000000, -1.000000000000000000 ) ) ;
#47137=DIRECTION ( 'NONE',  ( -4.625929269271635797E-16, 0.000000000000000000, -1.000000000000000000 ) ) ;
#47139=DIRECTION ( 'NONE',  ( 0.000000000000000000, -1.000000000000000000, 0.000000000000000000 ) ) ;
#47146=EDGE_CURVE ( 'NONE', #25202, #7505, #33395, .T. ) ;
#47149=ORIENTED_EDGE ( 'NONE', *, *, #30990, .T. ) ;
#47156=VERTEX_POINT ( 'NONE', #41327 ) ;
#47157=ADVANCED_FACE ( 'NONE', ( #17225 ), #17471, .F. ) ;
#47161=ORIENTED_EDGE ( 'NONE', *, *, #17069, .T. ) ;
#47177=EDGE_CURVE ( 'NONE', #19067, #40717, #29524, .T. ) ;
#47191=VERTEX_POINT ( 'NONE', #10027 ) ;
#47192=CARTESIAN_POINT ( 'NONE',  ( 34.99999999999997868, 17.00000000000000000, -90.00000000000000000 ) ) ;
#47193=VECTOR ( 'NONE', #34180, 1000.000000000000000 ) ;
#47197=EDGE_LOOP ( 'NONE', ( #44917, #47231, #18258, #10570 ) ) ;
#47207=ORIENTED_EDGE ( 'NONE', *, *, #45305, .T. ) ;
#47208=CARTESIAN_POINT ( 'NONE',  ( -114.9999999999978542, 16.00000000000000000, 95.00000000000000000 ) ) ;
#47209=FACE_OUTER_BOUND ( 'NONE', #23515, .T. ) ;
#47210=PLANE ( 'NONE',  #33193 ) ;
#47217=ORIENTED_EDGE ( 'NONE', *, *, #23470, .T. ) ;
#47228=DIRECTION ( 'NONE',  ( 1.000000000000000000, -0.000000000000000000, 0.000000000000000000 ) ) ;
#47229=VECTOR ( 'NONE', #35638, 1000.000000000000000 ) ;
#47231=ORIENTED_EDGE ( 'NONE', *, *, #20390, .F. ) ;
#47237=EDGE_LOOP ( 'NONE', ( #47476, #21490, #30601, #5118 ) ) ;
#47241=LINE ( 'NONE', #34741, #45413 ) ;
#47242=CARTESIAN_POINT ( 'NONE',  ( 80.00000000000061107, 16.00000000000000000, -54.99999999999999289 ) ) ;
#47244=VERTEX_POINT ( 'NONE', #46405 ) ;
#47255=FACE_OUTER_BOUND ( 'NONE', #41869, .T. ) ;
#47262=CARTESIAN_POINT ( 'NONE',  ( 85.00000000000152056, 16.00000000000000000, 60.00000000000000000 ) ) ;
#47264=CARTESIAN_POINT ( 'NONE',  ( 0.000000000000000000, 17.00000000000000000, 0.000000000000000000 ) ) ;
#47270=LINE ( 'NONE', #623, #8598 ) ;
#47274=CARTESIAN_POINT ( 'NONE',  ( 80.00000000000186162, 17.00000000000000000, 65.00000000000000000 ) ) ;
#47277=CARTESIAN_POINT ( 'NONE',  ( 175.0000000000000000, 15.00000000000000000, 122.5000000000000142 ) ) ;
#47282=DIRECTION ( 'NONE',  ( 1.000000000000000000, 0.000000000000000000, 0.000000000000000000 ) ) ;
#47283=EDGE_LOOP ( 'NONE', ( #11383, #5011, #7466, #10393 ) ) ;
#47284=DIRECTION ( 'NONE',  ( -0.000000000000000000, -1.000000000000000000, -0.000000000000000000 ) ) ;
#47286=CARTESIAN_POINT ( 'NONE',  ( -164.9999999999987779, 17.00000000000000000, 5.000000000000004441 ) ) ;
#47289=ORIENTED_EDGE ( 'NONE', *, *, #46934, .T. ) ;
#47292=DIRECTION ( 'NONE',  ( 0.000000000000000000, 0.000000000000000000, -1.000000000000000000 ) ) ;
#47294=EDGE_LOOP ( 'NONE', ( #37835, #33377, #24338, #16799 ) ) ;
#47296=DIRECTION ( 'NONE',  ( 1.000000000000000000, 0.000000000000000000, -0.000000000000000000 ) ) ;
#47297=VECTOR ( 'NONE', #27628, 1000.000000000000000 ) ;
#47301=CARTESIAN_POINT ( 'NONE',  ( 135.0000000000006253, 17.00000000000000000, -30.00000000000000000 ) ) ;
#47307=ORIENTED_EDGE ( 'NONE', *, *, #2138, .F. ) ;
#47320=EDGE_CURVE ( 'NONE', #21137, #32019, #26691, .T. ) ;
#47329=CARTESIAN_POINT ( 'NONE',  ( 35.00000000000122213, 16.00000000000000000, 30.00000000000000000 ) ) ;
#47341=FACE_OUTER_BOUND ( 'NONE', #28139, .T. ) ;
#47342=EDGE_CURVE ( 'NONE', #16365, #950, #3323, .T. ) ;
#47373=CARTESIAN_POINT ( 'NONE',  ( 130.0000000000018474, 17.00000000000000000, 65.00000000000000000 ) ) ;
#47378=CARTESIAN_POINT ( 'NONE',  ( 135.0000000000000000, 17.00000000000000000, -114.9999999999999858 ) ) ;
#47381=DIRECTION ( 'NONE',  ( 1.000000000000000000, 0.000000000000000000, -0.000000000000000000 ) ) ;
#47412=AXIS2_PLACEMENT_3D ( 'NONE', #31639, #47228, #27769 ) ;
#47444=DIRECTION ( 'NONE',  ( -0.000000000000000000, -1.000000000000000000, -0.000000000000000000 ) ) ;
#47447=DIRECTION ( 'NONE',  ( 1.000000000000000000, 0.000000000000000000, -4.625929269271635797E-16 ) ) ;
#47449=EDGE_CURVE ( 'NONE', #13767, #50570, #31315, .T. ) ;
#47454=DIRECTION ( 'NONE',  ( 1.000000000000000000, 0.000000000000000000, 0.000000000000000000 ) ) ;
#47458=FACE_OUTER_BOUND ( 'NONE', #21561, .T. ) ;
#47460=CARTESIAN_POINT ( 'NONE',  ( 0.000000000000000000, 17.00000000000000000, 0.000000000000000000 ) ) ;
#47461=EDGE_CURVE ( 'NONE', #14175, #3395, #8462, .T. ) ;
#47473=DIRECTION ( 'NONE',  ( -0.000000000000000000, -1.000000000000000000, -0.000000000000000000 ) ) ;
#47476=ORIENTED_EDGE ( 'NONE', *, *, #33700, .T. ) ;
#47479=VECTOR ( 'NONE', #21184, 1000.000000000000000 ) ;
#47481=LINE ( 'NONE', #12359, #24634 ) ;
#47488=ORIENTED_EDGE ( 'NONE', *, *, #35320, .F. ) ;
#47490=LINE ( 'NONE', #31895, #32512 ) ;
#47495=LINE ( 'NONE', #33412, #13635 ) ;
#47496=DIRECTION ( 'NONE',  ( -0.000000000000000000, -0.000000000000000000, -1.000000000000000000 ) ) ;
#47499=CARTESIAN_POINT ( 'NONE',  ( 0.000000000000000000, 17.00000000000000000, 0.000000000000000000 ) ) ;
#47509=ADVANCED_FACE ( 'NONE', ( #20498 ), #47909, .F. ) ;
#47511=DIRECTION ( 'NONE',  ( -0.000000000000000000, -1.000000000000000000, -0.000000000000000000 ) ) ;
#47512=EDGE_CURVE ( 'NONE', #29738, #37447, #17408, .T. ) ;
#47521=DIRECTION ( 'NONE',  ( 0.000000000000000000, -0.000000000000000000, -1.000000000000000000 ) ) ;
#47547=VECTOR ( 'NONE', #25617, 1000.000000000000000 ) ;
#47549=ORIENTED_EDGE ( 'NONE', *, *, #50536, .F. ) ;
#47580=DIRECTION ( 'NONE',  ( 0.000000000000000000, 0.000000000000000000, 1.000000000000000000 ) ) ;
#47581=DIRECTION ( 'NONE',  ( -0.000000000000000000, -1.000000000000000000, -0.000000000000000000 ) ) ;
#47583=ORIENTED_EDGE ( 'NONE', *, *, #934, .T. ) ;
#47584=DIRECTION ( 'NONE',  ( 0.000000000000000000, 0.000000000000000000, -1.000000000000000000 ) ) ;
#47587=VECTOR ( 'NONE', #42457, 1000.000000000000000 ) ;
#47594=ORIENTED_EDGE ( 'NONE', *, *, #31177, .F. ) ;
#47596=LINE ( 'NONE', #28144, #27892 ) ;
#47605=LINE ( 'NONE', #12486, #17693 ) ;
#47610=PLANE ( 'NONE',  #10982 ) ;
#47611=ORIENTED_EDGE ( 'NONE', *, *, #31783, .T. ) ;
#47612=DIRECTION ( 'NONE',  ( -1.000000000000000000, -0.000000000000000000, -0.000000000000000000 ) ) ;
#47621=VERTEX_POINT ( 'NONE', #7129 ) ;
#47627=ORIENTED_EDGE ( 'NONE', *, *, #8457, .T. ) ;
#47641=FACE_OUTER_BOUND ( 'NONE', #12926, .T. ) ;
#47650=VECTOR ( 'NONE', #39534, 1000.000000000000000 ) ;
#47653=LINE ( 'NONE', #24368, #46737 ) ;
#47663=LINE ( 'NONE', #42833, #9301 ) ;
#47672=ORIENTED_EDGE ( 'NONE', *, *, #28027, .F. ) ;
#47676=EDGE_LOOP ( 'NONE', ( #23421, #11560, #477, #18012 ) ) ;
#47682=CARTESIAN_POINT ( 'NONE',  ( -14.99999999999906919, 17.00000000000000000, 0.000000000000000000 ) ) ;
#47684=DIRECTION ( 'NONE',  ( 0.000000000000000000, 0.000000000000000000, -1.000000000000000000 ) ) ;
#47690=EDGE_CURVE ( 'NONE', #46923, #28634, #38440, .T. ) ;
#47692=ORIENTED_EDGE ( 'NONE', *, *, #13150, .T. ) ;
#47702=ORIENTED_EDGE ( 'NONE', *, *, #19625, .F. ) ;
#47713=ORIENTED_EDGE ( 'NONE', *, *, #47461, .F. ) ;
#47720=LINE ( 'NONE', #29525, #15869 ) ;
#47723=ORIENTED_EDGE ( 'NONE', *, *, #41816, .T. ) ;
#47725=ADVANCED_FACE ( 'NONE', ( #33574 ), #30471, .F. ) ;
#47727=DIRECTION ( 'NONE',  ( -1.000000000000000000, -0.000000000000000000, -0.000000000000000000 ) ) ;
#47728=VECTOR ( 'NONE', #14071, 1000.000000000000000 ) ;
#47729=DIRECTION ( 'NONE',  ( 0.000000000000000000, 0.000000000000000000, 1.000000000000000000 ) ) ;
#47731=PLANE ( 'NONE',  #20560 ) ;
#47732=DIRECTION ( 'NONE',  ( 0.000000000000000000, 0.000000000000000000, 1.000000000000000000 ) ) ;
#47738=LINE ( 'NONE', #48240, #12664 ) ;
#47748=ORIENTED_EDGE ( 'NONE', *, *, #32192, .T. ) ;
#47753=CARTESIAN_POINT ( 'NONE',  ( 85.00000000000090949, 17.00000000000000000, 0.000000000000000000 ) ) ;
#47754=ORIENTED_EDGE ( 'NONE', *, *, #12283, .T. ) ;
#47756=ORIENTED_EDGE ( 'NONE', *, *, #19386, .T. ) ;
#47763=LINE ( 'NONE', #16762, #16212 ) ;
#47767=LINE ( 'NONE', #43953, #14995 ) ;
#47781=LINE ( 'NONE', #14441, #24719 ) ;
#47784=EDGE_CURVE ( 'NONE', #23962, #34772, #690, .T. ) ;
#47813=EDGE_LOOP ( 'NONE', ( #39614, #11627, #42106, #23601 ) ) ;
#47822=CARTESIAN_POINT ( 'NONE',  ( -19.99999999999846523, 16.00000000000000000, 35.00000000000000000 ) ) ;
#47826=AXIS2_PLACEMENT_3D ( 'NONE', #31714, #50375, #23997 ) ;
#47829=VECTOR ( 'NONE', #6179, 1000.000000000000000 ) ;
#47831=DIRECTION ( 'NONE',  ( 1.000000000000000000, 0.000000000000000000, 0.000000000000000000 ) ) ;
#47841=EDGE_LOOP ( 'NONE', ( #43643, #40508, #9440, #32154 ) ) ;
#47851=DIRECTION ( 'NONE',  ( -0.000000000000000000, -1.000000000000000000, -0.000000000000000000 ) ) ;
#47852=EDGE_CURVE ( 'NONE', #36506, #10553, #32753, .T. ) ;
#47854=ORIENTED_EDGE ( 'NONE', *, *, #7055, .F. ) ;
#47867=EDGE_LOOP ( 'NONE', ( #3287, #9537, #20132, #6988 ) ) ;
#47870=PLANE ( 'NONE',  #25846 ) ;
#47881=CARTESIAN_POINT ( 'NONE',  ( -19.99999999999878142, 16.00000000000000000, 5.000000000000004441 ) ) ;
#47890=CARTESIAN_POINT ( 'NONE',  ( 30.00000000000187228, 16.00000000000000000, 65.00000000000000000 ) ) ;
#47893=CARTESIAN_POINT ( 'NONE',  ( 135.0000000000015632, 16.00000000000000000, 35.00000000000000000 ) ) ;
#47895=DIRECTION ( 'NONE',  ( 0.000000000000000000, -0.000000000000000000, -1.000000000000000000 ) ) ;
#47896=ORIENTED_EDGE ( 'NONE', *, *, #27469, .F. ) ;
#47900=AXIS2_PLACEMENT_3D ( 'NONE', #31032, #3819, #43063 ) ;
#47901=DIRECTION ( 'NONE',  ( 1.000000000000000000, 0.000000000000000000, 0.000000000000000000 ) ) ;
#47909=PLANE ( 'NONE',  #7659 ) ;
#47914=ORIENTED_EDGE ( 'NONE', *, *, #47177, .F. ) ;
#47917=VECTOR ( 'NONE', #47982, 1000.000000000000000 ) ;
#47918=ORIENTED_EDGE ( 'NONE', *, *, #13260, .F. ) ;
#47919=DIRECTION ( 'NONE',  ( -0.000000000000000000, -1.000000000000000000, -0.000000000000000000 ) ) ;
#47925=ADVANCED_FACE ( 'NONE', ( #32519 ), #13492, .F. ) ;
#47934=CARTESIAN_POINT ( 'NONE',  ( -19.99999999999785416, 16.00000000000000000, 115.0000000000000142 ) ) ;
#47940=AXIS2_PLACEMENT_3D ( 'NONE', #674, #16326, #36865 ) ;
#47950=ORIENTED_EDGE ( 'NONE', *, *, #28088, .F. ) ;
#47970=VECTOR ( 'NONE', #39113, 1000.000000000000000 ) ;
#47972=CARTESIAN_POINT ( 'NONE',  ( 135.0000000000000000, 17.00000000000000000, -114.9999999999999858 ) ) ;
#47976=ORIENTED_EDGE ( 'NONE', *, *, #28537, .F. ) ;
#47978=ORIENTED_EDGE ( 'NONE', *, *, #1148, .F. ) ;
#47982=DIRECTION ( 'NONE',  ( -1.000000000000000000, -0.000000000000000000, -0.000000000000000000 ) ) ;
#47985=ORIENTED_EDGE ( 'NONE', *, *, #19250, .T. ) ;
#47998=CARTESIAN_POINT ( 'NONE',  ( -69.99999999999972999, 17.00000000000000000, -84.99999999999998579 ) ) ;
#48003=ORIENTED_EDGE ( 'NONE', *, *, #8336, .T. ) ;
#48014=ORIENTED_EDGE ( 'NONE', *, *, #15233, .T. ) ;
#48016=DIRECTION ( 'NONE',  ( 1.000000000000000000, 0.000000000000000000, -0.000000000000000000 ) ) ;
#48029=ORIENTED_EDGE ( 'NONE', *, *, #15059, .F. ) ;
#48040=VERTEX_POINT ( 'NONE', #49605 ) ;
#48052=EDGE_LOOP ( 'NONE', ( #5812, #28292, #20928, #7636 ) ) ;
#48053=ORIENTED_EDGE ( 'NONE', *, *, #21603, .F. ) ;
#48054=ORIENTED_EDGE ( 'NONE', *, *, #27730, .F. ) ;
#48055=LINE ( 'NONE', #8361, #26688 ) ;
#48063=EDGE_CURVE ( 'NONE', #20388, #14316, #29907, .T. ) ;
#48076=EDGE_CURVE ( 'NONE', #42991, #45968, #49845, .T. ) ;
#48083=CARTESIAN_POINT ( 'NONE',  ( -119.9999999999987921, 16.00000000000000000, 30.00000000000000000 ) ) ;
#48088=ADVANCED_FACE ( 'NONE', ( #18096 ), #28531, .F. ) ;
#48093=EDGE_CURVE ( 'NONE', #5809, #11044, #35754, .T. ) ;
#48098=LINE ( 'NONE', #8399, #15183 ) ;
#48107=ORIENTED_EDGE ( 'NONE', *, *, #45303, .F. ) ;
#48108=CARTESIAN_POINT ( 'NONE',  ( -64.99999999999909051, 17.00000000000000000, -24.99999999999999289 ) ) ;
#48111=ORIENTED_EDGE ( 'NONE', *, *, #27288, .F. ) ;
#48118=PLANE ( 'NONE',  #33364 ) ;
#48119=LINE ( 'NONE', #40478, #1601 ) ;
#48125=CARTESIAN_POINT ( 'NONE',  ( 35.00000000000152767, 17.00000000000000000, 60.00000000000000000 ) ) ;
#48131=LINE ( 'NONE', #9178, #37827 ) ;
#48144=LINE ( 'NONE', #37425, #22445 ) ;
#48151=LINE ( 'NONE', #28459, #18857 ) ;
#48181=ORIENTED_EDGE ( 'NONE', *, *, #14357, .F. ) ;
#48192=EDGE_LOOP ( 'NONE', ( #33680, #3943, #25246, #37024 ) ) ;
#48212=CARTESIAN_POINT ( 'NONE',  ( -165.0000000000000284, 16.00000000000000000, -114.9999999999999858 ) ) ;
#48216=VECTOR ( 'NONE', #47444, 1000.000000000000000 ) ;
#48221=ORIENTED_EDGE ( 'NONE', *, *, #726, .T. ) ;
#48240=CARTESIAN_POINT ( 'NONE',  ( -64.99999999999815259, 16.00000000000000000, 65.00000000000000000 ) ) ;
#48245=DIRECTION ( 'NONE',  ( -0.000000000000000000, -1.000000000000000000, -0.000000000000000000 ) ) ;
#48251=FACE_OUTER_BOUND ( 'NONE', #17265, .T. ) ;
#48252=CARTESIAN_POINT ( 'NONE',  ( -164.9999999999994031, 17.00000000000000000, -30.00000000000000000 ) ) ;
#48257=FACE_OUTER_BOUND ( 'NONE', #20391, .T. ) ;
#48275=VECTOR ( 'NONE', #2329, 1000.000000000000000 ) ;
#48279=ORIENTED_EDGE ( 'NONE', *, *, #37199, .T. ) ;
#48281=ORIENTED_EDGE ( 'NONE', *, *, #23675, .F. ) ;
#48284=CARTESIAN_POINT ( 'NONE',  ( -15.00000000000001421, 17.00000000000000000, -114.9999999999999858 ) ) ;
#48289=DIRECTION ( 'NONE',  ( -0.000000000000000000, -1.000000000000000000, -0.000000000000000000 ) ) ;
#48313=VECTOR ( 'NONE', #26351, 1000.000000000000000 ) ;
#48318=VECTOR ( 'NONE', #13589, 1000.000000000000000 ) ;
#48325=VECTOR ( 'NONE', #6625, 1000.000000000000000 ) ;
#48330=ORIENTED_EDGE ( 'NONE', *, *, #34919, .F. ) ;
#48332=FACE_OUTER_BOUND ( 'NONE', #20806, .T. ) ;
#48342=EDGE_CURVE ( 'NONE', #7126, #20602, #2330, .T. ) ;
#48346=DIRECTION ( 'NONE',  ( 0.000000000000000000, -0.000000000000000000, -1.000000000000000000 ) ) ;
#48348=DIRECTION ( 'NONE',  ( -1.000000000000000000, -0.000000000000000000, -0.000000000000000000 ) ) ;
#48353=VECTOR ( 'NONE', #47901, 1000.000000000000000 ) ;
#48359=EDGE_CURVE ( 'NONE', #42474, #23347, #22084, .T. ) ;
#48365=EDGE_CURVE ( 'NONE', #18303, #1528, #23090, .T. ) ;
#48376=LINE ( 'NONE', #12509, #42598 ) ;
#48381=CARTESIAN_POINT ( 'NONE',  ( 164.9999999999999716, 16.00000000000000000, 115.0000000000000142 ) ) ;
#48382=EDGE_CURVE ( 'NONE', #405, #41804, #46146, .T. ) ;
#48385=ADVANCED_FACE ( 'NONE', ( #15145 ), #18720, .F. ) ;
#48390=CARTESIAN_POINT ( 'NONE',  ( -64.99999999999846523, 17.00000000000000000, 35.00000000000000000 ) ) ;
#48396=PLANE ( 'NONE',  #13438 ) ;
#48408=LINE ( 'NONE', #44334, #39921 ) ;
#48414=VECTOR ( 'NONE', #33307, 1000.000000000000000 ) ;
#48424=EDGE_CURVE ( 'NONE', #2839, #2472, #6942, .T. ) ;
#48430=ORIENTED_EDGE ( 'NONE', *, *, #12158, .T. ) ;
#48434=EDGE_LOOP ( 'NONE', ( #39409, #8009, #36601, #908, #36034, #36834, #35073, #14055, #11377, #44529, #3275, #41720, #224, #19044, #37031, #40667, #3614, #11489, #8671, #17373, #44525, #8797, #13874, #25423, #6524, #4931, #20404, #44540, #45208, #45052, #43373, #41765 ) ) ;
#48437=CARTESIAN_POINT ( 'NONE',  ( 30.00000000000062172, 17.00000000000000000, -30.00000000000000000 ) ) ;
#48439=DIRECTION ( 'NONE',  ( -0.000000000000000000, -0.000000000000000000, 1.000000000000000000 ) ) ;
#48440=LINE ( 'NONE', #28988, #7431 ) ;
#48461=LINE ( 'NONE', #18199, #40297 ) ;
#48462=EDGE_CURVE ( 'NONE', #33627, #40517, #39021, .T. ) ;
#48483=AXIS2_PLACEMENT_3D ( 'NONE', #11903, #30909, #38859 ) ;
#48490=EDGE_CURVE ( 'NONE', #14175, #35777, #35688, .T. ) ;
#48491=VERTEX_POINT ( 'NONE', #23349 ) ;
#48516=CARTESIAN_POINT ( 'NONE',  ( -69.99999999999940314, 17.00000000000000000, -54.99999999999999289 ) ) ;
#48519=CARTESIAN_POINT ( 'NONE',  ( 35.00000000000091660, 17.00000000000000000, 0.000000000000000000 ) ) ;
#48525=PLANE ( 'NONE',  #45756 ) ;
#48527=EDGE_CURVE ( 'NONE', #41913, #9256, #47663, .T. ) ;
#48532=CARTESIAN_POINT ( 'NONE',  ( -164.9999999999987779, 17.00000000000000000, 30.00000000000000000 ) ) ;
#48537=ORIENTED_EDGE ( 'NONE', *, *, #30976, .T. ) ;
#48538=ORIENTED_EDGE ( 'NONE', *, *, #32289, .F. ) ;
#48542=CARTESIAN_POINT ( 'NONE',  ( 35.00000000000091660, 17.00000000000000000, 0.000000000000000000 ) ) ;
#48545=CARTESIAN_POINT ( 'NONE',  ( -19.99999999999908695, 16.00000000000000000, -24.99999999999999289 ) ) ;
#48546=VERTEX_POINT ( 'NONE', #16168 ) ;
#48549=CARTESIAN_POINT ( 'NONE',  ( -19.99999999999878142, 16.00000000000000000, 30.00000000000000000 ) ) ;
#48560=EDGE_LOOP ( 'NONE', ( #45778, #49480, #24113, #6481 ) ) ;
#48563=VERTEX_POINT ( 'NONE', #15653 ) ;
#48564=VECTOR ( 'NONE', #41249, 1000.000000000000000 ) ;
#48570=DIRECTION ( 'NONE',  ( -0.000000000000000000, -0.000000000000000000, -1.000000000000000000 ) ) ;
#48582=DIRECTION ( 'NONE',  ( 0.000000000000000000, 0.000000000000000000, 1.000000000000000000 ) ) ;
#48590=VECTOR ( 'NONE', #13947, 1000.000000000000000 ) ;
#48608=CARTESIAN_POINT ( 'NONE',  ( -64.99999999999909051, 17.00000000000000000, 0.000000000000000000 ) ) ;
#48610=CARTESIAN_POINT ( 'NONE',  ( 135.0000000000019043, 17.00000000000000000, 65.00000000000000000 ) ) ;
#48623=VECTOR ( 'NONE', #34534, 1000.000000000000000 ) ;
#48633=LINE ( 'NONE', #33306, #7196 ) ;
#48636=PLANE ( 'NONE',  #46369 ) ;
#48642=AXIS2_PLACEMENT_3D ( 'NONE', #41110, #21606, #38486 ) ;
#48643=CARTESIAN_POINT ( 'NONE',  ( -20.00000000000003197, 17.00000000000000000, -114.9999999999999858 ) ) ;
#48655=AXIS2_PLACEMENT_3D ( 'NONE', #10111, #28860, #25769 ) ;
#48657=CARTESIAN_POINT ( 'NONE',  ( 35.00000000000216716, 17.00000000000000000, 115.0000000000000142 ) ) ;
#48662=VECTOR ( 'NONE', #30830, 1000.000000000000000 ) ;
#48664=EDGE_CURVE ( 'NONE', #7126, #42669, #24868, .T. ) ;
#48668=LINE ( 'NONE', #42026, #29005 ) ;
#48684=EDGE_LOOP ( 'NONE', ( #48330, #2335, #11960, #49982 ) ) ;
#48688=ORIENTED_EDGE ( 'NONE', *, *, #4044, .F. ) ;
#48694=PLANE ( 'NONE',  #35499 ) ;
#48699=VECTOR ( 'NONE', #4069, 1000.000000000000000 ) ;
#48700=VERTEX_POINT ( 'NONE', #17905 ) ;
#48707=ORIENTED_EDGE ( 'NONE', *, *, #24245, .F. ) ;
#48708=EDGE_CURVE ( 'NONE', #41095, #10553, #48668, .T. ) ;
#48709=FACE_OUTER_BOUND ( 'NONE', #4356, .T. ) ;
#48711=EDGE_CURVE ( 'NONE', #2212, #39326, #38453, .T. ) ;
#48720=VECTOR ( 'NONE', #46397, 1000.000000000000000 ) ;
#48731=ORIENTED_EDGE ( 'NONE', *, *, #8476, .F. ) ;
#48735=VECTOR ( 'NONE', #17923, 1000.000000000000000 ) ;
#48739=ORIENTED_EDGE ( 'NONE', *, *, #10848, .T. ) ;
#48761=VECTOR ( 'NONE', #21156, 1000.000000000000000 ) ;
#48764=CARTESIAN_POINT ( 'NONE',  ( -164.9999999999981526, 17.00000000000000000, 65.00000000000000000 ) ) ;
#48765=VECTOR ( 'NONE', #48946, 1000.000000000000000 ) ;
#48775=CARTESIAN_POINT ( 'NONE',  ( -114.9999999999981526, 17.00000000000000000, 90.00000000000000000 ) ) ;
#48786=LINE ( 'NONE', #37312, #25890 ) ;
#48793=LINE ( 'NONE', #32953, #19641 ) ;
#48798=DIRECTION ( 'NONE',  ( -0.000000000000000000, -1.000000000000000000, -0.000000000000000000 ) ) ;
#48799=LINE ( 'NONE', #49038, #45899 ) ;
#48829=CARTESIAN_POINT ( 'NONE',  ( -114.9999999999994031, 17.00000000000000000, -54.99999999999999289 ) ) ;
#48830=EDGE_CURVE ( 'NONE', #34173, #20578, #4047, .T. ) ;
#48834=VECTOR ( 'NONE', #27101, 1000.000000000000000 ) ;
#48842=EDGE_CURVE ( 'NONE', #18457, #32184, #16103, .T. ) ;
#48850=ORIENTED_EDGE ( 'NONE', *, *, #22162, .T. ) ;
#48858=EDGE_LOOP ( 'NONE', ( #35380, #21021, #43390, #8746 ) ) ;
#48869=DIRECTION ( 'NONE',  ( -0.000000000000000000, -0.000000000000000000, -1.000000000000000000 ) ) ;
#48893=AXIS2_PLACEMENT_3D ( 'NONE', #7936, #19719, #988 ) ;
#48896=EDGE_CURVE ( 'NONE', #3284, #37192, #3791, .T. ) ;
#48904=CARTESIAN_POINT ( 'NONE',  ( 135.0000000000012790, 16.00000000000000000, 5.000000000000004441 ) ) ;
#48905=ORIENTED_EDGE ( 'NONE', *, *, #12633, .F. ) ;
#48920=CARTESIAN_POINT ( 'NONE',  ( -165.0000000000000284, 16.00000000000000000, 115.0000000000000142 ) ) ;
#48922=CARTESIAN_POINT ( 'NONE',  ( -165.0000000000000284, 15.00000000000000000, -114.9999999999999858 ) ) ;
#48928=VECTOR ( 'NONE', #21169, 1000.000000000000000 ) ;
#48929=FACE_OUTER_BOUND ( 'NONE', #8213, .T. ) ;
#48933=ORIENTED_EDGE ( 'NONE', *, *, #17091, .T. ) ;
#48940=ORIENTED_EDGE ( 'NONE', *, *, #39187, .T. ) ;
#48945=CARTESIAN_POINT ( 'NONE',  ( 80.00000000000061107, 17.00000000000000000, -54.99999999999999289 ) ) ;
#48946=DIRECTION ( 'NONE',  ( -0.000000000000000000, -1.000000000000000000, -0.000000000000000000 ) ) ;
#48955=ADVANCED_FACE ( 'NONE', ( #20202 ), #47610, .F. ) ;
#48992=CARTESIAN_POINT ( 'NONE',  ( 130.0000000000012221, 16.00000000000000000, 5.000000000000004441 ) ) ;
#48999=AXIS2_PLACEMENT_3D ( 'NONE', #21680, #41437, #22437 ) ;
#49004=CARTESIAN_POINT ( 'NONE',  ( -120.0000000000000426, 17.00000000000000000, -114.9999999999999858 ) ) ;
#49009=CARTESIAN_POINT ( 'NONE',  ( 34.99999999999997868, 17.00000000000000000, -114.9999999999999858 ) ) ;
#49018=DIRECTION ( 'NONE',  ( -0.000000000000000000, -1.000000000000000000, -0.000000000000000000 ) ) ;
#49021=EDGE_CURVE ( 'NONE', #44903, #13654, #33285, .T. ) ;
#49025=EDGE_CURVE ( 'NONE', #6936, #27632, #33026, .T. ) ;
#49038=CARTESIAN_POINT ( 'NONE',  ( -114.9999999999997158, 17.00000000000000000, -60.00000000000000000 ) ) ;
#49041=VECTOR ( 'NONE', #34195, 1000.000000000000000 ) ;
#49046=ORIENTED_EDGE ( 'NONE', *, *, #35549, .T. ) ;
#49051=ADVANCED_FACE ( 'NONE', ( #2462 ), #49615, .F. ) ;
#49052=EDGE_CURVE ( 'NONE', #46304, #6217, #10417, .T. ) ;
#49053=ORIENTED_EDGE ( 'NONE', *, *, #27810, .T. ) ;
#49056=CARTESIAN_POINT ( 'NONE',  ( -64.99999999999783995, 17.00000000000000000, 95.00000000000000000 ) ) ;
#49058=LINE ( 'NONE', #25012, #8388 ) ;
#49060=EDGE_CURVE ( 'NONE', #14979, #30626, #26830, .T. ) ;
#49068=ORIENTED_EDGE ( 'NONE', *, *, #1734, .T. ) ;
#49071=VERTEX_POINT ( 'NONE', #37637 ) ;
#49085=CARTESIAN_POINT ( 'NONE',  ( 85.00000000000090949, 16.00000000000000000, 0.000000000000000000 ) ) ;
#49091=DIRECTION ( 'NONE',  ( 1.000000000000000000, 0.000000000000000000, -0.000000000000000000 ) ) ;
#49097=LINE ( 'NONE', #36874, #47479 ) ;
#49100=DIRECTION ( 'NONE',  ( -9.251858538542979716E-16, 0.000000000000000000, -1.000000000000000000 ) ) ;
#49120=AXIS2_PLACEMENT_3D ( 'NONE', #43364, #12573, #28243 ) ;
#49133=ORIENTED_EDGE ( 'NONE', *, *, #30838, .F. ) ;
#49134=FACE_OUTER_BOUND ( 'NONE', #21312, .T. ) ;
#49137=CARTESIAN_POINT ( 'NONE',  ( -64.99999999999940314, 16.00000000000000000, -30.00000000000000000 ) ) ;
#49139=DIRECTION ( 'NONE',  ( 0.000000000000000000, -1.000000000000000000, 0.000000000000000000 ) ) ;
#49140=CARTESIAN_POINT ( 'NONE',  ( -14.99999999999970868, 17.00000000000000000, -84.99999999999998579 ) ) ;
#49143=LINE ( 'NONE', #37417, #1174 ) ;
#49153=VECTOR ( 'NONE', #46044, 1000.000000000000000 ) ;
#49155=LINE ( 'NONE', #29703, #38971 ) ;
#49161=DIRECTION ( 'NONE',  ( 0.000000000000000000, 0.000000000000000000, 1.000000000000000000 ) ) ;
#49162=ORIENTED_EDGE ( 'NONE', *, *, #25525, .F. ) ;
#49163=LINE ( 'NONE', #14556, #7502 ) ;
#49164=DIRECTION ( 'NONE',  ( 0.000000000000000000, 0.000000000000000000, -1.000000000000000000 ) ) ;
#49173=ORIENTED_EDGE ( 'NONE', *, *, #17972, .F. ) ;
#49177=FACE_OUTER_BOUND ( 'NONE', #455, .T. ) ;
#49179=PLANE ( 'NONE',  #3847 ) ;
#49188=CARTESIAN_POINT ( 'NONE',  ( -114.9999999999994031, 17.00000000000000000, -30.00000000000000000 ) ) ;
#49189=DIRECTION ( 'NONE',  ( -1.000000000000000000, -0.000000000000000000, -0.000000000000000000 ) ) ;
#49191=ORIENTED_EDGE ( 'NONE', *, *, #48896, .T. ) ;
#49192=ORIENTED_EDGE ( 'NONE', *, *, #44584, .F. ) ;
#49196=CARTESIAN_POINT ( 'NONE',  ( 164.9999999999999716, 16.00000000000000000, 0.000000000000000000 ) ) ;
#49197=VECTOR ( 'NONE', #36104, 1000.000000000000000 ) ;
#49201=FACE_BOUND ( 'NONE', #32950, .T. ) ;
#49213=LINE ( 'NONE', #45126, #19925 ) ;
#49214=ORIENTED_EDGE ( 'NONE', *, *, #34452, .F. ) ;
#49220=ADVANCED_FACE ( 'NONE', ( #31448 ), #19880, .F. ) ;
#49226=DIRECTION ( 'NONE',  ( -0.000000000000000000, -1.000000000000000000, -0.000000000000000000 ) ) ;
#49228=CARTESIAN_POINT ( 'NONE',  ( 35.00000000000061107, 16.00000000000000000, -30.00000000000000000 ) ) ;
#49232=DIRECTION ( 'NONE',  ( 0.000000000000000000, 0.000000000000000000, -1.000000000000000000 ) ) ;
#49234=DIRECTION ( 'NONE',  ( -0.000000000000000000, -1.000000000000000000, -0.000000000000000000 ) ) ;
#49240=ORIENTED_EDGE ( 'NONE', *, *, #28567, .F. ) ;
#49244=CARTESIAN_POINT ( 'NONE',  ( 164.9999999999999716, 16.00000000000000000, 115.0000000000000142 ) ) ;
#49246=CARTESIAN_POINT ( 'NONE',  ( 135.0000000000019043, 16.00000000000000000, 90.00000000000000000 ) ) ;
#49258=AXIS2_PLACEMENT_3D ( 'NONE', #24166, #39822, #4660 ) ;
#49260=CARTESIAN_POINT ( 'NONE',  ( 85.00000000000123634, 16.00000000000000000, 5.000000000000004441 ) ) ;
#49261=CARTESIAN_POINT ( 'NONE',  ( -20.00000000000003197, 17.00000000000000000, -114.9999999999999858 ) ) ;
#49277=PLANE ( 'NONE',  #44092 ) ;
#49282=DIRECTION ( 'NONE',  ( -0.000000000000000000, -1.000000000000000000, -0.000000000000000000 ) ) ;
#49292=DIRECTION ( 'NONE',  ( -0.000000000000000000, -1.000000000000000000, -0.000000000000000000 ) ) ;
#49306=DIRECTION ( 'NONE',  ( -0.000000000000000000, -0.000000000000000000, -1.000000000000000000 ) ) ;
#49307=LINE ( 'NONE', #44729, #35468 ) ;
#49313=EDGE_CURVE ( 'NONE', #19392, #49920, #20385, .T. ) ;
#49314=CARTESIAN_POINT ( 'NONE',  ( 80.00000000000186162, 16.00000000000000000, 65.00000000000000000 ) ) ;
#49319=PLANE ( 'NONE',  #28414 ) ;
#49330=FACE_OUTER_BOUND ( 'NONE', #1976, .T. ) ;
#49346=EDGE_CURVE ( 'NONE', #29552, #39659, #21147, .T. ) ;
#49351=EDGE_CURVE ( 'NONE', #22127, #5410, #44727, .T. ) ;
#49355=LINE ( 'NONE', #33510, #13946 ) ;
#49370=DIRECTION ( 'NONE',  ( 1.000000000000000000, 0.000000000000000000, 0.000000000000000000 ) ) ;
#49386=CARTESIAN_POINT ( 'NONE',  ( 30.00000000000123279, 17.00000000000000000, 5.000000000000004441 ) ) ;
#49387=LINE ( 'NONE', #49137, #16850 ) ;
#49405=EDGE_CURVE ( 'NONE', #1663, #35301, #33966, .T. ) ;
#49416=CARTESIAN_POINT ( 'NONE',  ( -14.99999999999876366, 16.00000000000000000, 5.000000000000004441 ) ) ;
#49419=CARTESIAN_POINT ( 'NONE',  ( -14.99999999999876366, 17.00000000000000000, 30.00000000000000000 ) ) ;
#49420=DIRECTION ( 'NONE',  ( 1.000000000000000000, 0.000000000000000000, -0.000000000000000000 ) ) ;
#49422=EDGE_CURVE ( 'NONE', #37462, #4392, #14188, .T. ) ;
#49439=VECTOR ( 'NONE', #18193, 1000.000000000000000 ) ;
#49443=DIRECTION ( 'NONE',  ( -0.000000000000000000, -0.000000000000000000, -1.000000000000000000 ) ) ;
#49451=EDGE_CURVE ( 'NONE', #375, #39210, #41147, .T. ) ;
#49453=FACE_BOUND ( 'NONE', #26689, .T. ) ;
#49462=CARTESIAN_POINT ( 'NONE',  ( -165.0000000000000284, 17.00000000000000000, 115.0000000000000142 ) ) ;
#49463=LINE ( 'NONE', #23580, #47046 ) ;
#49467=CARTESIAN_POINT ( 'NONE',  ( 80.00000000000217426, 16.00000000000000000, 115.0000000000000142 ) ) ;
#49477=ADVANCED_FACE ( 'NONE', ( #49556 ), #26512, .F. ) ;
#49480=ORIENTED_EDGE ( 'NONE', *, *, #10202, .F. ) ;
#49483=EDGE_CURVE ( 'NONE', #29419, #5984, #41909, .T. ) ;
#49484=CARTESIAN_POINT ( 'NONE',  ( -14.99999999999970868, 17.00000000000000000, -60.00000000000000000 ) ) ;
#49487=DIRECTION ( 'NONE',  ( -1.000000000000000000, 0.000000000000000000, 0.000000000000000000 ) ) ;
#49491=ORIENTED_EDGE ( 'NONE', *, *, #14042, .F. ) ;
#49492=CARTESIAN_POINT ( 'NONE',  ( -165.0000000000000284, 16.00000000000000000, 115.0000000000000142 ) ) ;
#49496=DIRECTION ( 'NONE',  ( -1.000000000000000000, -0.000000000000000000, -0.000000000000000000 ) ) ;
#49504=CARTESIAN_POINT ( 'NONE',  ( -14.99999999999812594, 16.00000000000000000, 90.00000000000000000 ) ) ;
#49522=VECTOR ( 'NONE', #25059, 1000.000000000000000 ) ;
#49526=PLANE ( 'NONE',  #24813 ) ;
#49542=VECTOR ( 'NONE', #47132, 1000.000000000000000 ) ;
#49551=CARTESIAN_POINT ( 'NONE',  ( 84.99999999999997158, 17.00000000000000000, -90.00000000000000000 ) ) ;
#49553=VECTOR ( 'NONE', #24941, 1000.000000000000000 ) ;
#49556=FACE_OUTER_BOUND ( 'NONE', #26560, .T. ) ;
#49558=LINE ( 'NONE', #45724, #43604 ) ;
#49571=EDGE_LOOP ( 'NONE', ( #17742, #17184, #1375, #35364 ) ) ;
#49575=VECTOR ( 'NONE', #37920, 1000.000000000000000 ) ;
#49582=CARTESIAN_POINT ( 'NONE',  ( -19.99999999999815969, 16.00000000000000000, 65.00000000000000000 ) ) ;
#49588=FACE_OUTER_BOUND ( 'NONE', #2735, .T. ) ;
#49590=VECTOR ( 'NONE', #1282, 1000.000000000000000 ) ;
#49599=EDGE_CURVE ( 'NONE', #26763, #8001, #47241, .T. ) ;
#49600=ORIENTED_EDGE ( 'NONE', *, *, #12631, .T. ) ;
#49602=VECTOR ( 'NONE', #32025, 1000.000000000000000 ) ;
#49605=CARTESIAN_POINT ( 'NONE',  ( 130.0000000000021032, 17.00000000000000000, 115.0000000000000142 ) ) ;
#49609=ORIENTED_EDGE ( 'NONE', *, *, #7311, .F. ) ;
#49613=ORIENTED_EDGE ( 'NONE', *, *, #44298, .T. ) ;
#49615=PLANE ( 'NONE',  #19993 ) ;
#49619=ORIENTED_EDGE ( 'NONE', *, *, #43586, .F. ) ;
#49621=EDGE_CURVE ( 'NONE', #572, #34164, #8040, .T. ) ;
#49635=DIRECTION ( 'NONE',  ( 0.000000000000000000, -1.000000000000000000, 0.000000000000000000 ) ) ;
#49655=ADVANCED_FACE ( 'NONE', ( #40345 ), #36512, .F. ) ;
#49666=VECTOR ( 'NONE', #13068, 1000.000000000000000 ) ;
#49669=DIRECTION ( 'NONE',  ( 9.251858538543084240E-16, -0.000000000000000000, 1.000000000000000000 ) ) ;
#49671=DIRECTION ( 'NONE',  ( -0.000000000000000000, -1.000000000000000000, -0.000000000000000000 ) ) ;
#49676=EDGE_CURVE ( 'NONE', #2527, #41220, #4928, .T. ) ;
#49678=ORIENTED_EDGE ( 'NONE', *, *, #2908, .F. ) ;
#49683=DIRECTION ( 'NONE',  ( 0.000000000000000000, 0.000000000000000000, 1.000000000000000000 ) ) ;
#49689=CARTESIAN_POINT ( 'NONE',  ( -164.9999999999978400, 17.00000000000000000, 95.00000000000000000 ) ) ;
#49692=EDGE_CURVE ( 'NONE', #46590, #574, #598, .T. ) ;
#49695=ORIENTED_EDGE ( 'NONE', *, *, #22745, .T. ) ;
#49696=ORIENTED_EDGE ( 'NONE', *, *, #46790, .F. ) ;
#49716=CARTESIAN_POINT ( 'NONE',  ( -64.99999999999877787, 16.00000000000000000, 5.000000000000004441 ) ) ;
#49722=FACE_OUTER_BOUND ( 'NONE', #30733, .T. ) ;
#49735=VECTOR ( 'NONE', #33494, 1000.000000000000000 ) ;
#49738=DIRECTION ( 'NONE',  ( 0.000000000000000000, 0.000000000000000000, 1.000000000000000000 ) ) ;
#49743=VERTEX_POINT ( 'NONE', #6132 ) ;
#49745=EDGE_CURVE ( 'NONE', #44556, #22127, #47738, .T. ) ;
#49758=CARTESIAN_POINT ( 'NONE',  ( -64.99999999999971578, 17.00000000000000000, -84.99999999999998579 ) ) ;
#49759=EDGE_CURVE ( 'NONE', #32394, #32969, #20831, .T. ) ;
#49766=VERTEX_POINT ( 'NONE', #37700 ) ;
#49770=PLANE ( 'NONE',  #10282 ) ;
#49774=LINE ( 'NONE', #14674, #2677 ) ;
#49784=LINE ( 'NONE', #25744, #44268 ) ;
#49790=CARTESIAN_POINT ( 'NONE',  ( 85.00000000000152056, 17.00000000000000000, 60.00000000000000000 ) ) ;
#49796=EDGE_LOOP ( 'NONE', ( #45238, #38635, #28489, #3149 ) ) ;
#49800=VECTOR ( 'NONE', #40633, 1000.000000000000000 ) ;
#49803=CARTESIAN_POINT ( 'NONE',  ( 80.00000000000122213, 17.00000000000000000, 30.00000000000000000 ) ) ;
#49804=PLANE ( 'NONE',  #23471 ) ;
#49813=VERTEX_POINT ( 'NONE', #11500 ) ;
#49815=ORIENTED_EDGE ( 'NONE', *, *, #43066, .T. ) ;
#49834=DIRECTION ( 'NONE',  ( -0.000000000000000000, -0.000000000000000000, -1.000000000000000000 ) ) ;
#49845=LINE ( 'NONE', #2452, #40443 ) ;
#49848=PRODUCT ( 'solar panel', 'solar panel', '', ( #32100 ) ) ;
#49850=DIRECTION ( 'NONE',  ( 1.000000000000000000, 0.000000000000000000, 0.000000000000000000 ) ) ;
#49855=DIRECTION ( 'NONE',  ( 1.000000000000000000, 0.000000000000000000, 0.000000000000000000 ) ) ;
#49859=CARTESIAN_POINT ( 'NONE',  ( 80.00000000000186162, 16.00000000000000000, 90.00000000000000000 ) ) ;
#49889=EDGE_CURVE ( 'NONE', #13738, #30975, #33851, .T. ) ;
#49893=CARTESIAN_POINT ( 'NONE',  ( 35.00000000000216716, 16.00000000000000000, 95.00000000000000000 ) ) ;
#49894=ORIENTED_EDGE ( 'NONE', *, *, #20811, .F. ) ;
#49899=VECTOR ( 'NONE', #49234, 1000.000000000000000 ) ;
#49903=ORIENTED_EDGE ( 'NONE', *, *, #35057, .T. ) ;
#49910=CARTESIAN_POINT ( 'NONE',  ( 130.0000000000015064, 16.00000000000000000, 35.00000000000000000 ) ) ;
#49919=CARTESIAN_POINT ( 'NONE',  ( -114.9999999999981526, 16.00000000000000000, 65.00000000000000000 ) ) ;
#49920=VERTEX_POINT ( 'NONE', #15094 ) ;
#49926=EDGE_CURVE ( 'NONE', #18303, #32019, #30752, .T. ) ;
#49927=ORIENTED_EDGE ( 'NONE', *, *, #49021, .T. ) ;
#49928=CARTESIAN_POINT ( 'NONE',  ( -164.9999999999984936, 17.00000000000000000, 35.00000000000000000 ) ) ;
#49931=CARTESIAN_POINT ( 'NONE',  ( -165.0000000000000284, 16.00000000000000000, -114.9999999999999858 ) ) ;
#49934=ORIENTED_EDGE ( 'NONE', *, *, #43537, .T. ) ;
#49937=DIRECTION ( 'NONE',  ( 0.000000000000000000, 0.000000000000000000, 1.000000000000000000 ) ) ;
#49948=VECTOR ( 'NONE', #50362, 1000.000000000000000 ) ;
#49950=DIRECTION ( 'NONE',  ( 1.000000000000000000, 0.000000000000000000, 0.000000000000000000 ) ) ;
#49951=FACE_BOUND ( 'NONE', #1292, .T. ) ;
#49953=FACE_OUTER_BOUND ( 'NONE', #26869, .T. ) ;
#49955=LINE ( 'NONE', #19460, #3693 ) ;
#49968=DIRECTION ( 'NONE',  ( -0.000000000000000000, -1.000000000000000000, -0.000000000000000000 ) ) ;
#49970=EDGE_CURVE ( 'NONE', #23499, #35246, #7652, .T. ) ;
#49982=ORIENTED_EDGE ( 'NONE', *, *, #43065, .F. ) ;
#49986=AXIS2_PLACEMENT_3D ( 'NONE', #39713, #40463, #13241 ) ;
#49992=CARTESIAN_POINT ( 'NONE',  ( -164.9999999999978400, 17.00000000000000000, 95.00000000000000000 ) ) ;
#49995=ORIENTED_EDGE ( 'NONE', *, *, #48711, .F. ) ;
#49996=VECTOR ( 'NONE', #33632, 1000.000000000000000 ) ;
#49997=ORIENTED_EDGE ( 'NONE', *, *, #9629, .T. ) ;
#50001=CARTESIAN_POINT ( 'NONE',  ( 35.00000000000216716, 16.00000000000000000, 95.00000000000000000 ) ) ;
#50005=CARTESIAN_POINT ( 'NONE',  ( 130.0000000000005684, 17.00000000000000000, -54.99999999999999289 ) ) ;
#50011=ORIENTED_EDGE ( 'NONE', *, *, #16121, .F. ) ;
#50022=CARTESIAN_POINT ( 'NONE',  ( 0.000000000000000000, 17.00000000000000000, 0.000000000000000000 ) ) ;
#50023=FACE_OUTER_BOUND ( 'NONE', #31901, .T. ) ;
#50025=CARTESIAN_POINT ( 'NONE',  ( -115.0000000000000284, 17.00000000000000000, -90.00000000000000000 ) ) ;
#50026=VECTOR ( 'NONE', #15728, 1000.000000000000000 ) ;
#50027=CARTESIAN_POINT ( 'NONE',  ( -119.9999999999978400, 17.00000000000000000, 115.0000000000000142 ) ) ;
#50037=LINE ( 'NONE', #41638, #26555 ) ;
#50039=DIRECTION ( 'NONE',  ( 1.000000000000000000, 0.000000000000000000, 0.000000000000000000 ) ) ;
#50047=CARTESIAN_POINT ( 'NONE',  ( -65.00000000000002842, 17.00000000000000000, -90.00000000000000000 ) ) ;
#50048=DIRECTION ( 'NONE',  ( 1.000000000000000000, 0.000000000000000000, 0.000000000000000000 ) ) ;
#50050=EDGE_CURVE ( 'NONE', #32019, #28645, #37399, .T. ) ;
#50062=ORIENTED_EDGE ( 'NONE', *, *, #18779, .T. ) ;
#50063=CARTESIAN_POINT ( 'NONE',  ( 164.9999999999999716, 16.00000000000000000, -30.00000000000000000 ) ) ;
#50069=EDGE_LOOP ( 'NONE', ( #15349, #36161, #9116, #22792 ) ) ;
#50078=FACE_OUTER_BOUND ( 'NONE', #8736, .T. ) ;
#50080=FACE_OUTER_BOUND ( 'NONE', #31611, .T. ) ;
#50089=CARTESIAN_POINT ( 'NONE',  ( 35.00000000000061107, 17.00000000000000000, -30.00000000000000000 ) ) ;
#50094=AXIS2_PLACEMENT_3D ( 'NONE', #41435, #25533, #46004 ) ;
#50109=ORIENTED_EDGE ( 'NONE', *, *, #32807, .T. ) ;
#50118=VERTEX_POINT ( 'NONE', #40971 ) ;
#50142=CARTESIAN_POINT ( 'NONE',  ( 34.99999999999997868, 17.00000000000000000, -114.9999999999999858 ) ) ;
#50144=CARTESIAN_POINT ( 'NONE',  ( 0.000000000000000000, 17.00000000000000000, 0.000000000000000000 ) ) ;
#50148=FACE_OUTER_BOUND ( 'NONE', #47813, .T. ) ;
#50152=DIRECTION ( 'NONE',  ( 0.000000000000000000, 0.000000000000000000, 1.000000000000000000 ) ) ;
#50162=EDGE_CURVE ( 'NONE', #15972, #30725, #5815, .T. ) ;
#50171=EDGE_LOOP ( 'NONE', ( #23157, #48905, #22466, #22050 ) ) ;
#50183=DIRECTION ( 'NONE',  ( 0.000000000000000000, -0.000000000000000000, -1.000000000000000000 ) ) ;
#50192=VERTEX_POINT ( 'NONE', #49859 ) ;
#50195=CARTESIAN_POINT ( 'NONE',  ( -69.99999999999972999, 17.00000000000000000, -84.99999999999998579 ) ) ;
#50196=FACE_BOUND ( 'NONE', #8460, .T. ) ;
#50200=DIRECTION ( 'NONE',  ( 0.000000000000000000, 0.000000000000000000, 1.000000000000000000 ) ) ;
#50202=CARTESIAN_POINT ( 'NONE',  ( 164.9999999999999716, 17.00000000000000000, -55.00000000000000711 ) ) ;
#50203=CARTESIAN_POINT ( 'NONE',  ( 135.0000000000021600, 17.00000000000000000, 95.00000000000000000 ) ) ;
#50218=DIRECTION ( 'NONE',  ( -0.000000000000000000, -1.000000000000000000, -0.000000000000000000 ) ) ;
#50220=EDGE_CURVE ( 'NONE', #31254, #22853, #7085, .T. ) ;
#50221=LINE ( 'NONE', #11796, #17190 ) ;
#50236=VERTEX_POINT ( 'NONE', #34540 ) ;
#50241=CARTESIAN_POINT ( 'NONE',  ( -15.00000000000001421, 17.00000000000000000, -114.9999999999999858 ) ) ;
#50244=ORIENTED_EDGE ( 'NONE', *, *, #22195, .F. ) ;
#50246=PLANE ( 'NONE',  #31676 ) ;
#50254=CARTESIAN_POINT ( 'NONE',  ( -114.9999999999984652, 17.00000000000000000, 60.00000000000000000 ) ) ;
#50267=LINE ( 'NONE', #6710, #24260 ) ;
#50277=LINE ( 'NONE', #11847, #21743 ) ;
#50278=DIRECTION ( 'NONE',  ( -1.000000000000000000, -0.000000000000000000, 4.625929269271584521E-16 ) ) ;
#50280=ORIENTED_EDGE ( 'NONE', *, *, #33997, .F. ) ;
#50281=CARTESIAN_POINT ( 'NONE',  ( -114.9999999999991047, 17.00000000000000000, -24.99999999999999289 ) ) ;
#50290=EDGE_CURVE ( 'NONE', #21162, #38025, #33207, .T. ) ;
#50294=DIRECTION ( 'NONE',  ( -0.000000000000000000, -1.000000000000000000, -0.000000000000000000 ) ) ;
#50303=FACE_OUTER_BOUND ( 'NONE', #6708, .T. ) ;
#50310=ORIENTED_EDGE ( 'NONE', *, *, #24754, .T. ) ;
#50317=LINE ( 'NONE', #30892, #7965 ) ;
#50318=VERTEX_POINT ( 'NONE', #13681 ) ;
#50320=CARTESIAN_POINT ( 'NONE',  ( 35.00000000000061107, 17.00000000000000000, -30.00000000000000000 ) ) ;
#50324=EDGE_CURVE ( 'NONE', #34466, #22541, #37063, .T. ) ;
#50330=PLANE ( 'NONE',  #42695 ) ;
#50341=EDGE_CURVE ( 'NONE', #343, #39269, #37564, .T. ) ;
#50344=DIRECTION ( 'NONE',  ( 1.000000000000000000, 0.000000000000000000, 0.000000000000000000 ) ) ;
#50346=ORIENTED_EDGE ( 'NONE', *, *, #39395, .T. ) ;
#50351=LINE ( 'NONE', #19353, #11362 ) ;
#50361=AXIS2_PLACEMENT_3D ( 'NONE', #43721, #8590, #47292 ) ;
#50362=DIRECTION ( 'NONE',  ( -0.000000000000000000, -1.000000000000000000, -0.000000000000000000 ) ) ;
#50364=LINE ( 'NONE', #35815, #31947 ) ;
#50375=DIRECTION ( 'NONE',  ( 0.000000000000000000, 0.000000000000000000, 1.000000000000000000 ) ) ;
#50380=ORIENTED_EDGE ( 'NONE', *, *, #50162, .F. ) ;
#50381=ORIENTED_EDGE ( 'NONE', *, *, #30641, .T. ) ;
#50387=ORIENTED_EDGE ( 'NONE', *, *, #35549, .F. ) ;
#50406=DIRECTION ( 'NONE',  ( -0.000000000000000000, 1.000000000000000000, 0.000000000000000000 ) ) ;
#50408=CARTESIAN_POINT ( 'NONE',  ( 35.00000000000091660, 16.00000000000000000, 0.000000000000000000 ) ) ;
#50410=EDGE_LOOP ( 'NONE', ( #16736, #30077, #36005, #42959 ) ) ;
#50423=LINE ( 'NONE', #31751, #13994 ) ;
#50429=CARTESIAN_POINT ( 'NONE',  ( -164.9999999999994031, 17.00000000000000000, -30.00000000000000000 ) ) ;
#50432=EDGE_CURVE ( 'NONE', #17930, #30535, #49955, .T. ) ;
#50438=VECTOR ( 'NONE', #27715, 1000.000000000000000 ) ;
#50445=LINE ( 'NONE', #42527, #35012 ) ;
#50449=CARTESIAN_POINT ( 'NONE',  ( -120.0000000000000426, 17.00000000000000000, -90.00000000000000000 ) ) ;
#50455=EDGE_LOOP ( 'NONE', ( #43180, #9616, #16406, #32695 ) ) ;
#50458=PLANE ( 'NONE',  #18482 ) ;
#50467=PLANE ( 'NONE',  #48642 ) ;
#50469=CARTESIAN_POINT ( 'NONE',  ( 130.0000000000002842, 17.00000000000000000, -84.99999999999998579 ) ) ;
#50473=DIRECTION ( 'NONE',  ( 1.000000000000000000, 0.000000000000000000, -0.000000000000000000 ) ) ;
#50477=VECTOR ( 'NONE', #48570, 1000.000000000000000 ) ;
#50480=CARTESIAN_POINT ( 'NONE',  ( -119.9999999999981668, 16.00000000000000000, 90.00000000000000000 ) ) ;
#50492=LINE ( 'NONE', #31317, #8481 ) ;
#50517=FACE_OUTER_BOUND ( 'NONE', #32073, .T. ) ;
#50522=EDGE_CURVE ( 'NONE', #23700, #28202, #15617, .T. ) ;
#50526=ORIENTED_EDGE ( 'NONE', *, *, #43751, .F. ) ;
#50530=DIRECTION ( 'NONE',  ( -0.000000000000000000, -1.000000000000000000, -0.000000000000000000 ) ) ;
#50536=EDGE_CURVE ( 'NONE', #46762, #20108, #11522, .T. ) ;
#50543=AXIS2_PLACEMENT_3D ( 'NONE', #33251, #25527, #29627 ) ;
#50554=ORIENTED_EDGE ( 'NONE', *, *, #6400, .T. ) ;
#50558=LINE ( 'NONE', #30608, #41790 ) ;
#50559=VERTEX_POINT ( 'NONE', #25036 ) ;
#50560=LINE ( 'NONE', #12361, #4987 ) ;
#50570=VERTEX_POINT ( 'NONE', #13468 ) ;
#50589=EDGE_CURVE ( 'NONE', #15045, #29675, #40683, .T. ) ;
#50591=ORIENTED_EDGE ( 'NONE', *, *, #23993, .T. ) ;
#50592=CARTESIAN_POINT ( 'NONE',  ( -64.99999999999815259, 17.00000000000000000, 90.00000000000000000 ) ) ;
#50595=DIRECTION ( 'NONE',  ( 0.000000000000000000, 0.000000000000000000, -1.000000000000000000 ) ) ;
#50604=CARTESIAN_POINT ( 'NONE',  ( 0.000000000000000000, 17.00000000000000000, 0.000000000000000000 ) ) ;
#50610=CARTESIAN_POINT ( 'NONE',  ( -69.99999999999816680, 16.00000000000000000, 90.00000000000000000 ) ) ;
#50631=LINE ( 'NONE', #46283, #4305 ) ;
#50635=VERTEX_POINT ( 'NONE', #2429 ) ;
#50637=EDGE_LOOP ( 'NONE', ( #32099, #16535, #18977, #26767 ) ) ;
#50651=EDGE_LOOP ( 'NONE', ( #8422, #10148, #2041, #48933 ) ) ;
#50652=ORIENTED_EDGE ( 'NONE', *, *, #29760, .T. ) ;
#50660=VECTOR ( 'NONE', #7443, 1000.000000000000000 ) ;
#50663=ADVANCED_FACE ( 'NONE', ( #29879 ), #38100, .F. ) ;
#50664=CARTESIAN_POINT ( 'NONE',  ( 30.00000000000062172, 17.00000000000000000, -30.00000000000000000 ) ) ;
#50673=ORIENTED_EDGE ( 'NONE', *, *, #48359, .T. ) ;
#50692=ADVANCED_FACE ( 'NONE', ( #50078 ), #14989, .F. ) ;
#50698=VECTOR ( 'NONE', #21527, 1000.000000000000000 ) ;
#50703=ORIENTED_EDGE ( 'NONE', *, *, #30990, .F. ) ;
#50712=ORIENTED_EDGE ( 'NONE', *, *, #21249, .T. ) ;
#50719=DIRECTION ( 'NONE',  ( -0.000000000000000000, -0.000000000000000000, -1.000000000000000000 ) ) ;
#50748=COLOUR_RGB('Light Blue',0.38,0.62,0.78);
#50749=FILL_AREA_STYLE_COLOUR('',#50748);
#50750=FILL_AREA_STYLE('',(#50749));
#50751=SURFACE_STYLE_FILL_AREA(#50750);
#50752=SURFACE_SIDE_STYLE('',(#50751));
#50753=SURFACE_STYLE_USAGE(.BOTH.,#50752);
#50754=PRESENTATION_STYLE_ASSIGNMENT((#50753));
ENDSEC;
END-ISO-10303-21;
